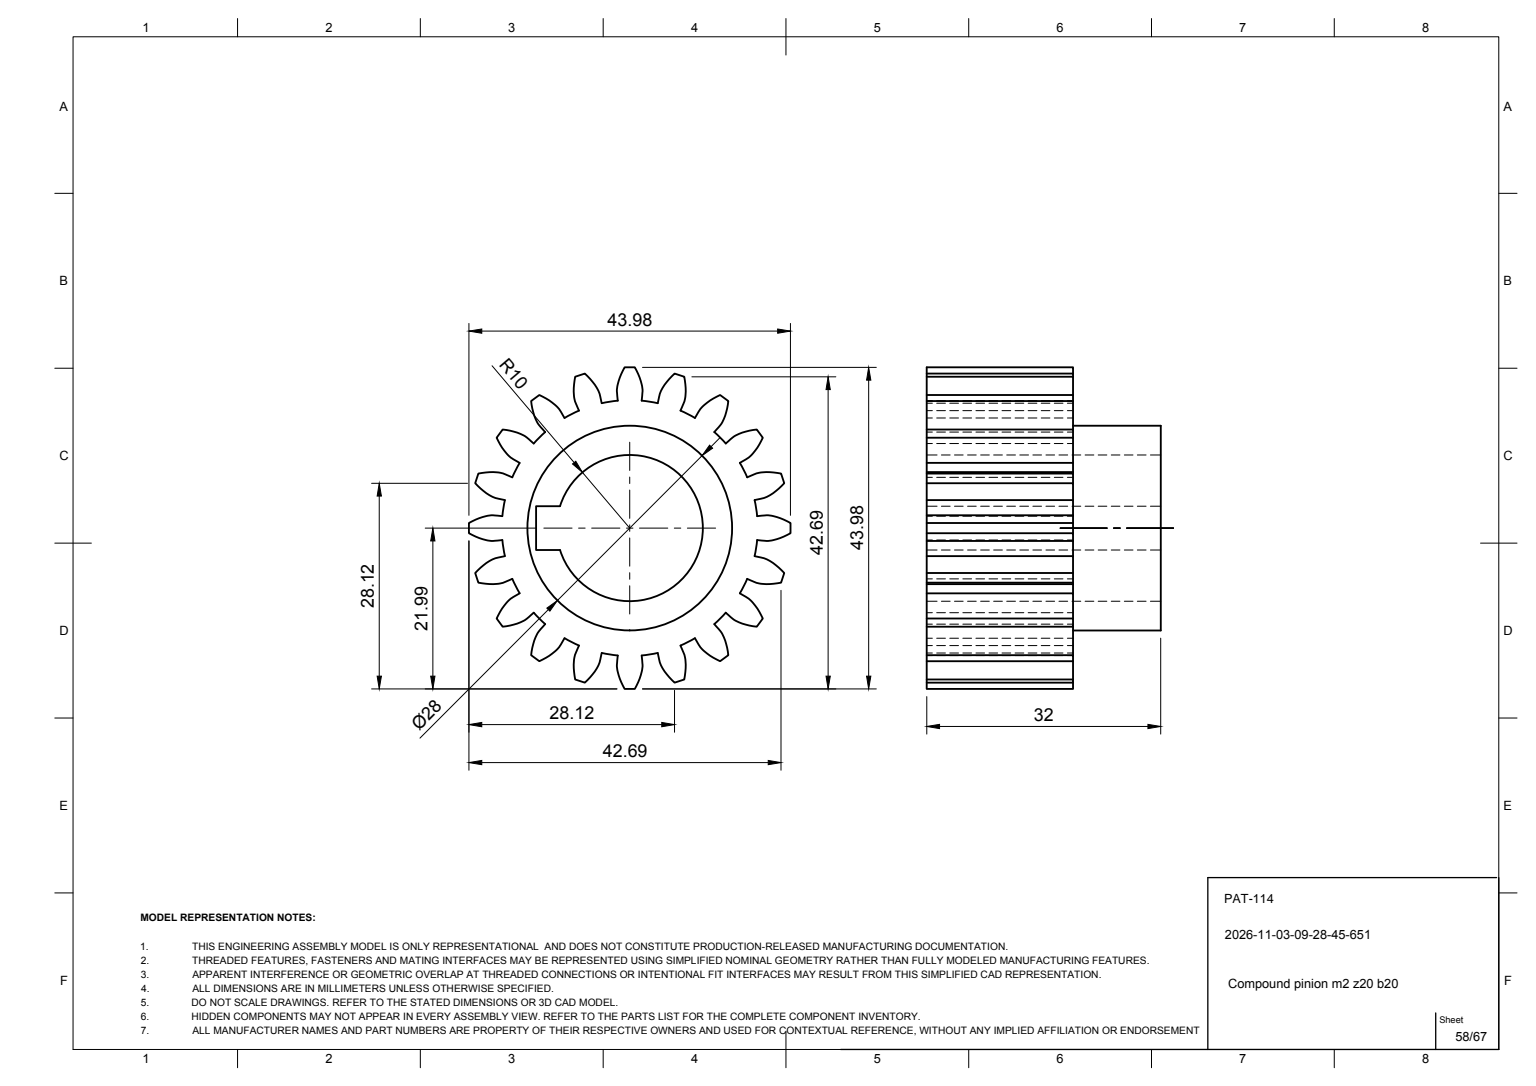
ISO-10303-21;
HEADER;
/* Generated by software containing ST-Developer
 * from STEP Tools, Inc. (www.steptools.com) 
 */

FILE_DESCRIPTION(
/* description */ ('Two-stage gear reducer in split housing'),
/* implementation_level */ '2;1');

FILE_NAME(
/* name */ 'Compound pinion m2 z20 b20.step',
/* time_stamp */ '2026-10-28T03:22:31-07:00',
/* author */ (''),
/* organization */ (''),
/* preprocessor_version */ 'ST-DEVELOPER v20.2',
/* originating_system */ 'Autodesk Translation Framework v15.17.0.0',
/* authorisation */ '');

FILE_SCHEMA (('AUTOMOTIVE_DESIGN { 1 0 10303 214 3 1 1 }'));
ENDSEC;

DATA;
#10=MECHANICAL_DESIGN_GEOMETRIC_PRESENTATION_REPRESENTATION('',(#1294),#73366);
#51=(
BOUNDED_SURFACE()
B_SPLINE_SURFACE(5,1,((#40614,#40615),(#40616,#40617),(#40618,#40619),(#40620,
#40621),(#40622,#40623),(#40624,#40625),(#40626,#40627),(#40628,#40629),
(#40630,#40631),(#40632,#40633),(#40634,#40635),(#40636,#40637),(#40638,
#40639),(#40640,#40641),(#40642,#40643),(#40644,#40645),(#40646,#40647),
(#40648,#40649),(#40650,#40651),(#40652,#40653),(#40654,#40655),(#40656,
#40657),(#40658,#40659),(#40660,#40661),(#40662,#40663),(#40664,#40665),
(#40666,#40667),(#40668,#40669),(#40670,#40671),(#40672,#40673),(#40674,
#40675),(#40676,#40677),(#40678,#40679),(#40680,#40681),(#40682,#40683),
(#40684,#40685),(#40686,#40687),(#40688,#40689),(#40690,#40691),(#40692,
#40693),(#40694,#40695),(#40696,#40697),(#40698,#40699),(#40700,#40701),
(#40702,#40703),(#40704,#40705),(#40706,#40707),(#40708,#40709),(#40710,
#40711),(#40712,#40713),(#40714,#40715),(#40716,#40717),(#40718,#40719),
(#40720,#40721),(#40722,#40723),(#40724,#40725),(#40726,#40727),(#40728,
#40729),(#40730,#40731),(#40732,#40733),(#40734,#40735),(#40736,#40737),
(#40738,#40739),(#40740,#40741),(#40742,#40743),(#40744,#40745),(#40746,
#40747),(#40748,#40749),(#40750,#40751),(#40752,#40753)),.UNSPECIFIED.,
 .F.,.F.,.F.)
B_SPLINE_SURFACE_WITH_KNOTS((6,1,1,1,1,1,1,1,1,1,1,1,1,1,1,1,1,1,1,1,1,
1,1,1,1,1,1,1,1,1,1,1,1,1,1,1,1,1,1,1,1,1,1,1,1,1,1,1,1,1,1,1,1,1,1,1,1,
1,1,1,1,1,1,1,1,6),(2,2),(-1.,-0.984615384615383,-0.969230769230768,-0.953846153846152,
-0.938461538461537,-0.923076923076922,-0.907692307692306,-0.892307692307691,
-0.876923076923076,-0.86153846153846,-0.846153846153845,-0.83076923076923,
-0.815384615384614,-0.799999999999999,-0.784615384615384,-0.769230769230768,
-0.753846153846153,-0.738461538461538,-0.723076923076922,-0.707692307692307,
-0.692307692307692,-0.676923076923076,-0.661538461538461,-0.646153846153846,
-0.63076923076923,-0.615384615384615,-0.6,-0.584615384615384,-0.569230769230769,
-0.553846153846154,-0.538461538461538,-0.523076923076923,-0.507692307692308,
-0.492307692307692,-0.476923076923077,-0.461538461538462,-0.446153846153846,
-0.430769230769231,-0.415384615384615,-0.4,-0.384615384615385,-0.369230769230769,
-0.353846153846154,-0.338461538461538,-0.323076923076923,-0.307692307692308,
-0.292307692307692,-0.276923076923077,-0.261538461538462,-0.246153846153846,
-0.230769230769231,-0.215384615384615,-0.2,-0.184615384615385,-0.169230769230769,
-0.153846153846154,-0.138461538461538,-0.123076923076923,-0.107692307692308,
-0.0923076923076923,-0.0769230769230769,-0.0615384615384615,-0.0461538461538462,
-0.0307692307692308,-0.0153846153846154,0.),(-1.,1.),.UNSPECIFIED.)
GEOMETRIC_REPRESENTATION_ITEM()
RATIONAL_B_SPLINE_SURFACE(((1.,1.),(1.,1.),(1.,1.),(1.,1.),(1.,1.),(1.,
1.),(1.,1.),(1.,1.),(1.,1.),(1.,1.),(1.,1.),(1.,1.),(1.,1.),(1.,1.),(1.,
1.),(1.,1.),(1.,1.),(1.,1.),(1.,1.),(1.,1.),(1.,1.),(1.,1.),(1.,1.),(1.,
1.),(1.,1.),(1.,1.),(1.,1.),(1.,1.),(1.,1.),(1.,1.),(1.,1.),(1.,1.),(1.,
1.),(1.,1.),(1.,1.),(1.,1.),(1.,1.),(1.,1.),(1.,1.),(1.,1.),(1.,1.),(1.,
1.),(1.,1.),(1.,1.),(1.,1.),(1.,1.),(1.,1.),(1.,1.),(1.,1.),(1.,1.),(1.,
1.),(1.,1.),(1.,1.),(1.,1.),(1.,1.),(1.,1.),(1.,1.),(1.,1.),(1.,1.),(1.,
1.),(1.,1.),(1.,1.),(1.,1.),(1.,1.),(1.,1.),(1.,1.),(1.,1.),(1.,1.),(1.,
1.),(1.,1.)))
REPRESENTATION_ITEM('')
SURFACE()
);
#52=(
BOUNDED_SURFACE()
B_SPLINE_SURFACE(5,1,((#40832,#40833),(#40834,#40835),(#40836,#40837),(#40838,
#40839),(#40840,#40841),(#40842,#40843),(#40844,#40845),(#40846,#40847),
(#40848,#40849),(#40850,#40851),(#40852,#40853),(#40854,#40855),(#40856,
#40857),(#40858,#40859),(#40860,#40861),(#40862,#40863),(#40864,#40865),
(#40866,#40867),(#40868,#40869),(#40870,#40871),(#40872,#40873),(#40874,
#40875),(#40876,#40877),(#40878,#40879),(#40880,#40881),(#40882,#40883),
(#40884,#40885),(#40886,#40887),(#40888,#40889),(#40890,#40891),(#40892,
#40893),(#40894,#40895),(#40896,#40897),(#40898,#40899),(#40900,#40901),
(#40902,#40903),(#40904,#40905),(#40906,#40907),(#40908,#40909),(#40910,
#40911),(#40912,#40913),(#40914,#40915),(#40916,#40917),(#40918,#40919),
(#40920,#40921),(#40922,#40923),(#40924,#40925),(#40926,#40927),(#40928,
#40929),(#40930,#40931),(#40932,#40933),(#40934,#40935),(#40936,#40937),
(#40938,#40939),(#40940,#40941),(#40942,#40943),(#40944,#40945),(#40946,
#40947),(#40948,#40949),(#40950,#40951),(#40952,#40953),(#40954,#40955),
(#40956,#40957),(#40958,#40959),(#40960,#40961),(#40962,#40963),(#40964,
#40965),(#40966,#40967),(#40968,#40969),(#40970,#40971)),.UNSPECIFIED.,
 .F.,.F.,.F.)
B_SPLINE_SURFACE_WITH_KNOTS((6,1,1,1,1,1,1,1,1,1,1,1,1,1,1,1,1,1,1,1,1,
1,1,1,1,1,1,1,1,1,1,1,1,1,1,1,1,1,1,1,1,1,1,1,1,1,1,1,1,1,1,1,1,1,1,1,1,
1,1,1,1,1,1,1,1,6),(2,2),(-1.,-0.984615384615383,-0.969230769230768,-0.953846153846152,
-0.938461538461537,-0.923076923076922,-0.907692307692306,-0.892307692307691,
-0.876923076923076,-0.86153846153846,-0.846153846153845,-0.83076923076923,
-0.815384615384614,-0.799999999999999,-0.784615384615384,-0.769230769230768,
-0.753846153846153,-0.738461538461538,-0.723076923076922,-0.707692307692307,
-0.692307692307692,-0.676923076923076,-0.661538461538461,-0.646153846153846,
-0.63076923076923,-0.615384615384615,-0.6,-0.584615384615384,-0.569230769230769,
-0.553846153846154,-0.538461538461538,-0.523076923076923,-0.507692307692308,
-0.492307692307692,-0.476923076923077,-0.461538461538462,-0.446153846153846,
-0.430769230769231,-0.415384615384615,-0.4,-0.384615384615385,-0.369230769230769,
-0.353846153846154,-0.338461538461538,-0.323076923076923,-0.307692307692308,
-0.292307692307692,-0.276923076923077,-0.261538461538462,-0.246153846153846,
-0.230769230769231,-0.215384615384615,-0.2,-0.184615384615385,-0.169230769230769,
-0.153846153846154,-0.138461538461538,-0.123076923076923,-0.107692307692308,
-0.0923076923076923,-0.0769230769230769,-0.0615384615384615,-0.0461538461538462,
-0.0307692307692308,-0.0153846153846154,0.),(-1.,1.),.UNSPECIFIED.)
GEOMETRIC_REPRESENTATION_ITEM()
RATIONAL_B_SPLINE_SURFACE(((1.,1.),(1.,1.),(1.,1.),(1.,1.),(1.,1.),(1.,
1.),(1.,1.),(1.,1.),(1.,1.),(1.,1.),(1.,1.),(1.,1.),(1.,1.),(1.,1.),(1.,
1.),(1.,1.),(1.,1.),(1.,1.),(1.,1.),(1.,1.),(1.,1.),(1.,1.),(1.,1.),(1.,
1.),(1.,1.),(1.,1.),(1.,1.),(1.,1.),(1.,1.),(1.,1.),(1.,1.),(1.,1.),(1.,
1.),(1.,1.),(1.,1.),(1.,1.),(1.,1.),(1.,1.),(1.,1.),(1.,1.),(1.,1.),(1.,
1.),(1.,1.),(1.,1.),(1.,1.),(1.,1.),(1.,1.),(1.,1.),(1.,1.),(1.,1.),(1.,
1.),(1.,1.),(1.,1.),(1.,1.),(1.,1.),(1.,1.),(1.,1.),(1.,1.),(1.,1.),(1.,
1.),(1.,1.),(1.,1.),(1.,1.),(1.,1.),(1.,1.),(1.,1.),(1.,1.),(1.,1.),(1.,
1.),(1.,1.)))
REPRESENTATION_ITEM('')
SURFACE()
);
#53=(
BOUNDED_SURFACE()
B_SPLINE_SURFACE(5,1,((#41048,#41049),(#41050,#41051),(#41052,#41053),(#41054,
#41055),(#41056,#41057),(#41058,#41059),(#41060,#41061),(#41062,#41063),
(#41064,#41065),(#41066,#41067),(#41068,#41069),(#41070,#41071),(#41072,
#41073),(#41074,#41075),(#41076,#41077),(#41078,#41079),(#41080,#41081),
(#41082,#41083),(#41084,#41085),(#41086,#41087),(#41088,#41089),(#41090,
#41091),(#41092,#41093),(#41094,#41095),(#41096,#41097),(#41098,#41099),
(#41100,#41101),(#41102,#41103),(#41104,#41105),(#41106,#41107),(#41108,
#41109),(#41110,#41111),(#41112,#41113),(#41114,#41115),(#41116,#41117),
(#41118,#41119),(#41120,#41121),(#41122,#41123),(#41124,#41125),(#41126,
#41127),(#41128,#41129),(#41130,#41131),(#41132,#41133),(#41134,#41135),
(#41136,#41137),(#41138,#41139),(#41140,#41141),(#41142,#41143),(#41144,
#41145),(#41146,#41147),(#41148,#41149),(#41150,#41151),(#41152,#41153),
(#41154,#41155),(#41156,#41157),(#41158,#41159),(#41160,#41161),(#41162,
#41163),(#41164,#41165),(#41166,#41167),(#41168,#41169),(#41170,#41171),
(#41172,#41173),(#41174,#41175),(#41176,#41177),(#41178,#41179),(#41180,
#41181),(#41182,#41183),(#41184,#41185),(#41186,#41187)),.UNSPECIFIED.,
 .F.,.F.,.F.)
B_SPLINE_SURFACE_WITH_KNOTS((6,1,1,1,1,1,1,1,1,1,1,1,1,1,1,1,1,1,1,1,1,
1,1,1,1,1,1,1,1,1,1,1,1,1,1,1,1,1,1,1,1,1,1,1,1,1,1,1,1,1,1,1,1,1,1,1,1,
1,1,1,1,1,1,1,1,6),(2,2),(-1.,-0.984615384615383,-0.969230769230768,-0.953846153846152,
-0.938461538461537,-0.923076923076922,-0.907692307692306,-0.892307692307691,
-0.876923076923076,-0.86153846153846,-0.846153846153845,-0.83076923076923,
-0.815384615384614,-0.799999999999999,-0.784615384615384,-0.769230769230768,
-0.753846153846153,-0.738461538461538,-0.723076923076922,-0.707692307692307,
-0.692307692307692,-0.676923076923076,-0.661538461538461,-0.646153846153846,
-0.63076923076923,-0.615384615384615,-0.6,-0.584615384615384,-0.569230769230769,
-0.553846153846154,-0.538461538461538,-0.523076923076923,-0.507692307692308,
-0.492307692307692,-0.476923076923077,-0.461538461538462,-0.446153846153846,
-0.430769230769231,-0.415384615384615,-0.4,-0.384615384615385,-0.369230769230769,
-0.353846153846154,-0.338461538461538,-0.323076923076923,-0.307692307692308,
-0.292307692307692,-0.276923076923077,-0.261538461538462,-0.246153846153846,
-0.230769230769231,-0.215384615384615,-0.2,-0.184615384615385,-0.169230769230769,
-0.153846153846154,-0.138461538461538,-0.123076923076923,-0.107692307692308,
-0.0923076923076923,-0.0769230769230769,-0.0615384615384615,-0.0461538461538462,
-0.0307692307692308,-0.0153846153846154,0.),(-1.,1.),.UNSPECIFIED.)
GEOMETRIC_REPRESENTATION_ITEM()
RATIONAL_B_SPLINE_SURFACE(((1.,1.),(1.,1.),(1.,1.),(1.,1.),(1.,1.),(1.,
1.),(1.,1.),(1.,1.),(1.,1.),(1.,1.),(1.,1.),(1.,1.),(1.,1.),(1.,1.),(1.,
1.),(1.,1.),(1.,1.),(1.,1.),(1.,1.),(1.,1.),(1.,1.),(1.,1.),(1.,1.),(1.,
1.),(1.,1.),(1.,1.),(1.,1.),(1.,1.),(1.,1.),(1.,1.),(1.,1.),(1.,1.),(1.,
1.),(1.,1.),(1.,1.),(1.,1.),(1.,1.),(1.,1.),(1.,1.),(1.,1.),(1.,1.),(1.,
1.),(1.,1.),(1.,1.),(1.,1.),(1.,1.),(1.,1.),(1.,1.),(1.,1.),(1.,1.),(1.,
1.),(1.,1.),(1.,1.),(1.,1.),(1.,1.),(1.,1.),(1.,1.),(1.,1.),(1.,1.),(1.,
1.),(1.,1.),(1.,1.),(1.,1.),(1.,1.),(1.,1.),(1.,1.),(1.,1.),(1.,1.),(1.,
1.),(1.,1.)))
REPRESENTATION_ITEM('')
SURFACE()
);
#54=(
BOUNDED_SURFACE()
B_SPLINE_SURFACE(5,1,((#41264,#41265),(#41266,#41267),(#41268,#41269),(#41270,
#41271),(#41272,#41273),(#41274,#41275),(#41276,#41277),(#41278,#41279),
(#41280,#41281),(#41282,#41283),(#41284,#41285),(#41286,#41287),(#41288,
#41289),(#41290,#41291),(#41292,#41293),(#41294,#41295),(#41296,#41297),
(#41298,#41299),(#41300,#41301),(#41302,#41303),(#41304,#41305),(#41306,
#41307),(#41308,#41309),(#41310,#41311),(#41312,#41313),(#41314,#41315),
(#41316,#41317),(#41318,#41319),(#41320,#41321),(#41322,#41323),(#41324,
#41325),(#41326,#41327),(#41328,#41329),(#41330,#41331),(#41332,#41333),
(#41334,#41335),(#41336,#41337),(#41338,#41339),(#41340,#41341),(#41342,
#41343),(#41344,#41345),(#41346,#41347),(#41348,#41349),(#41350,#41351),
(#41352,#41353),(#41354,#41355),(#41356,#41357),(#41358,#41359),(#41360,
#41361),(#41362,#41363),(#41364,#41365),(#41366,#41367),(#41368,#41369),
(#41370,#41371),(#41372,#41373),(#41374,#41375),(#41376,#41377),(#41378,
#41379),(#41380,#41381),(#41382,#41383),(#41384,#41385),(#41386,#41387),
(#41388,#41389),(#41390,#41391),(#41392,#41393),(#41394,#41395),(#41396,
#41397),(#41398,#41399),(#41400,#41401),(#41402,#41403)),.UNSPECIFIED.,
 .F.,.F.,.F.)
B_SPLINE_SURFACE_WITH_KNOTS((6,1,1,1,1,1,1,1,1,1,1,1,1,1,1,1,1,1,1,1,1,
1,1,1,1,1,1,1,1,1,1,1,1,1,1,1,1,1,1,1,1,1,1,1,1,1,1,1,1,1,1,1,1,1,1,1,1,
1,1,1,1,1,1,1,1,6),(2,2),(-1.,-0.984615384615383,-0.969230769230768,-0.953846153846152,
-0.938461538461537,-0.923076923076922,-0.907692307692306,-0.892307692307691,
-0.876923076923076,-0.86153846153846,-0.846153846153845,-0.83076923076923,
-0.815384615384614,-0.799999999999999,-0.784615384615384,-0.769230769230768,
-0.753846153846153,-0.738461538461538,-0.723076923076922,-0.707692307692307,
-0.692307692307692,-0.676923076923076,-0.661538461538461,-0.646153846153846,
-0.63076923076923,-0.615384615384615,-0.6,-0.584615384615384,-0.569230769230769,
-0.553846153846154,-0.538461538461538,-0.523076923076923,-0.507692307692308,
-0.492307692307692,-0.476923076923077,-0.461538461538462,-0.446153846153846,
-0.430769230769231,-0.415384615384615,-0.4,-0.384615384615385,-0.369230769230769,
-0.353846153846154,-0.338461538461538,-0.323076923076923,-0.307692307692308,
-0.292307692307692,-0.276923076923077,-0.261538461538462,-0.246153846153846,
-0.230769230769231,-0.215384615384615,-0.2,-0.184615384615385,-0.169230769230769,
-0.153846153846154,-0.138461538461538,-0.123076923076923,-0.107692307692308,
-0.0923076923076923,-0.0769230769230769,-0.0615384615384615,-0.0461538461538462,
-0.0307692307692308,-0.0153846153846154,0.),(-1.,1.),.UNSPECIFIED.)
GEOMETRIC_REPRESENTATION_ITEM()
RATIONAL_B_SPLINE_SURFACE(((1.,1.),(1.,1.),(1.,1.),(1.,1.),(1.,1.),(1.,
1.),(1.,1.),(1.,1.),(1.,1.),(1.,1.),(1.,1.),(1.,1.),(1.,1.),(1.,1.),(1.,
1.),(1.,1.),(1.,1.),(1.,1.),(1.,1.),(1.,1.),(1.,1.),(1.,1.),(1.,1.),(1.,
1.),(1.,1.),(1.,1.),(1.,1.),(1.,1.),(1.,1.),(1.,1.),(1.,1.),(1.,1.),(1.,
1.),(1.,1.),(1.,1.),(1.,1.),(1.,1.),(1.,1.),(1.,1.),(1.,1.),(1.,1.),(1.,
1.),(1.,1.),(1.,1.),(1.,1.),(1.,1.),(1.,1.),(1.,1.),(1.,1.),(1.,1.),(1.,
1.),(1.,1.),(1.,1.),(1.,1.),(1.,1.),(1.,1.),(1.,1.),(1.,1.),(1.,1.),(1.,
1.),(1.,1.),(1.,1.),(1.,1.),(1.,1.),(1.,1.),(1.,1.),(1.,1.),(1.,1.),(1.,
1.),(1.,1.)))
REPRESENTATION_ITEM('')
SURFACE()
);
#55=(
BOUNDED_SURFACE()
B_SPLINE_SURFACE(5,1,((#41480,#41481),(#41482,#41483),(#41484,#41485),(#41486,
#41487),(#41488,#41489),(#41490,#41491),(#41492,#41493),(#41494,#41495),
(#41496,#41497),(#41498,#41499),(#41500,#41501),(#41502,#41503),(#41504,
#41505),(#41506,#41507),(#41508,#41509),(#41510,#41511),(#41512,#41513),
(#41514,#41515),(#41516,#41517),(#41518,#41519),(#41520,#41521),(#41522,
#41523),(#41524,#41525),(#41526,#41527),(#41528,#41529),(#41530,#41531),
(#41532,#41533),(#41534,#41535),(#41536,#41537),(#41538,#41539),(#41540,
#41541),(#41542,#41543),(#41544,#41545),(#41546,#41547),(#41548,#41549),
(#41550,#41551),(#41552,#41553),(#41554,#41555),(#41556,#41557),(#41558,
#41559),(#41560,#41561),(#41562,#41563),(#41564,#41565),(#41566,#41567),
(#41568,#41569),(#41570,#41571),(#41572,#41573),(#41574,#41575),(#41576,
#41577),(#41578,#41579),(#41580,#41581),(#41582,#41583),(#41584,#41585),
(#41586,#41587),(#41588,#41589),(#41590,#41591),(#41592,#41593),(#41594,
#41595),(#41596,#41597),(#41598,#41599),(#41600,#41601),(#41602,#41603),
(#41604,#41605),(#41606,#41607),(#41608,#41609),(#41610,#41611),(#41612,
#41613),(#41614,#41615),(#41616,#41617),(#41618,#41619)),.UNSPECIFIED.,
 .F.,.F.,.F.)
B_SPLINE_SURFACE_WITH_KNOTS((6,1,1,1,1,1,1,1,1,1,1,1,1,1,1,1,1,1,1,1,1,
1,1,1,1,1,1,1,1,1,1,1,1,1,1,1,1,1,1,1,1,1,1,1,1,1,1,1,1,1,1,1,1,1,1,1,1,
1,1,1,1,1,1,1,1,6),(2,2),(-1.,-0.984615384615383,-0.969230769230768,-0.953846153846152,
-0.938461538461537,-0.923076923076922,-0.907692307692306,-0.892307692307691,
-0.876923076923076,-0.86153846153846,-0.846153846153845,-0.83076923076923,
-0.815384615384614,-0.799999999999999,-0.784615384615384,-0.769230769230768,
-0.753846153846153,-0.738461538461538,-0.723076923076922,-0.707692307692307,
-0.692307692307692,-0.676923076923076,-0.661538461538461,-0.646153846153846,
-0.63076923076923,-0.615384615384615,-0.6,-0.584615384615384,-0.569230769230769,
-0.553846153846154,-0.538461538461538,-0.523076923076923,-0.507692307692308,
-0.492307692307692,-0.476923076923077,-0.461538461538462,-0.446153846153846,
-0.430769230769231,-0.415384615384615,-0.4,-0.384615384615385,-0.369230769230769,
-0.353846153846154,-0.338461538461538,-0.323076923076923,-0.307692307692308,
-0.292307692307692,-0.276923076923077,-0.261538461538462,-0.246153846153846,
-0.230769230769231,-0.215384615384615,-0.2,-0.184615384615385,-0.169230769230769,
-0.153846153846154,-0.138461538461538,-0.123076923076923,-0.107692307692308,
-0.0923076923076923,-0.0769230769230769,-0.0615384615384615,-0.0461538461538462,
-0.0307692307692308,-0.0153846153846154,0.),(-1.,1.),.UNSPECIFIED.)
GEOMETRIC_REPRESENTATION_ITEM()
RATIONAL_B_SPLINE_SURFACE(((1.,1.),(1.,1.),(1.,1.),(1.,1.),(1.,1.),(1.,
1.),(1.,1.),(1.,1.),(1.,1.),(1.,1.),(1.,1.),(1.,1.),(1.,1.),(1.,1.),(1.,
1.),(1.,1.),(1.,1.),(1.,1.),(1.,1.),(1.,1.),(1.,1.),(1.,1.),(1.,1.),(1.,
1.),(1.,1.),(1.,1.),(1.,1.),(1.,1.),(1.,1.),(1.,1.),(1.,1.),(1.,1.),(1.,
1.),(1.,1.),(1.,1.),(1.,1.),(1.,1.),(1.,1.),(1.,1.),(1.,1.),(1.,1.),(1.,
1.),(1.,1.),(1.,1.),(1.,1.),(1.,1.),(1.,1.),(1.,1.),(1.,1.),(1.,1.),(1.,
1.),(1.,1.),(1.,1.),(1.,1.),(1.,1.),(1.,1.),(1.,1.),(1.,1.),(1.,1.),(1.,
1.),(1.,1.),(1.,1.),(1.,1.),(1.,1.),(1.,1.),(1.,1.),(1.,1.),(1.,1.),(1.,
1.),(1.,1.)))
REPRESENTATION_ITEM('')
SURFACE()
);
#56=(
BOUNDED_SURFACE()
B_SPLINE_SURFACE(5,1,((#41696,#41697),(#41698,#41699),(#41700,#41701),(#41702,
#41703),(#41704,#41705),(#41706,#41707),(#41708,#41709),(#41710,#41711),
(#41712,#41713),(#41714,#41715),(#41716,#41717),(#41718,#41719),(#41720,
#41721),(#41722,#41723),(#41724,#41725),(#41726,#41727),(#41728,#41729),
(#41730,#41731),(#41732,#41733),(#41734,#41735),(#41736,#41737),(#41738,
#41739),(#41740,#41741),(#41742,#41743),(#41744,#41745),(#41746,#41747),
(#41748,#41749),(#41750,#41751),(#41752,#41753),(#41754,#41755),(#41756,
#41757),(#41758,#41759),(#41760,#41761),(#41762,#41763),(#41764,#41765),
(#41766,#41767),(#41768,#41769),(#41770,#41771),(#41772,#41773),(#41774,
#41775),(#41776,#41777),(#41778,#41779),(#41780,#41781),(#41782,#41783),
(#41784,#41785),(#41786,#41787),(#41788,#41789),(#41790,#41791),(#41792,
#41793),(#41794,#41795),(#41796,#41797),(#41798,#41799),(#41800,#41801),
(#41802,#41803),(#41804,#41805),(#41806,#41807),(#41808,#41809),(#41810,
#41811),(#41812,#41813),(#41814,#41815),(#41816,#41817),(#41818,#41819),
(#41820,#41821),(#41822,#41823),(#41824,#41825),(#41826,#41827),(#41828,
#41829),(#41830,#41831),(#41832,#41833),(#41834,#41835)),.UNSPECIFIED.,
 .F.,.F.,.F.)
B_SPLINE_SURFACE_WITH_KNOTS((6,1,1,1,1,1,1,1,1,1,1,1,1,1,1,1,1,1,1,1,1,
1,1,1,1,1,1,1,1,1,1,1,1,1,1,1,1,1,1,1,1,1,1,1,1,1,1,1,1,1,1,1,1,1,1,1,1,
1,1,1,1,1,1,1,1,6),(2,2),(-1.,-0.984615384615383,-0.969230769230768,-0.953846153846152,
-0.938461538461537,-0.923076923076922,-0.907692307692306,-0.892307692307691,
-0.876923076923076,-0.86153846153846,-0.846153846153845,-0.83076923076923,
-0.815384615384614,-0.799999999999999,-0.784615384615384,-0.769230769230768,
-0.753846153846153,-0.738461538461538,-0.723076923076922,-0.707692307692307,
-0.692307692307692,-0.676923076923076,-0.661538461538461,-0.646153846153846,
-0.63076923076923,-0.615384615384615,-0.6,-0.584615384615384,-0.569230769230769,
-0.553846153846154,-0.538461538461538,-0.523076923076923,-0.507692307692308,
-0.492307692307692,-0.476923076923077,-0.461538461538462,-0.446153846153846,
-0.430769230769231,-0.415384615384615,-0.4,-0.384615384615385,-0.369230769230769,
-0.353846153846154,-0.338461538461538,-0.323076923076923,-0.307692307692308,
-0.292307692307692,-0.276923076923077,-0.261538461538462,-0.246153846153846,
-0.230769230769231,-0.215384615384615,-0.2,-0.184615384615385,-0.169230769230769,
-0.153846153846154,-0.138461538461538,-0.123076923076923,-0.107692307692308,
-0.0923076923076923,-0.0769230769230769,-0.0615384615384615,-0.0461538461538462,
-0.0307692307692308,-0.0153846153846154,0.),(-1.,1.),.UNSPECIFIED.)
GEOMETRIC_REPRESENTATION_ITEM()
RATIONAL_B_SPLINE_SURFACE(((1.,1.),(1.,1.),(1.,1.),(1.,1.),(1.,1.),(1.,
1.),(1.,1.),(1.,1.),(1.,1.),(1.,1.),(1.,1.),(1.,1.),(1.,1.),(1.,1.),(1.,
1.),(1.,1.),(1.,1.),(1.,1.),(1.,1.),(1.,1.),(1.,1.),(1.,1.),(1.,1.),(1.,
1.),(1.,1.),(1.,1.),(1.,1.),(1.,1.),(1.,1.),(1.,1.),(1.,1.),(1.,1.),(1.,
1.),(1.,1.),(1.,1.),(1.,1.),(1.,1.),(1.,1.),(1.,1.),(1.,1.),(1.,1.),(1.,
1.),(1.,1.),(1.,1.),(1.,1.),(1.,1.),(1.,1.),(1.,1.),(1.,1.),(1.,1.),(1.,
1.),(1.,1.),(1.,1.),(1.,1.),(1.,1.),(1.,1.),(1.,1.),(1.,1.),(1.,1.),(1.,
1.),(1.,1.),(1.,1.),(1.,1.),(1.,1.),(1.,1.),(1.,1.),(1.,1.),(1.,1.),(1.,
1.),(1.,1.)))
REPRESENTATION_ITEM('')
SURFACE()
);
#57=(
BOUNDED_SURFACE()
B_SPLINE_SURFACE(5,1,((#41912,#41913),(#41914,#41915),(#41916,#41917),(#41918,
#41919),(#41920,#41921),(#41922,#41923),(#41924,#41925),(#41926,#41927),
(#41928,#41929),(#41930,#41931),(#41932,#41933),(#41934,#41935),(#41936,
#41937),(#41938,#41939),(#41940,#41941),(#41942,#41943),(#41944,#41945),
(#41946,#41947),(#41948,#41949),(#41950,#41951),(#41952,#41953),(#41954,
#41955),(#41956,#41957),(#41958,#41959),(#41960,#41961),(#41962,#41963),
(#41964,#41965),(#41966,#41967),(#41968,#41969),(#41970,#41971),(#41972,
#41973),(#41974,#41975),(#41976,#41977),(#41978,#41979),(#41980,#41981),
(#41982,#41983),(#41984,#41985),(#41986,#41987),(#41988,#41989),(#41990,
#41991),(#41992,#41993),(#41994,#41995),(#41996,#41997),(#41998,#41999),
(#42000,#42001),(#42002,#42003),(#42004,#42005),(#42006,#42007),(#42008,
#42009),(#42010,#42011),(#42012,#42013),(#42014,#42015),(#42016,#42017),
(#42018,#42019),(#42020,#42021),(#42022,#42023),(#42024,#42025),(#42026,
#42027),(#42028,#42029),(#42030,#42031),(#42032,#42033),(#42034,#42035),
(#42036,#42037),(#42038,#42039),(#42040,#42041),(#42042,#42043),(#42044,
#42045),(#42046,#42047),(#42048,#42049),(#42050,#42051)),.UNSPECIFIED.,
 .F.,.F.,.F.)
B_SPLINE_SURFACE_WITH_KNOTS((6,1,1,1,1,1,1,1,1,1,1,1,1,1,1,1,1,1,1,1,1,
1,1,1,1,1,1,1,1,1,1,1,1,1,1,1,1,1,1,1,1,1,1,1,1,1,1,1,1,1,1,1,1,1,1,1,1,
1,1,1,1,1,1,1,1,6),(2,2),(-1.,-0.984615384615383,-0.969230769230768,-0.953846153846152,
-0.938461538461537,-0.923076923076922,-0.907692307692306,-0.892307692307691,
-0.876923076923076,-0.86153846153846,-0.846153846153845,-0.83076923076923,
-0.815384615384614,-0.799999999999999,-0.784615384615384,-0.769230769230768,
-0.753846153846153,-0.738461538461538,-0.723076923076922,-0.707692307692307,
-0.692307692307692,-0.676923076923076,-0.661538461538461,-0.646153846153846,
-0.63076923076923,-0.615384615384615,-0.6,-0.584615384615384,-0.569230769230769,
-0.553846153846154,-0.538461538461538,-0.523076923076923,-0.507692307692308,
-0.492307692307692,-0.476923076923077,-0.461538461538462,-0.446153846153846,
-0.430769230769231,-0.415384615384615,-0.4,-0.384615384615385,-0.369230769230769,
-0.353846153846154,-0.338461538461538,-0.323076923076923,-0.307692307692308,
-0.292307692307692,-0.276923076923077,-0.261538461538462,-0.246153846153846,
-0.230769230769231,-0.215384615384615,-0.2,-0.184615384615385,-0.169230769230769,
-0.153846153846154,-0.138461538461538,-0.123076923076923,-0.107692307692308,
-0.0923076923076923,-0.0769230769230769,-0.0615384615384615,-0.0461538461538462,
-0.0307692307692308,-0.0153846153846154,0.),(-1.,1.),.UNSPECIFIED.)
GEOMETRIC_REPRESENTATION_ITEM()
RATIONAL_B_SPLINE_SURFACE(((1.,1.),(1.,1.),(1.,1.),(1.,1.),(1.,1.),(1.,
1.),(1.,1.),(1.,1.),(1.,1.),(1.,1.),(1.,1.),(1.,1.),(1.,1.),(1.,1.),(1.,
1.),(1.,1.),(1.,1.),(1.,1.),(1.,1.),(1.,1.),(1.,1.),(1.,1.),(1.,1.),(1.,
1.),(1.,1.),(1.,1.),(1.,1.),(1.,1.),(1.,1.),(1.,1.),(1.,1.),(1.,1.),(1.,
1.),(1.,1.),(1.,1.),(1.,1.),(1.,1.),(1.,1.),(1.,1.),(1.,1.),(1.,1.),(1.,
1.),(1.,1.),(1.,1.),(1.,1.),(1.,1.),(1.,1.),(1.,1.),(1.,1.),(1.,1.),(1.,
1.),(1.,1.),(1.,1.),(1.,1.),(1.,1.),(1.,1.),(1.,1.),(1.,1.),(1.,1.),(1.,
1.),(1.,1.),(1.,1.),(1.,1.),(1.,1.),(1.,1.),(1.,1.),(1.,1.),(1.,1.),(1.,
1.),(1.,1.)))
REPRESENTATION_ITEM('')
SURFACE()
);
#58=(
BOUNDED_SURFACE()
B_SPLINE_SURFACE(5,1,((#42128,#42129),(#42130,#42131),(#42132,#42133),(#42134,
#42135),(#42136,#42137),(#42138,#42139),(#42140,#42141),(#42142,#42143),
(#42144,#42145),(#42146,#42147),(#42148,#42149),(#42150,#42151),(#42152,
#42153),(#42154,#42155),(#42156,#42157),(#42158,#42159),(#42160,#42161),
(#42162,#42163),(#42164,#42165),(#42166,#42167),(#42168,#42169),(#42170,
#42171),(#42172,#42173),(#42174,#42175),(#42176,#42177),(#42178,#42179),
(#42180,#42181),(#42182,#42183),(#42184,#42185),(#42186,#42187),(#42188,
#42189),(#42190,#42191),(#42192,#42193),(#42194,#42195),(#42196,#42197),
(#42198,#42199),(#42200,#42201),(#42202,#42203),(#42204,#42205),(#42206,
#42207),(#42208,#42209),(#42210,#42211),(#42212,#42213),(#42214,#42215),
(#42216,#42217),(#42218,#42219),(#42220,#42221),(#42222,#42223),(#42224,
#42225),(#42226,#42227),(#42228,#42229),(#42230,#42231),(#42232,#42233),
(#42234,#42235),(#42236,#42237),(#42238,#42239),(#42240,#42241),(#42242,
#42243),(#42244,#42245),(#42246,#42247),(#42248,#42249),(#42250,#42251),
(#42252,#42253),(#42254,#42255),(#42256,#42257),(#42258,#42259),(#42260,
#42261),(#42262,#42263),(#42264,#42265),(#42266,#42267)),.UNSPECIFIED.,
 .F.,.F.,.F.)
B_SPLINE_SURFACE_WITH_KNOTS((6,1,1,1,1,1,1,1,1,1,1,1,1,1,1,1,1,1,1,1,1,
1,1,1,1,1,1,1,1,1,1,1,1,1,1,1,1,1,1,1,1,1,1,1,1,1,1,1,1,1,1,1,1,1,1,1,1,
1,1,1,1,1,1,1,1,6),(2,2),(-1.,-0.984615384615383,-0.969230769230768,-0.953846153846152,
-0.938461538461537,-0.923076923076922,-0.907692307692306,-0.892307692307691,
-0.876923076923076,-0.86153846153846,-0.846153846153845,-0.83076923076923,
-0.815384615384614,-0.799999999999999,-0.784615384615384,-0.769230769230768,
-0.753846153846153,-0.738461538461538,-0.723076923076922,-0.707692307692307,
-0.692307692307692,-0.676923076923076,-0.661538461538461,-0.646153846153846,
-0.63076923076923,-0.615384615384615,-0.6,-0.584615384615384,-0.569230769230769,
-0.553846153846154,-0.538461538461538,-0.523076923076923,-0.507692307692308,
-0.492307692307692,-0.476923076923077,-0.461538461538462,-0.446153846153846,
-0.430769230769231,-0.415384615384615,-0.4,-0.384615384615385,-0.369230769230769,
-0.353846153846154,-0.338461538461538,-0.323076923076923,-0.307692307692308,
-0.292307692307692,-0.276923076923077,-0.261538461538462,-0.246153846153846,
-0.230769230769231,-0.215384615384615,-0.2,-0.184615384615385,-0.169230769230769,
-0.153846153846154,-0.138461538461538,-0.123076923076923,-0.107692307692308,
-0.0923076923076923,-0.0769230769230769,-0.0615384615384615,-0.0461538461538462,
-0.0307692307692308,-0.0153846153846154,0.),(-1.,1.),.UNSPECIFIED.)
GEOMETRIC_REPRESENTATION_ITEM()
RATIONAL_B_SPLINE_SURFACE(((1.,1.),(1.,1.),(1.,1.),(1.,1.),(1.,1.),(1.,
1.),(1.,1.),(1.,1.),(1.,1.),(1.,1.),(1.,1.),(1.,1.),(1.,1.),(1.,1.),(1.,
1.),(1.,1.),(1.,1.),(1.,1.),(1.,1.),(1.,1.),(1.,1.),(1.,1.),(1.,1.),(1.,
1.),(1.,1.),(1.,1.),(1.,1.),(1.,1.),(1.,1.),(1.,1.),(1.,1.),(1.,1.),(1.,
1.),(1.,1.),(1.,1.),(1.,1.),(1.,1.),(1.,1.),(1.,1.),(1.,1.),(1.,1.),(1.,
1.),(1.,1.),(1.,1.),(1.,1.),(1.,1.),(1.,1.),(1.,1.),(1.,1.),(1.,1.),(1.,
1.),(1.,1.),(1.,1.),(1.,1.),(1.,1.),(1.,1.),(1.,1.),(1.,1.),(1.,1.),(1.,
1.),(1.,1.),(1.,1.),(1.,1.),(1.,1.),(1.,1.),(1.,1.),(1.,1.),(1.,1.),(1.,
1.),(1.,1.)))
REPRESENTATION_ITEM('')
SURFACE()
);
#59=(
BOUNDED_SURFACE()
B_SPLINE_SURFACE(5,1,((#42344,#42345),(#42346,#42347),(#42348,#42349),(#42350,
#42351),(#42352,#42353),(#42354,#42355),(#42356,#42357),(#42358,#42359),
(#42360,#42361),(#42362,#42363),(#42364,#42365),(#42366,#42367),(#42368,
#42369),(#42370,#42371),(#42372,#42373),(#42374,#42375),(#42376,#42377),
(#42378,#42379),(#42380,#42381),(#42382,#42383),(#42384,#42385),(#42386,
#42387),(#42388,#42389),(#42390,#42391),(#42392,#42393),(#42394,#42395),
(#42396,#42397),(#42398,#42399),(#42400,#42401),(#42402,#42403),(#42404,
#42405),(#42406,#42407),(#42408,#42409),(#42410,#42411),(#42412,#42413),
(#42414,#42415),(#42416,#42417),(#42418,#42419),(#42420,#42421),(#42422,
#42423),(#42424,#42425),(#42426,#42427),(#42428,#42429),(#42430,#42431),
(#42432,#42433),(#42434,#42435),(#42436,#42437),(#42438,#42439),(#42440,
#42441),(#42442,#42443),(#42444,#42445),(#42446,#42447),(#42448,#42449),
(#42450,#42451),(#42452,#42453),(#42454,#42455),(#42456,#42457),(#42458,
#42459),(#42460,#42461),(#42462,#42463),(#42464,#42465),(#42466,#42467),
(#42468,#42469),(#42470,#42471),(#42472,#42473),(#42474,#42475),(#42476,
#42477),(#42478,#42479),(#42480,#42481),(#42482,#42483)),.UNSPECIFIED.,
 .F.,.F.,.F.)
B_SPLINE_SURFACE_WITH_KNOTS((6,1,1,1,1,1,1,1,1,1,1,1,1,1,1,1,1,1,1,1,1,
1,1,1,1,1,1,1,1,1,1,1,1,1,1,1,1,1,1,1,1,1,1,1,1,1,1,1,1,1,1,1,1,1,1,1,1,
1,1,1,1,1,1,1,1,6),(2,2),(-1.,-0.984615384615383,-0.969230769230768,-0.953846153846152,
-0.938461538461537,-0.923076923076922,-0.907692307692306,-0.892307692307691,
-0.876923076923076,-0.86153846153846,-0.846153846153845,-0.83076923076923,
-0.815384615384614,-0.799999999999999,-0.784615384615384,-0.769230769230768,
-0.753846153846153,-0.738461538461538,-0.723076923076922,-0.707692307692307,
-0.692307692307692,-0.676923076923076,-0.661538461538461,-0.646153846153846,
-0.63076923076923,-0.615384615384615,-0.6,-0.584615384615384,-0.569230769230769,
-0.553846153846154,-0.538461538461538,-0.523076923076923,-0.507692307692308,
-0.492307692307692,-0.476923076923077,-0.461538461538462,-0.446153846153846,
-0.430769230769231,-0.415384615384615,-0.4,-0.384615384615385,-0.369230769230769,
-0.353846153846154,-0.338461538461538,-0.323076923076923,-0.307692307692308,
-0.292307692307692,-0.276923076923077,-0.261538461538462,-0.246153846153846,
-0.230769230769231,-0.215384615384615,-0.2,-0.184615384615385,-0.169230769230769,
-0.153846153846154,-0.138461538461538,-0.123076923076923,-0.107692307692308,
-0.0923076923076923,-0.0769230769230769,-0.0615384615384615,-0.0461538461538462,
-0.0307692307692308,-0.0153846153846154,0.),(-1.,1.),.UNSPECIFIED.)
GEOMETRIC_REPRESENTATION_ITEM()
RATIONAL_B_SPLINE_SURFACE(((1.,1.),(1.,1.),(1.,1.),(1.,1.),(1.,1.),(1.,
1.),(1.,1.),(1.,1.),(1.,1.),(1.,1.),(1.,1.),(1.,1.),(1.,1.),(1.,1.),(1.,
1.),(1.,1.),(1.,1.),(1.,1.),(1.,1.),(1.,1.),(1.,1.),(1.,1.),(1.,1.),(1.,
1.),(1.,1.),(1.,1.),(1.,1.),(1.,1.),(1.,1.),(1.,1.),(1.,1.),(1.,1.),(1.,
1.),(1.,1.),(1.,1.),(1.,1.),(1.,1.),(1.,1.),(1.,1.),(1.,1.),(1.,1.),(1.,
1.),(1.,1.),(1.,1.),(1.,1.),(1.,1.),(1.,1.),(1.,1.),(1.,1.),(1.,1.),(1.,
1.),(1.,1.),(1.,1.),(1.,1.),(1.,1.),(1.,1.),(1.,1.),(1.,1.),(1.,1.),(1.,
1.),(1.,1.),(1.,1.),(1.,1.),(1.,1.),(1.,1.),(1.,1.),(1.,1.),(1.,1.),(1.,
1.),(1.,1.)))
REPRESENTATION_ITEM('')
SURFACE()
);
#60=(
BOUNDED_SURFACE()
B_SPLINE_SURFACE(5,1,((#42560,#42561),(#42562,#42563),(#42564,#42565),(#42566,
#42567),(#42568,#42569),(#42570,#42571),(#42572,#42573),(#42574,#42575),
(#42576,#42577),(#42578,#42579),(#42580,#42581),(#42582,#42583),(#42584,
#42585),(#42586,#42587),(#42588,#42589),(#42590,#42591),(#42592,#42593),
(#42594,#42595),(#42596,#42597),(#42598,#42599),(#42600,#42601),(#42602,
#42603),(#42604,#42605),(#42606,#42607),(#42608,#42609),(#42610,#42611),
(#42612,#42613),(#42614,#42615),(#42616,#42617),(#42618,#42619),(#42620,
#42621),(#42622,#42623),(#42624,#42625),(#42626,#42627),(#42628,#42629),
(#42630,#42631),(#42632,#42633),(#42634,#42635),(#42636,#42637),(#42638,
#42639),(#42640,#42641),(#42642,#42643),(#42644,#42645),(#42646,#42647),
(#42648,#42649),(#42650,#42651),(#42652,#42653),(#42654,#42655),(#42656,
#42657),(#42658,#42659),(#42660,#42661),(#42662,#42663),(#42664,#42665),
(#42666,#42667),(#42668,#42669),(#42670,#42671),(#42672,#42673),(#42674,
#42675),(#42676,#42677),(#42678,#42679),(#42680,#42681),(#42682,#42683),
(#42684,#42685),(#42686,#42687),(#42688,#42689),(#42690,#42691),(#42692,
#42693),(#42694,#42695),(#42696,#42697),(#42698,#42699)),.UNSPECIFIED.,
 .F.,.F.,.F.)
B_SPLINE_SURFACE_WITH_KNOTS((6,1,1,1,1,1,1,1,1,1,1,1,1,1,1,1,1,1,1,1,1,
1,1,1,1,1,1,1,1,1,1,1,1,1,1,1,1,1,1,1,1,1,1,1,1,1,1,1,1,1,1,1,1,1,1,1,1,
1,1,1,1,1,1,1,1,6),(2,2),(-1.,-0.984615384615383,-0.969230769230768,-0.953846153846152,
-0.938461538461537,-0.923076923076922,-0.907692307692306,-0.892307692307691,
-0.876923076923076,-0.86153846153846,-0.846153846153845,-0.83076923076923,
-0.815384615384614,-0.799999999999999,-0.784615384615384,-0.769230769230768,
-0.753846153846153,-0.738461538461538,-0.723076923076922,-0.707692307692307,
-0.692307692307692,-0.676923076923076,-0.661538461538461,-0.646153846153846,
-0.63076923076923,-0.615384615384615,-0.6,-0.584615384615384,-0.569230769230769,
-0.553846153846154,-0.538461538461538,-0.523076923076923,-0.507692307692308,
-0.492307692307692,-0.476923076923077,-0.461538461538462,-0.446153846153846,
-0.430769230769231,-0.415384615384615,-0.4,-0.384615384615385,-0.369230769230769,
-0.353846153846154,-0.338461538461538,-0.323076923076923,-0.307692307692308,
-0.292307692307692,-0.276923076923077,-0.261538461538462,-0.246153846153846,
-0.230769230769231,-0.215384615384615,-0.2,-0.184615384615385,-0.169230769230769,
-0.153846153846154,-0.138461538461538,-0.123076923076923,-0.107692307692308,
-0.0923076923076923,-0.0769230769230769,-0.0615384615384615,-0.0461538461538462,
-0.0307692307692308,-0.0153846153846154,0.),(-1.,1.),.UNSPECIFIED.)
GEOMETRIC_REPRESENTATION_ITEM()
RATIONAL_B_SPLINE_SURFACE(((1.,1.),(1.,1.),(1.,1.),(1.,1.),(1.,1.),(1.,
1.),(1.,1.),(1.,1.),(1.,1.),(1.,1.),(1.,1.),(1.,1.),(1.,1.),(1.,1.),(1.,
1.),(1.,1.),(1.,1.),(1.,1.),(1.,1.),(1.,1.),(1.,1.),(1.,1.),(1.,1.),(1.,
1.),(1.,1.),(1.,1.),(1.,1.),(1.,1.),(1.,1.),(1.,1.),(1.,1.),(1.,1.),(1.,
1.),(1.,1.),(1.,1.),(1.,1.),(1.,1.),(1.,1.),(1.,1.),(1.,1.),(1.,1.),(1.,
1.),(1.,1.),(1.,1.),(1.,1.),(1.,1.),(1.,1.),(1.,1.),(1.,1.),(1.,1.),(1.,
1.),(1.,1.),(1.,1.),(1.,1.),(1.,1.),(1.,1.),(1.,1.),(1.,1.),(1.,1.),(1.,
1.),(1.,1.),(1.,1.),(1.,1.),(1.,1.),(1.,1.),(1.,1.),(1.,1.),(1.,1.),(1.,
1.),(1.,1.)))
REPRESENTATION_ITEM('')
SURFACE()
);
#61=(
BOUNDED_SURFACE()
B_SPLINE_SURFACE(5,1,((#42776,#42777),(#42778,#42779),(#42780,#42781),(#42782,
#42783),(#42784,#42785),(#42786,#42787),(#42788,#42789),(#42790,#42791),
(#42792,#42793),(#42794,#42795),(#42796,#42797),(#42798,#42799),(#42800,
#42801),(#42802,#42803),(#42804,#42805),(#42806,#42807),(#42808,#42809),
(#42810,#42811),(#42812,#42813),(#42814,#42815),(#42816,#42817),(#42818,
#42819),(#42820,#42821),(#42822,#42823),(#42824,#42825),(#42826,#42827),
(#42828,#42829),(#42830,#42831),(#42832,#42833),(#42834,#42835),(#42836,
#42837),(#42838,#42839),(#42840,#42841),(#42842,#42843),(#42844,#42845),
(#42846,#42847),(#42848,#42849),(#42850,#42851),(#42852,#42853),(#42854,
#42855),(#42856,#42857),(#42858,#42859),(#42860,#42861),(#42862,#42863),
(#42864,#42865),(#42866,#42867),(#42868,#42869),(#42870,#42871),(#42872,
#42873),(#42874,#42875),(#42876,#42877),(#42878,#42879),(#42880,#42881),
(#42882,#42883),(#42884,#42885),(#42886,#42887),(#42888,#42889),(#42890,
#42891),(#42892,#42893),(#42894,#42895),(#42896,#42897),(#42898,#42899),
(#42900,#42901),(#42902,#42903),(#42904,#42905),(#42906,#42907),(#42908,
#42909),(#42910,#42911),(#42912,#42913),(#42914,#42915)),.UNSPECIFIED.,
 .F.,.F.,.F.)
B_SPLINE_SURFACE_WITH_KNOTS((6,1,1,1,1,1,1,1,1,1,1,1,1,1,1,1,1,1,1,1,1,
1,1,1,1,1,1,1,1,1,1,1,1,1,1,1,1,1,1,1,1,1,1,1,1,1,1,1,1,1,1,1,1,1,1,1,1,
1,1,1,1,1,1,1,1,6),(2,2),(-1.,-0.984615384615383,-0.969230769230768,-0.953846153846152,
-0.938461538461537,-0.923076923076922,-0.907692307692306,-0.892307692307691,
-0.876923076923076,-0.86153846153846,-0.846153846153845,-0.83076923076923,
-0.815384615384614,-0.799999999999999,-0.784615384615384,-0.769230769230768,
-0.753846153846153,-0.738461538461538,-0.723076923076922,-0.707692307692307,
-0.692307692307692,-0.676923076923076,-0.661538461538461,-0.646153846153846,
-0.63076923076923,-0.615384615384615,-0.6,-0.584615384615384,-0.569230769230769,
-0.553846153846154,-0.538461538461538,-0.523076923076923,-0.507692307692308,
-0.492307692307692,-0.476923076923077,-0.461538461538462,-0.446153846153846,
-0.430769230769231,-0.415384615384615,-0.4,-0.384615384615385,-0.369230769230769,
-0.353846153846154,-0.338461538461538,-0.323076923076923,-0.307692307692308,
-0.292307692307692,-0.276923076923077,-0.261538461538462,-0.246153846153846,
-0.230769230769231,-0.215384615384615,-0.2,-0.184615384615385,-0.169230769230769,
-0.153846153846154,-0.138461538461538,-0.123076923076923,-0.107692307692308,
-0.0923076923076923,-0.0769230769230769,-0.0615384615384615,-0.0461538461538462,
-0.0307692307692308,-0.0153846153846154,0.),(-1.,1.),.UNSPECIFIED.)
GEOMETRIC_REPRESENTATION_ITEM()
RATIONAL_B_SPLINE_SURFACE(((1.,1.),(1.,1.),(1.,1.),(1.,1.),(1.,1.),(1.,
1.),(1.,1.),(1.,1.),(1.,1.),(1.,1.),(1.,1.),(1.,1.),(1.,1.),(1.,1.),(1.,
1.),(1.,1.),(1.,1.),(1.,1.),(1.,1.),(1.,1.),(1.,1.),(1.,1.),(1.,1.),(1.,
1.),(1.,1.),(1.,1.),(1.,1.),(1.,1.),(1.,1.),(1.,1.),(1.,1.),(1.,1.),(1.,
1.),(1.,1.),(1.,1.),(1.,1.),(1.,1.),(1.,1.),(1.,1.),(1.,1.),(1.,1.),(1.,
1.),(1.,1.),(1.,1.),(1.,1.),(1.,1.),(1.,1.),(1.,1.),(1.,1.),(1.,1.),(1.,
1.),(1.,1.),(1.,1.),(1.,1.),(1.,1.),(1.,1.),(1.,1.),(1.,1.),(1.,1.),(1.,
1.),(1.,1.),(1.,1.),(1.,1.),(1.,1.),(1.,1.),(1.,1.),(1.,1.),(1.,1.),(1.,
1.),(1.,1.)))
REPRESENTATION_ITEM('')
SURFACE()
);
#62=(
BOUNDED_SURFACE()
B_SPLINE_SURFACE(5,1,((#42992,#42993),(#42994,#42995),(#42996,#42997),(#42998,
#42999),(#43000,#43001),(#43002,#43003),(#43004,#43005),(#43006,#43007),
(#43008,#43009),(#43010,#43011),(#43012,#43013),(#43014,#43015),(#43016,
#43017),(#43018,#43019),(#43020,#43021),(#43022,#43023),(#43024,#43025),
(#43026,#43027),(#43028,#43029),(#43030,#43031),(#43032,#43033),(#43034,
#43035),(#43036,#43037),(#43038,#43039),(#43040,#43041),(#43042,#43043),
(#43044,#43045),(#43046,#43047),(#43048,#43049),(#43050,#43051),(#43052,
#43053),(#43054,#43055),(#43056,#43057),(#43058,#43059),(#43060,#43061),
(#43062,#43063),(#43064,#43065),(#43066,#43067),(#43068,#43069),(#43070,
#43071),(#43072,#43073),(#43074,#43075),(#43076,#43077),(#43078,#43079),
(#43080,#43081),(#43082,#43083),(#43084,#43085),(#43086,#43087),(#43088,
#43089),(#43090,#43091),(#43092,#43093),(#43094,#43095),(#43096,#43097),
(#43098,#43099),(#43100,#43101),(#43102,#43103),(#43104,#43105),(#43106,
#43107),(#43108,#43109),(#43110,#43111),(#43112,#43113),(#43114,#43115),
(#43116,#43117),(#43118,#43119),(#43120,#43121),(#43122,#43123),(#43124,
#43125),(#43126,#43127),(#43128,#43129),(#43130,#43131)),.UNSPECIFIED.,
 .F.,.F.,.F.)
B_SPLINE_SURFACE_WITH_KNOTS((6,1,1,1,1,1,1,1,1,1,1,1,1,1,1,1,1,1,1,1,1,
1,1,1,1,1,1,1,1,1,1,1,1,1,1,1,1,1,1,1,1,1,1,1,1,1,1,1,1,1,1,1,1,1,1,1,1,
1,1,1,1,1,1,1,1,6),(2,2),(-1.,-0.984615384615383,-0.969230769230768,-0.953846153846152,
-0.938461538461537,-0.923076923076922,-0.907692307692306,-0.892307692307691,
-0.876923076923076,-0.86153846153846,-0.846153846153845,-0.83076923076923,
-0.815384615384614,-0.799999999999999,-0.784615384615384,-0.769230769230768,
-0.753846153846153,-0.738461538461538,-0.723076923076922,-0.707692307692307,
-0.692307692307692,-0.676923076923076,-0.661538461538461,-0.646153846153846,
-0.63076923076923,-0.615384615384615,-0.6,-0.584615384615384,-0.569230769230769,
-0.553846153846154,-0.538461538461538,-0.523076923076923,-0.507692307692308,
-0.492307692307692,-0.476923076923077,-0.461538461538462,-0.446153846153846,
-0.430769230769231,-0.415384615384615,-0.4,-0.384615384615385,-0.369230769230769,
-0.353846153846154,-0.338461538461538,-0.323076923076923,-0.307692307692308,
-0.292307692307692,-0.276923076923077,-0.261538461538462,-0.246153846153846,
-0.230769230769231,-0.215384615384615,-0.2,-0.184615384615385,-0.169230769230769,
-0.153846153846154,-0.138461538461538,-0.123076923076923,-0.107692307692308,
-0.0923076923076923,-0.0769230769230769,-0.0615384615384615,-0.0461538461538462,
-0.0307692307692308,-0.0153846153846154,0.),(-1.,1.),.UNSPECIFIED.)
GEOMETRIC_REPRESENTATION_ITEM()
RATIONAL_B_SPLINE_SURFACE(((1.,1.),(1.,1.),(1.,1.),(1.,1.),(1.,1.),(1.,
1.),(1.,1.),(1.,1.),(1.,1.),(1.,1.),(1.,1.),(1.,1.),(1.,1.),(1.,1.),(1.,
1.),(1.,1.),(1.,1.),(1.,1.),(1.,1.),(1.,1.),(1.,1.),(1.,1.),(1.,1.),(1.,
1.),(1.,1.),(1.,1.),(1.,1.),(1.,1.),(1.,1.),(1.,1.),(1.,1.),(1.,1.),(1.,
1.),(1.,1.),(1.,1.),(1.,1.),(1.,1.),(1.,1.),(1.,1.),(1.,1.),(1.,1.),(1.,
1.),(1.,1.),(1.,1.),(1.,1.),(1.,1.),(1.,1.),(1.,1.),(1.,1.),(1.,1.),(1.,
1.),(1.,1.),(1.,1.),(1.,1.),(1.,1.),(1.,1.),(1.,1.),(1.,1.),(1.,1.),(1.,
1.),(1.,1.),(1.,1.),(1.,1.),(1.,1.),(1.,1.),(1.,1.),(1.,1.),(1.,1.),(1.,
1.),(1.,1.)))
REPRESENTATION_ITEM('')
SURFACE()
);
#63=(
BOUNDED_SURFACE()
B_SPLINE_SURFACE(5,1,((#43208,#43209),(#43210,#43211),(#43212,#43213),(#43214,
#43215),(#43216,#43217),(#43218,#43219),(#43220,#43221),(#43222,#43223),
(#43224,#43225),(#43226,#43227),(#43228,#43229),(#43230,#43231),(#43232,
#43233),(#43234,#43235),(#43236,#43237),(#43238,#43239),(#43240,#43241),
(#43242,#43243),(#43244,#43245),(#43246,#43247),(#43248,#43249),(#43250,
#43251),(#43252,#43253),(#43254,#43255),(#43256,#43257),(#43258,#43259),
(#43260,#43261),(#43262,#43263),(#43264,#43265),(#43266,#43267),(#43268,
#43269),(#43270,#43271),(#43272,#43273),(#43274,#43275),(#43276,#43277),
(#43278,#43279),(#43280,#43281),(#43282,#43283),(#43284,#43285),(#43286,
#43287),(#43288,#43289),(#43290,#43291),(#43292,#43293),(#43294,#43295),
(#43296,#43297),(#43298,#43299),(#43300,#43301),(#43302,#43303),(#43304,
#43305),(#43306,#43307),(#43308,#43309),(#43310,#43311),(#43312,#43313),
(#43314,#43315),(#43316,#43317),(#43318,#43319),(#43320,#43321),(#43322,
#43323),(#43324,#43325),(#43326,#43327),(#43328,#43329),(#43330,#43331),
(#43332,#43333),(#43334,#43335),(#43336,#43337),(#43338,#43339),(#43340,
#43341),(#43342,#43343),(#43344,#43345),(#43346,#43347)),.UNSPECIFIED.,
 .F.,.F.,.F.)
B_SPLINE_SURFACE_WITH_KNOTS((6,1,1,1,1,1,1,1,1,1,1,1,1,1,1,1,1,1,1,1,1,
1,1,1,1,1,1,1,1,1,1,1,1,1,1,1,1,1,1,1,1,1,1,1,1,1,1,1,1,1,1,1,1,1,1,1,1,
1,1,1,1,1,1,1,1,6),(2,2),(-1.,-0.984615384615383,-0.969230769230768,-0.953846153846152,
-0.938461538461537,-0.923076923076922,-0.907692307692306,-0.892307692307691,
-0.876923076923076,-0.86153846153846,-0.846153846153845,-0.83076923076923,
-0.815384615384614,-0.799999999999999,-0.784615384615384,-0.769230769230768,
-0.753846153846153,-0.738461538461538,-0.723076923076922,-0.707692307692307,
-0.692307692307692,-0.676923076923076,-0.661538461538461,-0.646153846153846,
-0.63076923076923,-0.615384615384615,-0.6,-0.584615384615384,-0.569230769230769,
-0.553846153846154,-0.538461538461538,-0.523076923076923,-0.507692307692308,
-0.492307692307692,-0.476923076923077,-0.461538461538462,-0.446153846153846,
-0.430769230769231,-0.415384615384615,-0.4,-0.384615384615385,-0.369230769230769,
-0.353846153846154,-0.338461538461538,-0.323076923076923,-0.307692307692308,
-0.292307692307692,-0.276923076923077,-0.261538461538462,-0.246153846153846,
-0.230769230769231,-0.215384615384615,-0.2,-0.184615384615385,-0.169230769230769,
-0.153846153846154,-0.138461538461538,-0.123076923076923,-0.107692307692308,
-0.0923076923076923,-0.0769230769230769,-0.0615384615384615,-0.0461538461538462,
-0.0307692307692308,-0.0153846153846154,0.),(-1.,1.),.UNSPECIFIED.)
GEOMETRIC_REPRESENTATION_ITEM()
RATIONAL_B_SPLINE_SURFACE(((1.,1.),(1.,1.),(1.,1.),(1.,1.),(1.,1.),(1.,
1.),(1.,1.),(1.,1.),(1.,1.),(1.,1.),(1.,1.),(1.,1.),(1.,1.),(1.,1.),(1.,
1.),(1.,1.),(1.,1.),(1.,1.),(1.,1.),(1.,1.),(1.,1.),(1.,1.),(1.,1.),(1.,
1.),(1.,1.),(1.,1.),(1.,1.),(1.,1.),(1.,1.),(1.,1.),(1.,1.),(1.,1.),(1.,
1.),(1.,1.),(1.,1.),(1.,1.),(1.,1.),(1.,1.),(1.,1.),(1.,1.),(1.,1.),(1.,
1.),(1.,1.),(1.,1.),(1.,1.),(1.,1.),(1.,1.),(1.,1.),(1.,1.),(1.,1.),(1.,
1.),(1.,1.),(1.,1.),(1.,1.),(1.,1.),(1.,1.),(1.,1.),(1.,1.),(1.,1.),(1.,
1.),(1.,1.),(1.,1.),(1.,1.),(1.,1.),(1.,1.),(1.,1.),(1.,1.),(1.,1.),(1.,
1.),(1.,1.)))
REPRESENTATION_ITEM('')
SURFACE()
);
#64=(
BOUNDED_SURFACE()
B_SPLINE_SURFACE(5,1,((#43424,#43425),(#43426,#43427),(#43428,#43429),(#43430,
#43431),(#43432,#43433),(#43434,#43435),(#43436,#43437),(#43438,#43439),
(#43440,#43441),(#43442,#43443),(#43444,#43445),(#43446,#43447),(#43448,
#43449),(#43450,#43451),(#43452,#43453),(#43454,#43455),(#43456,#43457),
(#43458,#43459),(#43460,#43461),(#43462,#43463),(#43464,#43465),(#43466,
#43467),(#43468,#43469),(#43470,#43471),(#43472,#43473),(#43474,#43475),
(#43476,#43477),(#43478,#43479),(#43480,#43481),(#43482,#43483),(#43484,
#43485),(#43486,#43487),(#43488,#43489),(#43490,#43491),(#43492,#43493),
(#43494,#43495),(#43496,#43497),(#43498,#43499),(#43500,#43501),(#43502,
#43503),(#43504,#43505),(#43506,#43507),(#43508,#43509),(#43510,#43511),
(#43512,#43513),(#43514,#43515),(#43516,#43517),(#43518,#43519),(#43520,
#43521),(#43522,#43523),(#43524,#43525),(#43526,#43527),(#43528,#43529),
(#43530,#43531),(#43532,#43533),(#43534,#43535),(#43536,#43537),(#43538,
#43539),(#43540,#43541),(#43542,#43543),(#43544,#43545),(#43546,#43547),
(#43548,#43549),(#43550,#43551),(#43552,#43553),(#43554,#43555),(#43556,
#43557),(#43558,#43559),(#43560,#43561),(#43562,#43563)),.UNSPECIFIED.,
 .F.,.F.,.F.)
B_SPLINE_SURFACE_WITH_KNOTS((6,1,1,1,1,1,1,1,1,1,1,1,1,1,1,1,1,1,1,1,1,
1,1,1,1,1,1,1,1,1,1,1,1,1,1,1,1,1,1,1,1,1,1,1,1,1,1,1,1,1,1,1,1,1,1,1,1,
1,1,1,1,1,1,1,1,6),(2,2),(-1.,-0.984615384615383,-0.969230769230768,-0.953846153846152,
-0.938461538461537,-0.923076923076922,-0.907692307692306,-0.892307692307691,
-0.876923076923076,-0.86153846153846,-0.846153846153845,-0.83076923076923,
-0.815384615384614,-0.799999999999999,-0.784615384615384,-0.769230769230768,
-0.753846153846153,-0.738461538461538,-0.723076923076922,-0.707692307692307,
-0.692307692307692,-0.676923076923076,-0.661538461538461,-0.646153846153846,
-0.63076923076923,-0.615384615384615,-0.6,-0.584615384615384,-0.569230769230769,
-0.553846153846154,-0.538461538461538,-0.523076923076923,-0.507692307692308,
-0.492307692307692,-0.476923076923077,-0.461538461538462,-0.446153846153846,
-0.430769230769231,-0.415384615384615,-0.4,-0.384615384615385,-0.369230769230769,
-0.353846153846154,-0.338461538461538,-0.323076923076923,-0.307692307692308,
-0.292307692307692,-0.276923076923077,-0.261538461538462,-0.246153846153846,
-0.230769230769231,-0.215384615384615,-0.2,-0.184615384615385,-0.169230769230769,
-0.153846153846154,-0.138461538461538,-0.123076923076923,-0.107692307692308,
-0.0923076923076923,-0.0769230769230769,-0.0615384615384615,-0.0461538461538462,
-0.0307692307692308,-0.0153846153846154,0.),(-1.,1.),.UNSPECIFIED.)
GEOMETRIC_REPRESENTATION_ITEM()
RATIONAL_B_SPLINE_SURFACE(((1.,1.),(1.,1.),(1.,1.),(1.,1.),(1.,1.),(1.,
1.),(1.,1.),(1.,1.),(1.,1.),(1.,1.),(1.,1.),(1.,1.),(1.,1.),(1.,1.),(1.,
1.),(1.,1.),(1.,1.),(1.,1.),(1.,1.),(1.,1.),(1.,1.),(1.,1.),(1.,1.),(1.,
1.),(1.,1.),(1.,1.),(1.,1.),(1.,1.),(1.,1.),(1.,1.),(1.,1.),(1.,1.),(1.,
1.),(1.,1.),(1.,1.),(1.,1.),(1.,1.),(1.,1.),(1.,1.),(1.,1.),(1.,1.),(1.,
1.),(1.,1.),(1.,1.),(1.,1.),(1.,1.),(1.,1.),(1.,1.),(1.,1.),(1.,1.),(1.,
1.),(1.,1.),(1.,1.),(1.,1.),(1.,1.),(1.,1.),(1.,1.),(1.,1.),(1.,1.),(1.,
1.),(1.,1.),(1.,1.),(1.,1.),(1.,1.),(1.,1.),(1.,1.),(1.,1.),(1.,1.),(1.,
1.),(1.,1.)))
REPRESENTATION_ITEM('')
SURFACE()
);
#65=(
BOUNDED_SURFACE()
B_SPLINE_SURFACE(5,1,((#43640,#43641),(#43642,#43643),(#43644,#43645),(#43646,
#43647),(#43648,#43649),(#43650,#43651),(#43652,#43653),(#43654,#43655),
(#43656,#43657),(#43658,#43659),(#43660,#43661),(#43662,#43663),(#43664,
#43665),(#43666,#43667),(#43668,#43669),(#43670,#43671),(#43672,#43673),
(#43674,#43675),(#43676,#43677),(#43678,#43679),(#43680,#43681),(#43682,
#43683),(#43684,#43685),(#43686,#43687),(#43688,#43689),(#43690,#43691),
(#43692,#43693),(#43694,#43695),(#43696,#43697),(#43698,#43699),(#43700,
#43701),(#43702,#43703),(#43704,#43705),(#43706,#43707),(#43708,#43709),
(#43710,#43711),(#43712,#43713),(#43714,#43715),(#43716,#43717),(#43718,
#43719),(#43720,#43721),(#43722,#43723),(#43724,#43725),(#43726,#43727),
(#43728,#43729),(#43730,#43731),(#43732,#43733),(#43734,#43735),(#43736,
#43737),(#43738,#43739),(#43740,#43741),(#43742,#43743),(#43744,#43745),
(#43746,#43747),(#43748,#43749),(#43750,#43751),(#43752,#43753),(#43754,
#43755),(#43756,#43757),(#43758,#43759),(#43760,#43761),(#43762,#43763),
(#43764,#43765),(#43766,#43767),(#43768,#43769),(#43770,#43771),(#43772,
#43773),(#43774,#43775),(#43776,#43777),(#43778,#43779)),.UNSPECIFIED.,
 .F.,.F.,.F.)
B_SPLINE_SURFACE_WITH_KNOTS((6,1,1,1,1,1,1,1,1,1,1,1,1,1,1,1,1,1,1,1,1,
1,1,1,1,1,1,1,1,1,1,1,1,1,1,1,1,1,1,1,1,1,1,1,1,1,1,1,1,1,1,1,1,1,1,1,1,
1,1,1,1,1,1,1,1,6),(2,2),(-1.,-0.984615384615383,-0.969230769230768,-0.953846153846152,
-0.938461538461537,-0.923076923076922,-0.907692307692306,-0.892307692307691,
-0.876923076923076,-0.86153846153846,-0.846153846153845,-0.83076923076923,
-0.815384615384614,-0.799999999999999,-0.784615384615384,-0.769230769230768,
-0.753846153846153,-0.738461538461538,-0.723076923076922,-0.707692307692307,
-0.692307692307692,-0.676923076923076,-0.661538461538461,-0.646153846153846,
-0.63076923076923,-0.615384615384615,-0.6,-0.584615384615384,-0.569230769230769,
-0.553846153846154,-0.538461538461538,-0.523076923076923,-0.507692307692308,
-0.492307692307692,-0.476923076923077,-0.461538461538462,-0.446153846153846,
-0.430769230769231,-0.415384615384615,-0.4,-0.384615384615385,-0.369230769230769,
-0.353846153846154,-0.338461538461538,-0.323076923076923,-0.307692307692308,
-0.292307692307692,-0.276923076923077,-0.261538461538462,-0.246153846153846,
-0.230769230769231,-0.215384615384615,-0.2,-0.184615384615385,-0.169230769230769,
-0.153846153846154,-0.138461538461538,-0.123076923076923,-0.107692307692308,
-0.0923076923076923,-0.0769230769230769,-0.0615384615384615,-0.0461538461538462,
-0.0307692307692308,-0.0153846153846154,0.),(-1.,1.),.UNSPECIFIED.)
GEOMETRIC_REPRESENTATION_ITEM()
RATIONAL_B_SPLINE_SURFACE(((1.,1.),(1.,1.),(1.,1.),(1.,1.),(1.,1.),(1.,
1.),(1.,1.),(1.,1.),(1.,1.),(1.,1.),(1.,1.),(1.,1.),(1.,1.),(1.,1.),(1.,
1.),(1.,1.),(1.,1.),(1.,1.),(1.,1.),(1.,1.),(1.,1.),(1.,1.),(1.,1.),(1.,
1.),(1.,1.),(1.,1.),(1.,1.),(1.,1.),(1.,1.),(1.,1.),(1.,1.),(1.,1.),(1.,
1.),(1.,1.),(1.,1.),(1.,1.),(1.,1.),(1.,1.),(1.,1.),(1.,1.),(1.,1.),(1.,
1.),(1.,1.),(1.,1.),(1.,1.),(1.,1.),(1.,1.),(1.,1.),(1.,1.),(1.,1.),(1.,
1.),(1.,1.),(1.,1.),(1.,1.),(1.,1.),(1.,1.),(1.,1.),(1.,1.),(1.,1.),(1.,
1.),(1.,1.),(1.,1.),(1.,1.),(1.,1.),(1.,1.),(1.,1.),(1.,1.),(1.,1.),(1.,
1.),(1.,1.)))
REPRESENTATION_ITEM('')
SURFACE()
);
#66=(
BOUNDED_SURFACE()
B_SPLINE_SURFACE(5,1,((#43856,#43857),(#43858,#43859),(#43860,#43861),(#43862,
#43863),(#43864,#43865),(#43866,#43867),(#43868,#43869),(#43870,#43871),
(#43872,#43873),(#43874,#43875),(#43876,#43877),(#43878,#43879),(#43880,
#43881),(#43882,#43883),(#43884,#43885),(#43886,#43887),(#43888,#43889),
(#43890,#43891),(#43892,#43893),(#43894,#43895),(#43896,#43897),(#43898,
#43899),(#43900,#43901),(#43902,#43903),(#43904,#43905),(#43906,#43907),
(#43908,#43909),(#43910,#43911),(#43912,#43913),(#43914,#43915),(#43916,
#43917),(#43918,#43919),(#43920,#43921),(#43922,#43923),(#43924,#43925),
(#43926,#43927),(#43928,#43929),(#43930,#43931),(#43932,#43933),(#43934,
#43935),(#43936,#43937),(#43938,#43939),(#43940,#43941),(#43942,#43943),
(#43944,#43945),(#43946,#43947),(#43948,#43949),(#43950,#43951),(#43952,
#43953),(#43954,#43955),(#43956,#43957),(#43958,#43959),(#43960,#43961),
(#43962,#43963),(#43964,#43965),(#43966,#43967),(#43968,#43969),(#43970,
#43971),(#43972,#43973),(#43974,#43975),(#43976,#43977),(#43978,#43979),
(#43980,#43981),(#43982,#43983),(#43984,#43985),(#43986,#43987),(#43988,
#43989),(#43990,#43991),(#43992,#43993),(#43994,#43995)),.UNSPECIFIED.,
 .F.,.F.,.F.)
B_SPLINE_SURFACE_WITH_KNOTS((6,1,1,1,1,1,1,1,1,1,1,1,1,1,1,1,1,1,1,1,1,
1,1,1,1,1,1,1,1,1,1,1,1,1,1,1,1,1,1,1,1,1,1,1,1,1,1,1,1,1,1,1,1,1,1,1,1,
1,1,1,1,1,1,1,1,6),(2,2),(-1.,-0.984615384615383,-0.969230769230768,-0.953846153846152,
-0.938461538461537,-0.923076923076922,-0.907692307692306,-0.892307692307691,
-0.876923076923076,-0.86153846153846,-0.846153846153845,-0.83076923076923,
-0.815384615384614,-0.799999999999999,-0.784615384615384,-0.769230769230768,
-0.753846153846153,-0.738461538461538,-0.723076923076922,-0.707692307692307,
-0.692307692307692,-0.676923076923076,-0.661538461538461,-0.646153846153846,
-0.63076923076923,-0.615384615384615,-0.6,-0.584615384615384,-0.569230769230769,
-0.553846153846154,-0.538461538461538,-0.523076923076923,-0.507692307692308,
-0.492307692307692,-0.476923076923077,-0.461538461538462,-0.446153846153846,
-0.430769230769231,-0.415384615384615,-0.4,-0.384615384615385,-0.369230769230769,
-0.353846153846154,-0.338461538461538,-0.323076923076923,-0.307692307692308,
-0.292307692307692,-0.276923076923077,-0.261538461538462,-0.246153846153846,
-0.230769230769231,-0.215384615384615,-0.2,-0.184615384615385,-0.169230769230769,
-0.153846153846154,-0.138461538461538,-0.123076923076923,-0.107692307692308,
-0.0923076923076923,-0.0769230769230769,-0.0615384615384615,-0.0461538461538462,
-0.0307692307692308,-0.0153846153846154,0.),(-1.,1.),.UNSPECIFIED.)
GEOMETRIC_REPRESENTATION_ITEM()
RATIONAL_B_SPLINE_SURFACE(((1.,1.),(1.,1.),(1.,1.),(1.,1.),(1.,1.),(1.,
1.),(1.,1.),(1.,1.),(1.,1.),(1.,1.),(1.,1.),(1.,1.),(1.,1.),(1.,1.),(1.,
1.),(1.,1.),(1.,1.),(1.,1.),(1.,1.),(1.,1.),(1.,1.),(1.,1.),(1.,1.),(1.,
1.),(1.,1.),(1.,1.),(1.,1.),(1.,1.),(1.,1.),(1.,1.),(1.,1.),(1.,1.),(1.,
1.),(1.,1.),(1.,1.),(1.,1.),(1.,1.),(1.,1.),(1.,1.),(1.,1.),(1.,1.),(1.,
1.),(1.,1.),(1.,1.),(1.,1.),(1.,1.),(1.,1.),(1.,1.),(1.,1.),(1.,1.),(1.,
1.),(1.,1.),(1.,1.),(1.,1.),(1.,1.),(1.,1.),(1.,1.),(1.,1.),(1.,1.),(1.,
1.),(1.,1.),(1.,1.),(1.,1.),(1.,1.),(1.,1.),(1.,1.),(1.,1.),(1.,1.),(1.,
1.),(1.,1.)))
REPRESENTATION_ITEM('')
SURFACE()
);
#67=(
BOUNDED_SURFACE()
B_SPLINE_SURFACE(5,1,((#44072,#44073),(#44074,#44075),(#44076,#44077),(#44078,
#44079),(#44080,#44081),(#44082,#44083),(#44084,#44085),(#44086,#44087),
(#44088,#44089),(#44090,#44091),(#44092,#44093),(#44094,#44095),(#44096,
#44097),(#44098,#44099),(#44100,#44101),(#44102,#44103),(#44104,#44105),
(#44106,#44107),(#44108,#44109),(#44110,#44111),(#44112,#44113),(#44114,
#44115),(#44116,#44117),(#44118,#44119),(#44120,#44121),(#44122,#44123),
(#44124,#44125),(#44126,#44127),(#44128,#44129),(#44130,#44131),(#44132,
#44133),(#44134,#44135),(#44136,#44137),(#44138,#44139),(#44140,#44141),
(#44142,#44143),(#44144,#44145),(#44146,#44147),(#44148,#44149),(#44150,
#44151),(#44152,#44153),(#44154,#44155),(#44156,#44157),(#44158,#44159),
(#44160,#44161),(#44162,#44163),(#44164,#44165),(#44166,#44167),(#44168,
#44169),(#44170,#44171),(#44172,#44173),(#44174,#44175),(#44176,#44177),
(#44178,#44179),(#44180,#44181),(#44182,#44183),(#44184,#44185),(#44186,
#44187),(#44188,#44189),(#44190,#44191),(#44192,#44193),(#44194,#44195),
(#44196,#44197),(#44198,#44199),(#44200,#44201),(#44202,#44203),(#44204,
#44205),(#44206,#44207),(#44208,#44209),(#44210,#44211)),.UNSPECIFIED.,
 .F.,.F.,.F.)
B_SPLINE_SURFACE_WITH_KNOTS((6,1,1,1,1,1,1,1,1,1,1,1,1,1,1,1,1,1,1,1,1,
1,1,1,1,1,1,1,1,1,1,1,1,1,1,1,1,1,1,1,1,1,1,1,1,1,1,1,1,1,1,1,1,1,1,1,1,
1,1,1,1,1,1,1,1,6),(2,2),(-1.,-0.984615384615383,-0.969230769230768,-0.953846153846152,
-0.938461538461537,-0.923076923076922,-0.907692307692306,-0.892307692307691,
-0.876923076923076,-0.86153846153846,-0.846153846153845,-0.83076923076923,
-0.815384615384614,-0.799999999999999,-0.784615384615384,-0.769230769230768,
-0.753846153846153,-0.738461538461538,-0.723076923076922,-0.707692307692307,
-0.692307692307692,-0.676923076923076,-0.661538461538461,-0.646153846153846,
-0.63076923076923,-0.615384615384615,-0.6,-0.584615384615384,-0.569230769230769,
-0.553846153846154,-0.538461538461538,-0.523076923076923,-0.507692307692308,
-0.492307692307692,-0.476923076923077,-0.461538461538462,-0.446153846153846,
-0.430769230769231,-0.415384615384615,-0.4,-0.384615384615385,-0.369230769230769,
-0.353846153846154,-0.338461538461538,-0.323076923076923,-0.307692307692308,
-0.292307692307692,-0.276923076923077,-0.261538461538462,-0.246153846153846,
-0.230769230769231,-0.215384615384615,-0.2,-0.184615384615385,-0.169230769230769,
-0.153846153846154,-0.138461538461538,-0.123076923076923,-0.107692307692308,
-0.0923076923076923,-0.0769230769230769,-0.0615384615384615,-0.0461538461538462,
-0.0307692307692308,-0.0153846153846154,0.),(-1.,1.),.UNSPECIFIED.)
GEOMETRIC_REPRESENTATION_ITEM()
RATIONAL_B_SPLINE_SURFACE(((1.,1.),(1.,1.),(1.,1.),(1.,1.),(1.,1.),(1.,
1.),(1.,1.),(1.,1.),(1.,1.),(1.,1.),(1.,1.),(1.,1.),(1.,1.),(1.,1.),(1.,
1.),(1.,1.),(1.,1.),(1.,1.),(1.,1.),(1.,1.),(1.,1.),(1.,1.),(1.,1.),(1.,
1.),(1.,1.),(1.,1.),(1.,1.),(1.,1.),(1.,1.),(1.,1.),(1.,1.),(1.,1.),(1.,
1.),(1.,1.),(1.,1.),(1.,1.),(1.,1.),(1.,1.),(1.,1.),(1.,1.),(1.,1.),(1.,
1.),(1.,1.),(1.,1.),(1.,1.),(1.,1.),(1.,1.),(1.,1.),(1.,1.),(1.,1.),(1.,
1.),(1.,1.),(1.,1.),(1.,1.),(1.,1.),(1.,1.),(1.,1.),(1.,1.),(1.,1.),(1.,
1.),(1.,1.),(1.,1.),(1.,1.),(1.,1.),(1.,1.),(1.,1.),(1.,1.),(1.,1.),(1.,
1.),(1.,1.)))
REPRESENTATION_ITEM('')
SURFACE()
);
#68=(
BOUNDED_SURFACE()
B_SPLINE_SURFACE(5,1,((#44288,#44289),(#44290,#44291),(#44292,#44293),(#44294,
#44295),(#44296,#44297),(#44298,#44299),(#44300,#44301),(#44302,#44303),
(#44304,#44305),(#44306,#44307),(#44308,#44309),(#44310,#44311),(#44312,
#44313),(#44314,#44315),(#44316,#44317),(#44318,#44319),(#44320,#44321),
(#44322,#44323),(#44324,#44325),(#44326,#44327),(#44328,#44329),(#44330,
#44331),(#44332,#44333),(#44334,#44335),(#44336,#44337),(#44338,#44339),
(#44340,#44341),(#44342,#44343),(#44344,#44345),(#44346,#44347),(#44348,
#44349),(#44350,#44351),(#44352,#44353),(#44354,#44355),(#44356,#44357),
(#44358,#44359),(#44360,#44361),(#44362,#44363),(#44364,#44365),(#44366,
#44367),(#44368,#44369),(#44370,#44371),(#44372,#44373),(#44374,#44375),
(#44376,#44377),(#44378,#44379),(#44380,#44381),(#44382,#44383),(#44384,
#44385),(#44386,#44387),(#44388,#44389),(#44390,#44391),(#44392,#44393),
(#44394,#44395),(#44396,#44397),(#44398,#44399),(#44400,#44401),(#44402,
#44403),(#44404,#44405),(#44406,#44407),(#44408,#44409),(#44410,#44411),
(#44412,#44413),(#44414,#44415),(#44416,#44417),(#44418,#44419),(#44420,
#44421),(#44422,#44423),(#44424,#44425),(#44426,#44427)),.UNSPECIFIED.,
 .F.,.F.,.F.)
B_SPLINE_SURFACE_WITH_KNOTS((6,1,1,1,1,1,1,1,1,1,1,1,1,1,1,1,1,1,1,1,1,
1,1,1,1,1,1,1,1,1,1,1,1,1,1,1,1,1,1,1,1,1,1,1,1,1,1,1,1,1,1,1,1,1,1,1,1,
1,1,1,1,1,1,1,1,6),(2,2),(-1.,-0.984615384615383,-0.969230769230768,-0.953846153846152,
-0.938461538461537,-0.923076923076922,-0.907692307692306,-0.892307692307691,
-0.876923076923076,-0.86153846153846,-0.846153846153845,-0.83076923076923,
-0.815384615384614,-0.799999999999999,-0.784615384615384,-0.769230769230768,
-0.753846153846153,-0.738461538461538,-0.723076923076922,-0.707692307692307,
-0.692307692307692,-0.676923076923076,-0.661538461538461,-0.646153846153846,
-0.63076923076923,-0.615384615384615,-0.6,-0.584615384615384,-0.569230769230769,
-0.553846153846154,-0.538461538461538,-0.523076923076923,-0.507692307692308,
-0.492307692307692,-0.476923076923077,-0.461538461538462,-0.446153846153846,
-0.430769230769231,-0.415384615384615,-0.4,-0.384615384615385,-0.369230769230769,
-0.353846153846154,-0.338461538461538,-0.323076923076923,-0.307692307692308,
-0.292307692307692,-0.276923076923077,-0.261538461538462,-0.246153846153846,
-0.230769230769231,-0.215384615384615,-0.2,-0.184615384615385,-0.169230769230769,
-0.153846153846154,-0.138461538461538,-0.123076923076923,-0.107692307692308,
-0.0923076923076923,-0.0769230769230769,-0.0615384615384615,-0.0461538461538462,
-0.0307692307692308,-0.0153846153846154,0.),(-1.,1.),.UNSPECIFIED.)
GEOMETRIC_REPRESENTATION_ITEM()
RATIONAL_B_SPLINE_SURFACE(((1.,1.),(1.,1.),(1.,1.),(1.,1.),(1.,1.),(1.,
1.),(1.,1.),(1.,1.),(1.,1.),(1.,1.),(1.,1.),(1.,1.),(1.,1.),(1.,1.),(1.,
1.),(1.,1.),(1.,1.),(1.,1.),(1.,1.),(1.,1.),(1.,1.),(1.,1.),(1.,1.),(1.,
1.),(1.,1.),(1.,1.),(1.,1.),(1.,1.),(1.,1.),(1.,1.),(1.,1.),(1.,1.),(1.,
1.),(1.,1.),(1.,1.),(1.,1.),(1.,1.),(1.,1.),(1.,1.),(1.,1.),(1.,1.),(1.,
1.),(1.,1.),(1.,1.),(1.,1.),(1.,1.),(1.,1.),(1.,1.),(1.,1.),(1.,1.),(1.,
1.),(1.,1.),(1.,1.),(1.,1.),(1.,1.),(1.,1.),(1.,1.),(1.,1.),(1.,1.),(1.,
1.),(1.,1.),(1.,1.),(1.,1.),(1.,1.),(1.,1.),(1.,1.),(1.,1.),(1.,1.),(1.,
1.),(1.,1.)))
REPRESENTATION_ITEM('')
SURFACE()
);
#69=(
BOUNDED_SURFACE()
B_SPLINE_SURFACE(5,1,((#44504,#44505),(#44506,#44507),(#44508,#44509),(#44510,
#44511),(#44512,#44513),(#44514,#44515),(#44516,#44517),(#44518,#44519),
(#44520,#44521),(#44522,#44523),(#44524,#44525),(#44526,#44527),(#44528,
#44529),(#44530,#44531),(#44532,#44533),(#44534,#44535),(#44536,#44537),
(#44538,#44539),(#44540,#44541),(#44542,#44543),(#44544,#44545),(#44546,
#44547),(#44548,#44549),(#44550,#44551),(#44552,#44553),(#44554,#44555),
(#44556,#44557),(#44558,#44559),(#44560,#44561),(#44562,#44563),(#44564,
#44565),(#44566,#44567),(#44568,#44569),(#44570,#44571),(#44572,#44573),
(#44574,#44575),(#44576,#44577),(#44578,#44579),(#44580,#44581),(#44582,
#44583),(#44584,#44585),(#44586,#44587),(#44588,#44589),(#44590,#44591),
(#44592,#44593),(#44594,#44595),(#44596,#44597),(#44598,#44599),(#44600,
#44601),(#44602,#44603),(#44604,#44605),(#44606,#44607),(#44608,#44609),
(#44610,#44611),(#44612,#44613),(#44614,#44615),(#44616,#44617),(#44618,
#44619),(#44620,#44621),(#44622,#44623),(#44624,#44625),(#44626,#44627),
(#44628,#44629),(#44630,#44631),(#44632,#44633),(#44634,#44635),(#44636,
#44637),(#44638,#44639),(#44640,#44641),(#44642,#44643)),.UNSPECIFIED.,
 .F.,.F.,.F.)
B_SPLINE_SURFACE_WITH_KNOTS((6,1,1,1,1,1,1,1,1,1,1,1,1,1,1,1,1,1,1,1,1,
1,1,1,1,1,1,1,1,1,1,1,1,1,1,1,1,1,1,1,1,1,1,1,1,1,1,1,1,1,1,1,1,1,1,1,1,
1,1,1,1,1,1,1,1,6),(2,2),(-1.,-0.984615384615383,-0.969230769230768,-0.953846153846152,
-0.938461538461537,-0.923076923076922,-0.907692307692306,-0.892307692307691,
-0.876923076923076,-0.86153846153846,-0.846153846153845,-0.83076923076923,
-0.815384615384614,-0.799999999999999,-0.784615384615384,-0.769230769230768,
-0.753846153846153,-0.738461538461538,-0.723076923076922,-0.707692307692307,
-0.692307692307692,-0.676923076923076,-0.661538461538461,-0.646153846153846,
-0.63076923076923,-0.615384615384615,-0.6,-0.584615384615384,-0.569230769230769,
-0.553846153846154,-0.538461538461538,-0.523076923076923,-0.507692307692308,
-0.492307692307692,-0.476923076923077,-0.461538461538462,-0.446153846153846,
-0.430769230769231,-0.415384615384615,-0.4,-0.384615384615385,-0.369230769230769,
-0.353846153846154,-0.338461538461538,-0.323076923076923,-0.307692307692308,
-0.292307692307692,-0.276923076923077,-0.261538461538462,-0.246153846153846,
-0.230769230769231,-0.215384615384615,-0.2,-0.184615384615385,-0.169230769230769,
-0.153846153846154,-0.138461538461538,-0.123076923076923,-0.107692307692308,
-0.0923076923076923,-0.0769230769230769,-0.0615384615384615,-0.0461538461538462,
-0.0307692307692308,-0.0153846153846154,0.),(-1.,1.),.UNSPECIFIED.)
GEOMETRIC_REPRESENTATION_ITEM()
RATIONAL_B_SPLINE_SURFACE(((1.,1.),(1.,1.),(1.,1.),(1.,1.),(1.,1.),(1.,
1.),(1.,1.),(1.,1.),(1.,1.),(1.,1.),(1.,1.),(1.,1.),(1.,1.),(1.,1.),(1.,
1.),(1.,1.),(1.,1.),(1.,1.),(1.,1.),(1.,1.),(1.,1.),(1.,1.),(1.,1.),(1.,
1.),(1.,1.),(1.,1.),(1.,1.),(1.,1.),(1.,1.),(1.,1.),(1.,1.),(1.,1.),(1.,
1.),(1.,1.),(1.,1.),(1.,1.),(1.,1.),(1.,1.),(1.,1.),(1.,1.),(1.,1.),(1.,
1.),(1.,1.),(1.,1.),(1.,1.),(1.,1.),(1.,1.),(1.,1.),(1.,1.),(1.,1.),(1.,
1.),(1.,1.),(1.,1.),(1.,1.),(1.,1.),(1.,1.),(1.,1.),(1.,1.),(1.,1.),(1.,
1.),(1.,1.),(1.,1.),(1.,1.),(1.,1.),(1.,1.),(1.,1.),(1.,1.),(1.,1.),(1.,
1.),(1.,1.)))
REPRESENTATION_ITEM('')
SURFACE()
);
#70=(
BOUNDED_SURFACE()
B_SPLINE_SURFACE(5,1,((#44720,#44721),(#44722,#44723),(#44724,#44725),(#44726,
#44727),(#44728,#44729),(#44730,#44731),(#44732,#44733),(#44734,#44735),
(#44736,#44737),(#44738,#44739),(#44740,#44741),(#44742,#44743),(#44744,
#44745),(#44746,#44747),(#44748,#44749),(#44750,#44751),(#44752,#44753),
(#44754,#44755),(#44756,#44757),(#44758,#44759),(#44760,#44761),(#44762,
#44763),(#44764,#44765),(#44766,#44767),(#44768,#44769),(#44770,#44771),
(#44772,#44773),(#44774,#44775),(#44776,#44777),(#44778,#44779),(#44780,
#44781),(#44782,#44783),(#44784,#44785),(#44786,#44787),(#44788,#44789),
(#44790,#44791),(#44792,#44793),(#44794,#44795),(#44796,#44797),(#44798,
#44799),(#44800,#44801),(#44802,#44803),(#44804,#44805),(#44806,#44807),
(#44808,#44809),(#44810,#44811),(#44812,#44813),(#44814,#44815),(#44816,
#44817),(#44818,#44819),(#44820,#44821),(#44822,#44823),(#44824,#44825),
(#44826,#44827),(#44828,#44829),(#44830,#44831),(#44832,#44833),(#44834,
#44835),(#44836,#44837),(#44838,#44839),(#44840,#44841),(#44842,#44843),
(#44844,#44845),(#44846,#44847),(#44848,#44849),(#44850,#44851),(#44852,
#44853),(#44854,#44855),(#44856,#44857),(#44858,#44859)),.UNSPECIFIED.,
 .F.,.F.,.F.)
B_SPLINE_SURFACE_WITH_KNOTS((6,1,1,1,1,1,1,1,1,1,1,1,1,1,1,1,1,1,1,1,1,
1,1,1,1,1,1,1,1,1,1,1,1,1,1,1,1,1,1,1,1,1,1,1,1,1,1,1,1,1,1,1,1,1,1,1,1,
1,1,1,1,1,1,1,1,6),(2,2),(-1.,-0.984615384615383,-0.969230769230768,-0.953846153846152,
-0.938461538461537,-0.923076923076922,-0.907692307692306,-0.892307692307691,
-0.876923076923076,-0.86153846153846,-0.846153846153845,-0.83076923076923,
-0.815384615384614,-0.799999999999999,-0.784615384615384,-0.769230769230768,
-0.753846153846153,-0.738461538461538,-0.723076923076922,-0.707692307692307,
-0.692307692307692,-0.676923076923076,-0.661538461538461,-0.646153846153846,
-0.63076923076923,-0.615384615384615,-0.6,-0.584615384615384,-0.569230769230769,
-0.553846153846154,-0.538461538461538,-0.523076923076923,-0.507692307692308,
-0.492307692307692,-0.476923076923077,-0.461538461538462,-0.446153846153846,
-0.430769230769231,-0.415384615384615,-0.4,-0.384615384615385,-0.369230769230769,
-0.353846153846154,-0.338461538461538,-0.323076923076923,-0.307692307692308,
-0.292307692307692,-0.276923076923077,-0.261538461538462,-0.246153846153846,
-0.230769230769231,-0.215384615384615,-0.2,-0.184615384615385,-0.169230769230769,
-0.153846153846154,-0.138461538461538,-0.123076923076923,-0.107692307692308,
-0.0923076923076923,-0.0769230769230769,-0.0615384615384615,-0.0461538461538462,
-0.0307692307692308,-0.0153846153846154,0.),(-1.,1.),.UNSPECIFIED.)
GEOMETRIC_REPRESENTATION_ITEM()
RATIONAL_B_SPLINE_SURFACE(((1.,1.),(1.,1.),(1.,1.),(1.,1.),(1.,1.),(1.,
1.),(1.,1.),(1.,1.),(1.,1.),(1.,1.),(1.,1.),(1.,1.),(1.,1.),(1.,1.),(1.,
1.),(1.,1.),(1.,1.),(1.,1.),(1.,1.),(1.,1.),(1.,1.),(1.,1.),(1.,1.),(1.,
1.),(1.,1.),(1.,1.),(1.,1.),(1.,1.),(1.,1.),(1.,1.),(1.,1.),(1.,1.),(1.,
1.),(1.,1.),(1.,1.),(1.,1.),(1.,1.),(1.,1.),(1.,1.),(1.,1.),(1.,1.),(1.,
1.),(1.,1.),(1.,1.),(1.,1.),(1.,1.),(1.,1.),(1.,1.),(1.,1.),(1.,1.),(1.,
1.),(1.,1.),(1.,1.),(1.,1.),(1.,1.),(1.,1.),(1.,1.),(1.,1.),(1.,1.),(1.,
1.),(1.,1.),(1.,1.),(1.,1.),(1.,1.),(1.,1.),(1.,1.),(1.,1.),(1.,1.),(1.,
1.),(1.,1.)))
REPRESENTATION_ITEM('')
SURFACE()
);
#71=(
BOUNDED_SURFACE()
B_SPLINE_SURFACE(5,1,((#44936,#44937),(#44938,#44939),(#44940,#44941),(#44942,
#44943),(#44944,#44945),(#44946,#44947),(#44948,#44949),(#44950,#44951),
(#44952,#44953),(#44954,#44955),(#44956,#44957),(#44958,#44959),(#44960,
#44961),(#44962,#44963),(#44964,#44965),(#44966,#44967),(#44968,#44969),
(#44970,#44971),(#44972,#44973),(#44974,#44975),(#44976,#44977),(#44978,
#44979),(#44980,#44981),(#44982,#44983),(#44984,#44985),(#44986,#44987),
(#44988,#44989),(#44990,#44991),(#44992,#44993),(#44994,#44995),(#44996,
#44997),(#44998,#44999),(#45000,#45001),(#45002,#45003),(#45004,#45005),
(#45006,#45007),(#45008,#45009),(#45010,#45011),(#45012,#45013),(#45014,
#45015),(#45016,#45017),(#45018,#45019),(#45020,#45021),(#45022,#45023),
(#45024,#45025),(#45026,#45027),(#45028,#45029),(#45030,#45031),(#45032,
#45033),(#45034,#45035),(#45036,#45037),(#45038,#45039),(#45040,#45041),
(#45042,#45043),(#45044,#45045),(#45046,#45047),(#45048,#45049),(#45050,
#45051),(#45052,#45053),(#45054,#45055),(#45056,#45057),(#45058,#45059),
(#45060,#45061),(#45062,#45063),(#45064,#45065),(#45066,#45067),(#45068,
#45069),(#45070,#45071),(#45072,#45073),(#45074,#45075)),.UNSPECIFIED.,
 .F.,.F.,.F.)
B_SPLINE_SURFACE_WITH_KNOTS((6,1,1,1,1,1,1,1,1,1,1,1,1,1,1,1,1,1,1,1,1,
1,1,1,1,1,1,1,1,1,1,1,1,1,1,1,1,1,1,1,1,1,1,1,1,1,1,1,1,1,1,1,1,1,1,1,1,
1,1,1,1,1,1,1,1,6),(2,2),(-1.,-0.984615384615383,-0.969230769230768,-0.953846153846152,
-0.938461538461537,-0.923076923076922,-0.907692307692306,-0.892307692307691,
-0.876923076923076,-0.86153846153846,-0.846153846153845,-0.83076923076923,
-0.815384615384614,-0.799999999999999,-0.784615384615384,-0.769230769230768,
-0.753846153846153,-0.738461538461538,-0.723076923076922,-0.707692307692307,
-0.692307692307692,-0.676923076923076,-0.661538461538461,-0.646153846153846,
-0.63076923076923,-0.615384615384615,-0.6,-0.584615384615384,-0.569230769230769,
-0.553846153846154,-0.538461538461538,-0.523076923076923,-0.507692307692308,
-0.492307692307692,-0.476923076923077,-0.461538461538462,-0.446153846153846,
-0.430769230769231,-0.415384615384615,-0.4,-0.384615384615385,-0.369230769230769,
-0.353846153846154,-0.338461538461538,-0.323076923076923,-0.307692307692308,
-0.292307692307692,-0.276923076923077,-0.261538461538462,-0.246153846153846,
-0.230769230769231,-0.215384615384615,-0.2,-0.184615384615385,-0.169230769230769,
-0.153846153846154,-0.138461538461538,-0.123076923076923,-0.107692307692308,
-0.0923076923076923,-0.0769230769230769,-0.0615384615384615,-0.0461538461538462,
-0.0307692307692308,-0.0153846153846154,0.),(-1.,1.),.UNSPECIFIED.)
GEOMETRIC_REPRESENTATION_ITEM()
RATIONAL_B_SPLINE_SURFACE(((1.,1.),(1.,1.),(1.,1.),(1.,1.),(1.,1.),(1.,
1.),(1.,1.),(1.,1.),(1.,1.),(1.,1.),(1.,1.),(1.,1.),(1.,1.),(1.,1.),(1.,
1.),(1.,1.),(1.,1.),(1.,1.),(1.,1.),(1.,1.),(1.,1.),(1.,1.),(1.,1.),(1.,
1.),(1.,1.),(1.,1.),(1.,1.),(1.,1.),(1.,1.),(1.,1.),(1.,1.),(1.,1.),(1.,
1.),(1.,1.),(1.,1.),(1.,1.),(1.,1.),(1.,1.),(1.,1.),(1.,1.),(1.,1.),(1.,
1.),(1.,1.),(1.,1.),(1.,1.),(1.,1.),(1.,1.),(1.,1.),(1.,1.),(1.,1.),(1.,
1.),(1.,1.),(1.,1.),(1.,1.),(1.,1.),(1.,1.),(1.,1.),(1.,1.),(1.,1.),(1.,
1.),(1.,1.),(1.,1.),(1.,1.),(1.,1.),(1.,1.),(1.,1.),(1.,1.),(1.,1.),(1.,
1.),(1.,1.)))
REPRESENTATION_ITEM('')
SURFACE()
);
#72=(
BOUNDED_SURFACE()
B_SPLINE_SURFACE(5,1,((#45152,#45153),(#45154,#45155),(#45156,#45157),(#45158,
#45159),(#45160,#45161),(#45162,#45163),(#45164,#45165),(#45166,#45167),
(#45168,#45169),(#45170,#45171),(#45172,#45173),(#45174,#45175),(#45176,
#45177),(#45178,#45179),(#45180,#45181),(#45182,#45183),(#45184,#45185),
(#45186,#45187),(#45188,#45189),(#45190,#45191),(#45192,#45193),(#45194,
#45195),(#45196,#45197),(#45198,#45199),(#45200,#45201),(#45202,#45203),
(#45204,#45205),(#45206,#45207),(#45208,#45209),(#45210,#45211),(#45212,
#45213),(#45214,#45215),(#45216,#45217),(#45218,#45219),(#45220,#45221),
(#45222,#45223),(#45224,#45225),(#45226,#45227),(#45228,#45229),(#45230,
#45231),(#45232,#45233),(#45234,#45235),(#45236,#45237),(#45238,#45239),
(#45240,#45241),(#45242,#45243),(#45244,#45245),(#45246,#45247),(#45248,
#45249),(#45250,#45251),(#45252,#45253),(#45254,#45255),(#45256,#45257),
(#45258,#45259),(#45260,#45261),(#45262,#45263),(#45264,#45265),(#45266,
#45267),(#45268,#45269),(#45270,#45271),(#45272,#45273),(#45274,#45275),
(#45276,#45277),(#45278,#45279),(#45280,#45281),(#45282,#45283),(#45284,
#45285),(#45286,#45287),(#45288,#45289),(#45290,#45291)),.UNSPECIFIED.,
 .F.,.F.,.F.)
B_SPLINE_SURFACE_WITH_KNOTS((6,1,1,1,1,1,1,1,1,1,1,1,1,1,1,1,1,1,1,1,1,
1,1,1,1,1,1,1,1,1,1,1,1,1,1,1,1,1,1,1,1,1,1,1,1,1,1,1,1,1,1,1,1,1,1,1,1,
1,1,1,1,1,1,1,1,6),(2,2),(-1.,-0.984615384615383,-0.969230769230768,-0.953846153846152,
-0.938461538461537,-0.923076923076922,-0.907692307692306,-0.892307692307691,
-0.876923076923076,-0.86153846153846,-0.846153846153845,-0.83076923076923,
-0.815384615384614,-0.799999999999999,-0.784615384615384,-0.769230769230768,
-0.753846153846153,-0.738461538461538,-0.723076923076922,-0.707692307692307,
-0.692307692307692,-0.676923076923076,-0.661538461538461,-0.646153846153846,
-0.63076923076923,-0.615384615384615,-0.6,-0.584615384615384,-0.569230769230769,
-0.553846153846154,-0.538461538461538,-0.523076923076923,-0.507692307692308,
-0.492307692307692,-0.476923076923077,-0.461538461538462,-0.446153846153846,
-0.430769230769231,-0.415384615384615,-0.4,-0.384615384615385,-0.369230769230769,
-0.353846153846154,-0.338461538461538,-0.323076923076923,-0.307692307692308,
-0.292307692307692,-0.276923076923077,-0.261538461538462,-0.246153846153846,
-0.230769230769231,-0.215384615384615,-0.2,-0.184615384615385,-0.169230769230769,
-0.153846153846154,-0.138461538461538,-0.123076923076923,-0.107692307692308,
-0.0923076923076923,-0.0769230769230769,-0.0615384615384615,-0.0461538461538462,
-0.0307692307692308,-0.0153846153846154,0.),(-1.,1.),.UNSPECIFIED.)
GEOMETRIC_REPRESENTATION_ITEM()
RATIONAL_B_SPLINE_SURFACE(((1.,1.),(1.,1.),(1.,1.),(1.,1.),(1.,1.),(1.,
1.),(1.,1.),(1.,1.),(1.,1.),(1.,1.),(1.,1.),(1.,1.),(1.,1.),(1.,1.),(1.,
1.),(1.,1.),(1.,1.),(1.,1.),(1.,1.),(1.,1.),(1.,1.),(1.,1.),(1.,1.),(1.,
1.),(1.,1.),(1.,1.),(1.,1.),(1.,1.),(1.,1.),(1.,1.),(1.,1.),(1.,1.),(1.,
1.),(1.,1.),(1.,1.),(1.,1.),(1.,1.),(1.,1.),(1.,1.),(1.,1.),(1.,1.),(1.,
1.),(1.,1.),(1.,1.),(1.,1.),(1.,1.),(1.,1.),(1.,1.),(1.,1.),(1.,1.),(1.,
1.),(1.,1.),(1.,1.),(1.,1.),(1.,1.),(1.,1.),(1.,1.),(1.,1.),(1.,1.),(1.,
1.),(1.,1.),(1.,1.),(1.,1.),(1.,1.),(1.,1.),(1.,1.),(1.,1.),(1.,1.),(1.,
1.),(1.,1.)))
REPRESENTATION_ITEM('')
SURFACE()
);
#73=(
BOUNDED_SURFACE()
B_SPLINE_SURFACE(5,1,((#45368,#45369),(#45370,#45371),(#45372,#45373),(#45374,
#45375),(#45376,#45377),(#45378,#45379),(#45380,#45381),(#45382,#45383),
(#45384,#45385),(#45386,#45387),(#45388,#45389),(#45390,#45391),(#45392,
#45393),(#45394,#45395),(#45396,#45397),(#45398,#45399),(#45400,#45401),
(#45402,#45403),(#45404,#45405),(#45406,#45407),(#45408,#45409),(#45410,
#45411),(#45412,#45413),(#45414,#45415),(#45416,#45417),(#45418,#45419),
(#45420,#45421),(#45422,#45423),(#45424,#45425),(#45426,#45427),(#45428,
#45429),(#45430,#45431),(#45432,#45433),(#45434,#45435),(#45436,#45437),
(#45438,#45439),(#45440,#45441),(#45442,#45443),(#45444,#45445),(#45446,
#45447),(#45448,#45449),(#45450,#45451),(#45452,#45453),(#45454,#45455),
(#45456,#45457),(#45458,#45459),(#45460,#45461),(#45462,#45463),(#45464,
#45465),(#45466,#45467),(#45468,#45469),(#45470,#45471),(#45472,#45473),
(#45474,#45475),(#45476,#45477),(#45478,#45479),(#45480,#45481),(#45482,
#45483),(#45484,#45485),(#45486,#45487),(#45488,#45489),(#45490,#45491),
(#45492,#45493),(#45494,#45495),(#45496,#45497),(#45498,#45499),(#45500,
#45501),(#45502,#45503),(#45504,#45505),(#45506,#45507)),.UNSPECIFIED.,
 .F.,.F.,.F.)
B_SPLINE_SURFACE_WITH_KNOTS((6,1,1,1,1,1,1,1,1,1,1,1,1,1,1,1,1,1,1,1,1,
1,1,1,1,1,1,1,1,1,1,1,1,1,1,1,1,1,1,1,1,1,1,1,1,1,1,1,1,1,1,1,1,1,1,1,1,
1,1,1,1,1,1,1,1,6),(2,2),(-1.,-0.984615384615383,-0.969230769230768,-0.953846153846152,
-0.938461538461537,-0.923076923076922,-0.907692307692306,-0.892307692307691,
-0.876923076923076,-0.86153846153846,-0.846153846153845,-0.83076923076923,
-0.815384615384614,-0.799999999999999,-0.784615384615384,-0.769230769230768,
-0.753846153846153,-0.738461538461538,-0.723076923076922,-0.707692307692307,
-0.692307692307692,-0.676923076923076,-0.661538461538461,-0.646153846153846,
-0.63076923076923,-0.615384615384615,-0.6,-0.584615384615384,-0.569230769230769,
-0.553846153846154,-0.538461538461538,-0.523076923076923,-0.507692307692308,
-0.492307692307692,-0.476923076923077,-0.461538461538462,-0.446153846153846,
-0.430769230769231,-0.415384615384615,-0.4,-0.384615384615385,-0.369230769230769,
-0.353846153846154,-0.338461538461538,-0.323076923076923,-0.307692307692308,
-0.292307692307692,-0.276923076923077,-0.261538461538462,-0.246153846153846,
-0.230769230769231,-0.215384615384615,-0.2,-0.184615384615385,-0.169230769230769,
-0.153846153846154,-0.138461538461538,-0.123076923076923,-0.107692307692308,
-0.0923076923076923,-0.0769230769230769,-0.0615384615384615,-0.0461538461538462,
-0.0307692307692308,-0.0153846153846154,0.),(-1.,1.),.UNSPECIFIED.)
GEOMETRIC_REPRESENTATION_ITEM()
RATIONAL_B_SPLINE_SURFACE(((1.,1.),(1.,1.),(1.,1.),(1.,1.),(1.,1.),(1.,
1.),(1.,1.),(1.,1.),(1.,1.),(1.,1.),(1.,1.),(1.,1.),(1.,1.),(1.,1.),(1.,
1.),(1.,1.),(1.,1.),(1.,1.),(1.,1.),(1.,1.),(1.,1.),(1.,1.),(1.,1.),(1.,
1.),(1.,1.),(1.,1.),(1.,1.),(1.,1.),(1.,1.),(1.,1.),(1.,1.),(1.,1.),(1.,
1.),(1.,1.),(1.,1.),(1.,1.),(1.,1.),(1.,1.),(1.,1.),(1.,1.),(1.,1.),(1.,
1.),(1.,1.),(1.,1.),(1.,1.),(1.,1.),(1.,1.),(1.,1.),(1.,1.),(1.,1.),(1.,
1.),(1.,1.),(1.,1.),(1.,1.),(1.,1.),(1.,1.),(1.,1.),(1.,1.),(1.,1.),(1.,
1.),(1.,1.),(1.,1.),(1.,1.),(1.,1.),(1.,1.),(1.,1.),(1.,1.),(1.,1.),(1.,
1.),(1.,1.)))
REPRESENTATION_ITEM('')
SURFACE()
);
#74=(
BOUNDED_SURFACE()
B_SPLINE_SURFACE(5,1,((#45584,#45585),(#45586,#45587),(#45588,#45589),(#45590,
#45591),(#45592,#45593),(#45594,#45595),(#45596,#45597),(#45598,#45599),
(#45600,#45601),(#45602,#45603),(#45604,#45605),(#45606,#45607),(#45608,
#45609),(#45610,#45611),(#45612,#45613),(#45614,#45615),(#45616,#45617),
(#45618,#45619),(#45620,#45621),(#45622,#45623),(#45624,#45625),(#45626,
#45627),(#45628,#45629),(#45630,#45631),(#45632,#45633),(#45634,#45635),
(#45636,#45637),(#45638,#45639),(#45640,#45641),(#45642,#45643),(#45644,
#45645),(#45646,#45647),(#45648,#45649),(#45650,#45651),(#45652,#45653),
(#45654,#45655),(#45656,#45657),(#45658,#45659),(#45660,#45661),(#45662,
#45663),(#45664,#45665),(#45666,#45667),(#45668,#45669),(#45670,#45671),
(#45672,#45673),(#45674,#45675),(#45676,#45677),(#45678,#45679),(#45680,
#45681),(#45682,#45683),(#45684,#45685),(#45686,#45687),(#45688,#45689),
(#45690,#45691),(#45692,#45693),(#45694,#45695),(#45696,#45697),(#45698,
#45699),(#45700,#45701),(#45702,#45703),(#45704,#45705),(#45706,#45707),
(#45708,#45709),(#45710,#45711),(#45712,#45713),(#45714,#45715),(#45716,
#45717),(#45718,#45719),(#45720,#45721),(#45722,#45723)),.UNSPECIFIED.,
 .F.,.F.,.F.)
B_SPLINE_SURFACE_WITH_KNOTS((6,1,1,1,1,1,1,1,1,1,1,1,1,1,1,1,1,1,1,1,1,
1,1,1,1,1,1,1,1,1,1,1,1,1,1,1,1,1,1,1,1,1,1,1,1,1,1,1,1,1,1,1,1,1,1,1,1,
1,1,1,1,1,1,1,1,6),(2,2),(-1.,-0.984615384615383,-0.969230769230768,-0.953846153846152,
-0.938461538461537,-0.923076923076922,-0.907692307692306,-0.892307692307691,
-0.876923076923076,-0.86153846153846,-0.846153846153845,-0.83076923076923,
-0.815384615384614,-0.799999999999999,-0.784615384615384,-0.769230769230768,
-0.753846153846153,-0.738461538461538,-0.723076923076922,-0.707692307692307,
-0.692307692307692,-0.676923076923076,-0.661538461538461,-0.646153846153846,
-0.63076923076923,-0.615384615384615,-0.6,-0.584615384615384,-0.569230769230769,
-0.553846153846154,-0.538461538461538,-0.523076923076923,-0.507692307692308,
-0.492307692307692,-0.476923076923077,-0.461538461538462,-0.446153846153846,
-0.430769230769231,-0.415384615384615,-0.4,-0.384615384615385,-0.369230769230769,
-0.353846153846154,-0.338461538461538,-0.323076923076923,-0.307692307692308,
-0.292307692307692,-0.276923076923077,-0.261538461538462,-0.246153846153846,
-0.230769230769231,-0.215384615384615,-0.2,-0.184615384615385,-0.169230769230769,
-0.153846153846154,-0.138461538461538,-0.123076923076923,-0.107692307692308,
-0.0923076923076923,-0.0769230769230769,-0.0615384615384615,-0.0461538461538462,
-0.0307692307692308,-0.0153846153846154,0.),(-1.,1.),.UNSPECIFIED.)
GEOMETRIC_REPRESENTATION_ITEM()
RATIONAL_B_SPLINE_SURFACE(((1.,1.),(1.,1.),(1.,1.),(1.,1.),(1.,1.),(1.,
1.),(1.,1.),(1.,1.),(1.,1.),(1.,1.),(1.,1.),(1.,1.),(1.,1.),(1.,1.),(1.,
1.),(1.,1.),(1.,1.),(1.,1.),(1.,1.),(1.,1.),(1.,1.),(1.,1.),(1.,1.),(1.,
1.),(1.,1.),(1.,1.),(1.,1.),(1.,1.),(1.,1.),(1.,1.),(1.,1.),(1.,1.),(1.,
1.),(1.,1.),(1.,1.),(1.,1.),(1.,1.),(1.,1.),(1.,1.),(1.,1.),(1.,1.),(1.,
1.),(1.,1.),(1.,1.),(1.,1.),(1.,1.),(1.,1.),(1.,1.),(1.,1.),(1.,1.),(1.,
1.),(1.,1.),(1.,1.),(1.,1.),(1.,1.),(1.,1.),(1.,1.),(1.,1.),(1.,1.),(1.,
1.),(1.,1.),(1.,1.),(1.,1.),(1.,1.),(1.,1.),(1.,1.),(1.,1.),(1.,1.),(1.,
1.),(1.,1.)))
REPRESENTATION_ITEM('')
SURFACE()
);
#75=(
BOUNDED_SURFACE()
B_SPLINE_SURFACE(5,1,((#45800,#45801),(#45802,#45803),(#45804,#45805),(#45806,
#45807),(#45808,#45809),(#45810,#45811),(#45812,#45813),(#45814,#45815),
(#45816,#45817),(#45818,#45819),(#45820,#45821),(#45822,#45823),(#45824,
#45825),(#45826,#45827),(#45828,#45829),(#45830,#45831),(#45832,#45833),
(#45834,#45835),(#45836,#45837),(#45838,#45839),(#45840,#45841),(#45842,
#45843),(#45844,#45845),(#45846,#45847),(#45848,#45849),(#45850,#45851),
(#45852,#45853),(#45854,#45855),(#45856,#45857),(#45858,#45859),(#45860,
#45861),(#45862,#45863),(#45864,#45865),(#45866,#45867),(#45868,#45869),
(#45870,#45871),(#45872,#45873),(#45874,#45875),(#45876,#45877),(#45878,
#45879),(#45880,#45881),(#45882,#45883),(#45884,#45885),(#45886,#45887),
(#45888,#45889),(#45890,#45891),(#45892,#45893),(#45894,#45895),(#45896,
#45897),(#45898,#45899),(#45900,#45901),(#45902,#45903),(#45904,#45905),
(#45906,#45907),(#45908,#45909),(#45910,#45911),(#45912,#45913),(#45914,
#45915),(#45916,#45917),(#45918,#45919),(#45920,#45921),(#45922,#45923),
(#45924,#45925),(#45926,#45927),(#45928,#45929),(#45930,#45931),(#45932,
#45933),(#45934,#45935),(#45936,#45937),(#45938,#45939)),.UNSPECIFIED.,
 .F.,.F.,.F.)
B_SPLINE_SURFACE_WITH_KNOTS((6,1,1,1,1,1,1,1,1,1,1,1,1,1,1,1,1,1,1,1,1,
1,1,1,1,1,1,1,1,1,1,1,1,1,1,1,1,1,1,1,1,1,1,1,1,1,1,1,1,1,1,1,1,1,1,1,1,
1,1,1,1,1,1,1,1,6),(2,2),(-1.,-0.984615384615383,-0.969230769230768,-0.953846153846152,
-0.938461538461537,-0.923076923076922,-0.907692307692306,-0.892307692307691,
-0.876923076923076,-0.86153846153846,-0.846153846153845,-0.83076923076923,
-0.815384615384614,-0.799999999999999,-0.784615384615384,-0.769230769230768,
-0.753846153846153,-0.738461538461538,-0.723076923076922,-0.707692307692307,
-0.692307692307692,-0.676923076923076,-0.661538461538461,-0.646153846153846,
-0.63076923076923,-0.615384615384615,-0.6,-0.584615384615384,-0.569230769230769,
-0.553846153846154,-0.538461538461538,-0.523076923076923,-0.507692307692308,
-0.492307692307692,-0.476923076923077,-0.461538461538462,-0.446153846153846,
-0.430769230769231,-0.415384615384615,-0.4,-0.384615384615385,-0.369230769230769,
-0.353846153846154,-0.338461538461538,-0.323076923076923,-0.307692307692308,
-0.292307692307692,-0.276923076923077,-0.261538461538462,-0.246153846153846,
-0.230769230769231,-0.215384615384615,-0.2,-0.184615384615385,-0.169230769230769,
-0.153846153846154,-0.138461538461538,-0.123076923076923,-0.107692307692308,
-0.0923076923076923,-0.0769230769230769,-0.0615384615384615,-0.0461538461538462,
-0.0307692307692308,-0.0153846153846154,0.),(-1.,1.),.UNSPECIFIED.)
GEOMETRIC_REPRESENTATION_ITEM()
RATIONAL_B_SPLINE_SURFACE(((1.,1.),(1.,1.),(1.,1.),(1.,1.),(1.,1.),(1.,
1.),(1.,1.),(1.,1.),(1.,1.),(1.,1.),(1.,1.),(1.,1.),(1.,1.),(1.,1.),(1.,
1.),(1.,1.),(1.,1.),(1.,1.),(1.,1.),(1.,1.),(1.,1.),(1.,1.),(1.,1.),(1.,
1.),(1.,1.),(1.,1.),(1.,1.),(1.,1.),(1.,1.),(1.,1.),(1.,1.),(1.,1.),(1.,
1.),(1.,1.),(1.,1.),(1.,1.),(1.,1.),(1.,1.),(1.,1.),(1.,1.),(1.,1.),(1.,
1.),(1.,1.),(1.,1.),(1.,1.),(1.,1.),(1.,1.),(1.,1.),(1.,1.),(1.,1.),(1.,
1.),(1.,1.),(1.,1.),(1.,1.),(1.,1.),(1.,1.),(1.,1.),(1.,1.),(1.,1.),(1.,
1.),(1.,1.),(1.,1.),(1.,1.),(1.,1.),(1.,1.),(1.,1.),(1.,1.),(1.,1.),(1.,
1.),(1.,1.)))
REPRESENTATION_ITEM('')
SURFACE()
);
#76=(
BOUNDED_SURFACE()
B_SPLINE_SURFACE(5,1,((#46016,#46017),(#46018,#46019),(#46020,#46021),(#46022,
#46023),(#46024,#46025),(#46026,#46027),(#46028,#46029),(#46030,#46031),
(#46032,#46033),(#46034,#46035),(#46036,#46037),(#46038,#46039),(#46040,
#46041),(#46042,#46043),(#46044,#46045),(#46046,#46047),(#46048,#46049),
(#46050,#46051),(#46052,#46053),(#46054,#46055),(#46056,#46057),(#46058,
#46059),(#46060,#46061),(#46062,#46063),(#46064,#46065),(#46066,#46067),
(#46068,#46069),(#46070,#46071),(#46072,#46073),(#46074,#46075),(#46076,
#46077),(#46078,#46079),(#46080,#46081),(#46082,#46083),(#46084,#46085),
(#46086,#46087),(#46088,#46089),(#46090,#46091),(#46092,#46093),(#46094,
#46095),(#46096,#46097),(#46098,#46099),(#46100,#46101),(#46102,#46103),
(#46104,#46105),(#46106,#46107),(#46108,#46109),(#46110,#46111),(#46112,
#46113),(#46114,#46115),(#46116,#46117),(#46118,#46119),(#46120,#46121),
(#46122,#46123),(#46124,#46125),(#46126,#46127),(#46128,#46129),(#46130,
#46131),(#46132,#46133),(#46134,#46135),(#46136,#46137),(#46138,#46139),
(#46140,#46141),(#46142,#46143),(#46144,#46145),(#46146,#46147),(#46148,
#46149),(#46150,#46151),(#46152,#46153),(#46154,#46155)),.UNSPECIFIED.,
 .F.,.F.,.F.)
B_SPLINE_SURFACE_WITH_KNOTS((6,1,1,1,1,1,1,1,1,1,1,1,1,1,1,1,1,1,1,1,1,
1,1,1,1,1,1,1,1,1,1,1,1,1,1,1,1,1,1,1,1,1,1,1,1,1,1,1,1,1,1,1,1,1,1,1,1,
1,1,1,1,1,1,1,1,6),(2,2),(-1.,-0.984615384615383,-0.969230769230768,-0.953846153846152,
-0.938461538461537,-0.923076923076922,-0.907692307692306,-0.892307692307691,
-0.876923076923076,-0.86153846153846,-0.846153846153845,-0.83076923076923,
-0.815384615384614,-0.799999999999999,-0.784615384615384,-0.769230769230768,
-0.753846153846153,-0.738461538461538,-0.723076923076922,-0.707692307692307,
-0.692307692307692,-0.676923076923076,-0.661538461538461,-0.646153846153846,
-0.63076923076923,-0.615384615384615,-0.6,-0.584615384615384,-0.569230769230769,
-0.553846153846154,-0.538461538461538,-0.523076923076923,-0.507692307692308,
-0.492307692307692,-0.476923076923077,-0.461538461538462,-0.446153846153846,
-0.430769230769231,-0.415384615384615,-0.4,-0.384615384615385,-0.369230769230769,
-0.353846153846154,-0.338461538461538,-0.323076923076923,-0.307692307692308,
-0.292307692307692,-0.276923076923077,-0.261538461538462,-0.246153846153846,
-0.230769230769231,-0.215384615384615,-0.2,-0.184615384615385,-0.169230769230769,
-0.153846153846154,-0.138461538461538,-0.123076923076923,-0.107692307692308,
-0.0923076923076923,-0.0769230769230769,-0.0615384615384615,-0.0461538461538462,
-0.0307692307692308,-0.0153846153846154,0.),(-1.,1.),.UNSPECIFIED.)
GEOMETRIC_REPRESENTATION_ITEM()
RATIONAL_B_SPLINE_SURFACE(((1.,1.),(1.,1.),(1.,1.),(1.,1.),(1.,1.),(1.,
1.),(1.,1.),(1.,1.),(1.,1.),(1.,1.),(1.,1.),(1.,1.),(1.,1.),(1.,1.),(1.,
1.),(1.,1.),(1.,1.),(1.,1.),(1.,1.),(1.,1.),(1.,1.),(1.,1.),(1.,1.),(1.,
1.),(1.,1.),(1.,1.),(1.,1.),(1.,1.),(1.,1.),(1.,1.),(1.,1.),(1.,1.),(1.,
1.),(1.,1.),(1.,1.),(1.,1.),(1.,1.),(1.,1.),(1.,1.),(1.,1.),(1.,1.),(1.,
1.),(1.,1.),(1.,1.),(1.,1.),(1.,1.),(1.,1.),(1.,1.),(1.,1.),(1.,1.),(1.,
1.),(1.,1.),(1.,1.),(1.,1.),(1.,1.),(1.,1.),(1.,1.),(1.,1.),(1.,1.),(1.,
1.),(1.,1.),(1.,1.),(1.,1.),(1.,1.),(1.,1.),(1.,1.),(1.,1.),(1.,1.),(1.,
1.),(1.,1.)))
REPRESENTATION_ITEM('')
SURFACE()
);
#77=(
BOUNDED_SURFACE()
B_SPLINE_SURFACE(5,1,((#46232,#46233),(#46234,#46235),(#46236,#46237),(#46238,
#46239),(#46240,#46241),(#46242,#46243),(#46244,#46245),(#46246,#46247),
(#46248,#46249),(#46250,#46251),(#46252,#46253),(#46254,#46255),(#46256,
#46257),(#46258,#46259),(#46260,#46261),(#46262,#46263),(#46264,#46265),
(#46266,#46267),(#46268,#46269),(#46270,#46271),(#46272,#46273),(#46274,
#46275),(#46276,#46277),(#46278,#46279),(#46280,#46281),(#46282,#46283),
(#46284,#46285),(#46286,#46287),(#46288,#46289),(#46290,#46291),(#46292,
#46293),(#46294,#46295),(#46296,#46297),(#46298,#46299),(#46300,#46301),
(#46302,#46303),(#46304,#46305),(#46306,#46307),(#46308,#46309),(#46310,
#46311),(#46312,#46313),(#46314,#46315),(#46316,#46317),(#46318,#46319),
(#46320,#46321),(#46322,#46323),(#46324,#46325),(#46326,#46327),(#46328,
#46329),(#46330,#46331),(#46332,#46333),(#46334,#46335),(#46336,#46337),
(#46338,#46339),(#46340,#46341),(#46342,#46343),(#46344,#46345),(#46346,
#46347),(#46348,#46349),(#46350,#46351),(#46352,#46353),(#46354,#46355),
(#46356,#46357),(#46358,#46359),(#46360,#46361),(#46362,#46363),(#46364,
#46365),(#46366,#46367),(#46368,#46369),(#46370,#46371)),.UNSPECIFIED.,
 .F.,.F.,.F.)
B_SPLINE_SURFACE_WITH_KNOTS((6,1,1,1,1,1,1,1,1,1,1,1,1,1,1,1,1,1,1,1,1,
1,1,1,1,1,1,1,1,1,1,1,1,1,1,1,1,1,1,1,1,1,1,1,1,1,1,1,1,1,1,1,1,1,1,1,1,
1,1,1,1,1,1,1,1,6),(2,2),(-1.,-0.984615384615383,-0.969230769230768,-0.953846153846152,
-0.938461538461537,-0.923076923076922,-0.907692307692306,-0.892307692307691,
-0.876923076923076,-0.86153846153846,-0.846153846153845,-0.83076923076923,
-0.815384615384614,-0.799999999999999,-0.784615384615384,-0.769230769230768,
-0.753846153846153,-0.738461538461538,-0.723076923076922,-0.707692307692307,
-0.692307692307692,-0.676923076923076,-0.661538461538461,-0.646153846153846,
-0.63076923076923,-0.615384615384615,-0.6,-0.584615384615384,-0.569230769230769,
-0.553846153846154,-0.538461538461538,-0.523076923076923,-0.507692307692308,
-0.492307692307692,-0.476923076923077,-0.461538461538462,-0.446153846153846,
-0.430769230769231,-0.415384615384615,-0.4,-0.384615384615385,-0.369230769230769,
-0.353846153846154,-0.338461538461538,-0.323076923076923,-0.307692307692308,
-0.292307692307692,-0.276923076923077,-0.261538461538462,-0.246153846153846,
-0.230769230769231,-0.215384615384615,-0.2,-0.184615384615385,-0.169230769230769,
-0.153846153846154,-0.138461538461538,-0.123076923076923,-0.107692307692308,
-0.0923076923076923,-0.0769230769230769,-0.0615384615384615,-0.0461538461538462,
-0.0307692307692308,-0.0153846153846154,0.),(-1.,1.),.UNSPECIFIED.)
GEOMETRIC_REPRESENTATION_ITEM()
RATIONAL_B_SPLINE_SURFACE(((1.,1.),(1.,1.),(1.,1.),(1.,1.),(1.,1.),(1.,
1.),(1.,1.),(1.,1.),(1.,1.),(1.,1.),(1.,1.),(1.,1.),(1.,1.),(1.,1.),(1.,
1.),(1.,1.),(1.,1.),(1.,1.),(1.,1.),(1.,1.),(1.,1.),(1.,1.),(1.,1.),(1.,
1.),(1.,1.),(1.,1.),(1.,1.),(1.,1.),(1.,1.),(1.,1.),(1.,1.),(1.,1.),(1.,
1.),(1.,1.),(1.,1.),(1.,1.),(1.,1.),(1.,1.),(1.,1.),(1.,1.),(1.,1.),(1.,
1.),(1.,1.),(1.,1.),(1.,1.),(1.,1.),(1.,1.),(1.,1.),(1.,1.),(1.,1.),(1.,
1.),(1.,1.),(1.,1.),(1.,1.),(1.,1.),(1.,1.),(1.,1.),(1.,1.),(1.,1.),(1.,
1.),(1.,1.),(1.,1.),(1.,1.),(1.,1.),(1.,1.),(1.,1.),(1.,1.),(1.,1.),(1.,
1.),(1.,1.)))
REPRESENTATION_ITEM('')
SURFACE()
);
#78=(
BOUNDED_SURFACE()
B_SPLINE_SURFACE(5,1,((#46448,#46449),(#46450,#46451),(#46452,#46453),(#46454,
#46455),(#46456,#46457),(#46458,#46459),(#46460,#46461),(#46462,#46463),
(#46464,#46465),(#46466,#46467),(#46468,#46469),(#46470,#46471),(#46472,
#46473),(#46474,#46475),(#46476,#46477),(#46478,#46479),(#46480,#46481),
(#46482,#46483),(#46484,#46485),(#46486,#46487),(#46488,#46489),(#46490,
#46491),(#46492,#46493),(#46494,#46495),(#46496,#46497),(#46498,#46499),
(#46500,#46501),(#46502,#46503),(#46504,#46505),(#46506,#46507),(#46508,
#46509),(#46510,#46511),(#46512,#46513),(#46514,#46515),(#46516,#46517),
(#46518,#46519),(#46520,#46521),(#46522,#46523),(#46524,#46525),(#46526,
#46527),(#46528,#46529),(#46530,#46531),(#46532,#46533),(#46534,#46535),
(#46536,#46537),(#46538,#46539),(#46540,#46541),(#46542,#46543),(#46544,
#46545),(#46546,#46547),(#46548,#46549),(#46550,#46551),(#46552,#46553),
(#46554,#46555),(#46556,#46557),(#46558,#46559),(#46560,#46561),(#46562,
#46563),(#46564,#46565),(#46566,#46567),(#46568,#46569),(#46570,#46571),
(#46572,#46573),(#46574,#46575),(#46576,#46577),(#46578,#46579),(#46580,
#46581),(#46582,#46583),(#46584,#46585),(#46586,#46587)),.UNSPECIFIED.,
 .F.,.F.,.F.)
B_SPLINE_SURFACE_WITH_KNOTS((6,1,1,1,1,1,1,1,1,1,1,1,1,1,1,1,1,1,1,1,1,
1,1,1,1,1,1,1,1,1,1,1,1,1,1,1,1,1,1,1,1,1,1,1,1,1,1,1,1,1,1,1,1,1,1,1,1,
1,1,1,1,1,1,1,1,6),(2,2),(-1.,-0.984615384615383,-0.969230769230768,-0.953846153846152,
-0.938461538461537,-0.923076923076922,-0.907692307692306,-0.892307692307691,
-0.876923076923076,-0.86153846153846,-0.846153846153845,-0.83076923076923,
-0.815384615384614,-0.799999999999999,-0.784615384615384,-0.769230769230768,
-0.753846153846153,-0.738461538461538,-0.723076923076922,-0.707692307692307,
-0.692307692307692,-0.676923076923076,-0.661538461538461,-0.646153846153846,
-0.63076923076923,-0.615384615384615,-0.6,-0.584615384615384,-0.569230769230769,
-0.553846153846154,-0.538461538461538,-0.523076923076923,-0.507692307692308,
-0.492307692307692,-0.476923076923077,-0.461538461538462,-0.446153846153846,
-0.430769230769231,-0.415384615384615,-0.4,-0.384615384615385,-0.369230769230769,
-0.353846153846154,-0.338461538461538,-0.323076923076923,-0.307692307692308,
-0.292307692307692,-0.276923076923077,-0.261538461538462,-0.246153846153846,
-0.230769230769231,-0.215384615384615,-0.2,-0.184615384615385,-0.169230769230769,
-0.153846153846154,-0.138461538461538,-0.123076923076923,-0.107692307692308,
-0.0923076923076923,-0.0769230769230769,-0.0615384615384615,-0.0461538461538462,
-0.0307692307692308,-0.0153846153846154,0.),(-1.,1.),.UNSPECIFIED.)
GEOMETRIC_REPRESENTATION_ITEM()
RATIONAL_B_SPLINE_SURFACE(((1.,1.),(1.,1.),(1.,1.),(1.,1.),(1.,1.),(1.,
1.),(1.,1.),(1.,1.),(1.,1.),(1.,1.),(1.,1.),(1.,1.),(1.,1.),(1.,1.),(1.,
1.),(1.,1.),(1.,1.),(1.,1.),(1.,1.),(1.,1.),(1.,1.),(1.,1.),(1.,1.),(1.,
1.),(1.,1.),(1.,1.),(1.,1.),(1.,1.),(1.,1.),(1.,1.),(1.,1.),(1.,1.),(1.,
1.),(1.,1.),(1.,1.),(1.,1.),(1.,1.),(1.,1.),(1.,1.),(1.,1.),(1.,1.),(1.,
1.),(1.,1.),(1.,1.),(1.,1.),(1.,1.),(1.,1.),(1.,1.),(1.,1.),(1.,1.),(1.,
1.),(1.,1.),(1.,1.),(1.,1.),(1.,1.),(1.,1.),(1.,1.),(1.,1.),(1.,1.),(1.,
1.),(1.,1.),(1.,1.),(1.,1.),(1.,1.),(1.,1.),(1.,1.),(1.,1.),(1.,1.),(1.,
1.),(1.,1.)))
REPRESENTATION_ITEM('')
SURFACE()
);
#79=(
BOUNDED_SURFACE()
B_SPLINE_SURFACE(5,1,((#46664,#46665),(#46666,#46667),(#46668,#46669),(#46670,
#46671),(#46672,#46673),(#46674,#46675),(#46676,#46677),(#46678,#46679),
(#46680,#46681),(#46682,#46683),(#46684,#46685),(#46686,#46687),(#46688,
#46689),(#46690,#46691),(#46692,#46693),(#46694,#46695),(#46696,#46697),
(#46698,#46699),(#46700,#46701),(#46702,#46703),(#46704,#46705),(#46706,
#46707),(#46708,#46709),(#46710,#46711),(#46712,#46713),(#46714,#46715),
(#46716,#46717),(#46718,#46719),(#46720,#46721),(#46722,#46723),(#46724,
#46725),(#46726,#46727),(#46728,#46729),(#46730,#46731),(#46732,#46733),
(#46734,#46735),(#46736,#46737),(#46738,#46739),(#46740,#46741),(#46742,
#46743),(#46744,#46745),(#46746,#46747),(#46748,#46749),(#46750,#46751),
(#46752,#46753),(#46754,#46755),(#46756,#46757),(#46758,#46759),(#46760,
#46761),(#46762,#46763),(#46764,#46765),(#46766,#46767),(#46768,#46769),
(#46770,#46771),(#46772,#46773),(#46774,#46775),(#46776,#46777),(#46778,
#46779),(#46780,#46781),(#46782,#46783),(#46784,#46785),(#46786,#46787),
(#46788,#46789),(#46790,#46791),(#46792,#46793),(#46794,#46795),(#46796,
#46797),(#46798,#46799),(#46800,#46801),(#46802,#46803)),.UNSPECIFIED.,
 .F.,.F.,.F.)
B_SPLINE_SURFACE_WITH_KNOTS((6,1,1,1,1,1,1,1,1,1,1,1,1,1,1,1,1,1,1,1,1,
1,1,1,1,1,1,1,1,1,1,1,1,1,1,1,1,1,1,1,1,1,1,1,1,1,1,1,1,1,1,1,1,1,1,1,1,
1,1,1,1,1,1,1,1,6),(2,2),(-1.,-0.984615384615383,-0.969230769230768,-0.953846153846152,
-0.938461538461537,-0.923076923076922,-0.907692307692306,-0.892307692307691,
-0.876923076923076,-0.86153846153846,-0.846153846153845,-0.83076923076923,
-0.815384615384614,-0.799999999999999,-0.784615384615384,-0.769230769230768,
-0.753846153846153,-0.738461538461538,-0.723076923076922,-0.707692307692307,
-0.692307692307692,-0.676923076923076,-0.661538461538461,-0.646153846153846,
-0.63076923076923,-0.615384615384615,-0.6,-0.584615384615384,-0.569230769230769,
-0.553846153846154,-0.538461538461538,-0.523076923076923,-0.507692307692308,
-0.492307692307692,-0.476923076923077,-0.461538461538462,-0.446153846153846,
-0.430769230769231,-0.415384615384615,-0.4,-0.384615384615385,-0.369230769230769,
-0.353846153846154,-0.338461538461538,-0.323076923076923,-0.307692307692308,
-0.292307692307692,-0.276923076923077,-0.261538461538462,-0.246153846153846,
-0.230769230769231,-0.215384615384615,-0.2,-0.184615384615385,-0.169230769230769,
-0.153846153846154,-0.138461538461538,-0.123076923076923,-0.107692307692308,
-0.0923076923076923,-0.0769230769230769,-0.0615384615384615,-0.0461538461538462,
-0.0307692307692308,-0.0153846153846154,0.),(-1.,1.),.UNSPECIFIED.)
GEOMETRIC_REPRESENTATION_ITEM()
RATIONAL_B_SPLINE_SURFACE(((1.,1.),(1.,1.),(1.,1.),(1.,1.),(1.,1.),(1.,
1.),(1.,1.),(1.,1.),(1.,1.),(1.,1.),(1.,1.),(1.,1.),(1.,1.),(1.,1.),(1.,
1.),(1.,1.),(1.,1.),(1.,1.),(1.,1.),(1.,1.),(1.,1.),(1.,1.),(1.,1.),(1.,
1.),(1.,1.),(1.,1.),(1.,1.),(1.,1.),(1.,1.),(1.,1.),(1.,1.),(1.,1.),(1.,
1.),(1.,1.),(1.,1.),(1.,1.),(1.,1.),(1.,1.),(1.,1.),(1.,1.),(1.,1.),(1.,
1.),(1.,1.),(1.,1.),(1.,1.),(1.,1.),(1.,1.),(1.,1.),(1.,1.),(1.,1.),(1.,
1.),(1.,1.),(1.,1.),(1.,1.),(1.,1.),(1.,1.),(1.,1.),(1.,1.),(1.,1.),(1.,
1.),(1.,1.),(1.,1.),(1.,1.),(1.,1.),(1.,1.),(1.,1.),(1.,1.),(1.,1.),(1.,
1.),(1.,1.)))
REPRESENTATION_ITEM('')
SURFACE()
);
#80=(
BOUNDED_SURFACE()
B_SPLINE_SURFACE(5,1,((#46880,#46881),(#46882,#46883),(#46884,#46885),(#46886,
#46887),(#46888,#46889),(#46890,#46891),(#46892,#46893),(#46894,#46895),
(#46896,#46897),(#46898,#46899),(#46900,#46901),(#46902,#46903),(#46904,
#46905),(#46906,#46907),(#46908,#46909),(#46910,#46911),(#46912,#46913),
(#46914,#46915),(#46916,#46917),(#46918,#46919),(#46920,#46921),(#46922,
#46923),(#46924,#46925),(#46926,#46927),(#46928,#46929),(#46930,#46931),
(#46932,#46933),(#46934,#46935),(#46936,#46937),(#46938,#46939),(#46940,
#46941),(#46942,#46943),(#46944,#46945),(#46946,#46947),(#46948,#46949),
(#46950,#46951),(#46952,#46953),(#46954,#46955),(#46956,#46957),(#46958,
#46959),(#46960,#46961),(#46962,#46963),(#46964,#46965),(#46966,#46967),
(#46968,#46969),(#46970,#46971),(#46972,#46973),(#46974,#46975),(#46976,
#46977),(#46978,#46979),(#46980,#46981),(#46982,#46983),(#46984,#46985),
(#46986,#46987),(#46988,#46989),(#46990,#46991),(#46992,#46993),(#46994,
#46995),(#46996,#46997),(#46998,#46999),(#47000,#47001),(#47002,#47003),
(#47004,#47005),(#47006,#47007),(#47008,#47009),(#47010,#47011),(#47012,
#47013),(#47014,#47015),(#47016,#47017),(#47018,#47019)),.UNSPECIFIED.,
 .F.,.F.,.F.)
B_SPLINE_SURFACE_WITH_KNOTS((6,1,1,1,1,1,1,1,1,1,1,1,1,1,1,1,1,1,1,1,1,
1,1,1,1,1,1,1,1,1,1,1,1,1,1,1,1,1,1,1,1,1,1,1,1,1,1,1,1,1,1,1,1,1,1,1,1,
1,1,1,1,1,1,1,1,6),(2,2),(-1.,-0.984615384615383,-0.969230769230768,-0.953846153846152,
-0.938461538461537,-0.923076923076922,-0.907692307692306,-0.892307692307691,
-0.876923076923076,-0.86153846153846,-0.846153846153845,-0.83076923076923,
-0.815384615384614,-0.799999999999999,-0.784615384615384,-0.769230769230768,
-0.753846153846153,-0.738461538461538,-0.723076923076922,-0.707692307692307,
-0.692307692307692,-0.676923076923076,-0.661538461538461,-0.646153846153846,
-0.63076923076923,-0.615384615384615,-0.6,-0.584615384615384,-0.569230769230769,
-0.553846153846154,-0.538461538461538,-0.523076923076923,-0.507692307692308,
-0.492307692307692,-0.476923076923077,-0.461538461538462,-0.446153846153846,
-0.430769230769231,-0.415384615384615,-0.4,-0.384615384615385,-0.369230769230769,
-0.353846153846154,-0.338461538461538,-0.323076923076923,-0.307692307692308,
-0.292307692307692,-0.276923076923077,-0.261538461538462,-0.246153846153846,
-0.230769230769231,-0.215384615384615,-0.2,-0.184615384615385,-0.169230769230769,
-0.153846153846154,-0.138461538461538,-0.123076923076923,-0.107692307692308,
-0.0923076923076923,-0.0769230769230769,-0.0615384615384615,-0.0461538461538462,
-0.0307692307692308,-0.0153846153846154,0.),(-1.,1.),.UNSPECIFIED.)
GEOMETRIC_REPRESENTATION_ITEM()
RATIONAL_B_SPLINE_SURFACE(((1.,1.),(1.,1.),(1.,1.),(1.,1.),(1.,1.),(1.,
1.),(1.,1.),(1.,1.),(1.,1.),(1.,1.),(1.,1.),(1.,1.),(1.,1.),(1.,1.),(1.,
1.),(1.,1.),(1.,1.),(1.,1.),(1.,1.),(1.,1.),(1.,1.),(1.,1.),(1.,1.),(1.,
1.),(1.,1.),(1.,1.),(1.,1.),(1.,1.),(1.,1.),(1.,1.),(1.,1.),(1.,1.),(1.,
1.),(1.,1.),(1.,1.),(1.,1.),(1.,1.),(1.,1.),(1.,1.),(1.,1.),(1.,1.),(1.,
1.),(1.,1.),(1.,1.),(1.,1.),(1.,1.),(1.,1.),(1.,1.),(1.,1.),(1.,1.),(1.,
1.),(1.,1.),(1.,1.),(1.,1.),(1.,1.),(1.,1.),(1.,1.),(1.,1.),(1.,1.),(1.,
1.),(1.,1.),(1.,1.),(1.,1.),(1.,1.),(1.,1.),(1.,1.),(1.,1.),(1.,1.),(1.,
1.),(1.,1.)))
REPRESENTATION_ITEM('')
SURFACE()
);
#81=(
BOUNDED_SURFACE()
B_SPLINE_SURFACE(5,1,((#47096,#47097),(#47098,#47099),(#47100,#47101),(#47102,
#47103),(#47104,#47105),(#47106,#47107),(#47108,#47109),(#47110,#47111),
(#47112,#47113),(#47114,#47115),(#47116,#47117),(#47118,#47119),(#47120,
#47121),(#47122,#47123),(#47124,#47125),(#47126,#47127),(#47128,#47129),
(#47130,#47131),(#47132,#47133),(#47134,#47135),(#47136,#47137),(#47138,
#47139),(#47140,#47141),(#47142,#47143),(#47144,#47145),(#47146,#47147),
(#47148,#47149),(#47150,#47151),(#47152,#47153),(#47154,#47155),(#47156,
#47157),(#47158,#47159),(#47160,#47161),(#47162,#47163),(#47164,#47165),
(#47166,#47167),(#47168,#47169),(#47170,#47171),(#47172,#47173),(#47174,
#47175),(#47176,#47177),(#47178,#47179),(#47180,#47181),(#47182,#47183),
(#47184,#47185),(#47186,#47187),(#47188,#47189),(#47190,#47191),(#47192,
#47193),(#47194,#47195),(#47196,#47197),(#47198,#47199),(#47200,#47201),
(#47202,#47203),(#47204,#47205),(#47206,#47207),(#47208,#47209),(#47210,
#47211),(#47212,#47213),(#47214,#47215),(#47216,#47217),(#47218,#47219),
(#47220,#47221),(#47222,#47223),(#47224,#47225),(#47226,#47227),(#47228,
#47229),(#47230,#47231),(#47232,#47233),(#47234,#47235)),.UNSPECIFIED.,
 .F.,.F.,.F.)
B_SPLINE_SURFACE_WITH_KNOTS((6,1,1,1,1,1,1,1,1,1,1,1,1,1,1,1,1,1,1,1,1,
1,1,1,1,1,1,1,1,1,1,1,1,1,1,1,1,1,1,1,1,1,1,1,1,1,1,1,1,1,1,1,1,1,1,1,1,
1,1,1,1,1,1,1,1,6),(2,2),(-1.,-0.984615384615383,-0.969230769230768,-0.953846153846152,
-0.938461538461537,-0.923076923076922,-0.907692307692306,-0.892307692307691,
-0.876923076923076,-0.86153846153846,-0.846153846153845,-0.83076923076923,
-0.815384615384614,-0.799999999999999,-0.784615384615384,-0.769230769230768,
-0.753846153846153,-0.738461538461538,-0.723076923076922,-0.707692307692307,
-0.692307692307692,-0.676923076923076,-0.661538461538461,-0.646153846153846,
-0.63076923076923,-0.615384615384615,-0.6,-0.584615384615384,-0.569230769230769,
-0.553846153846154,-0.538461538461538,-0.523076923076923,-0.507692307692308,
-0.492307692307692,-0.476923076923077,-0.461538461538462,-0.446153846153846,
-0.430769230769231,-0.415384615384615,-0.4,-0.384615384615385,-0.369230769230769,
-0.353846153846154,-0.338461538461538,-0.323076923076923,-0.307692307692308,
-0.292307692307692,-0.276923076923077,-0.261538461538462,-0.246153846153846,
-0.230769230769231,-0.215384615384615,-0.2,-0.184615384615385,-0.169230769230769,
-0.153846153846154,-0.138461538461538,-0.123076923076923,-0.107692307692308,
-0.0923076923076923,-0.0769230769230769,-0.0615384615384615,-0.0461538461538462,
-0.0307692307692308,-0.0153846153846154,0.),(-1.,1.),.UNSPECIFIED.)
GEOMETRIC_REPRESENTATION_ITEM()
RATIONAL_B_SPLINE_SURFACE(((1.,1.),(1.,1.),(1.,1.),(1.,1.),(1.,1.),(1.,
1.),(1.,1.),(1.,1.),(1.,1.),(1.,1.),(1.,1.),(1.,1.),(1.,1.),(1.,1.),(1.,
1.),(1.,1.),(1.,1.),(1.,1.),(1.,1.),(1.,1.),(1.,1.),(1.,1.),(1.,1.),(1.,
1.),(1.,1.),(1.,1.),(1.,1.),(1.,1.),(1.,1.),(1.,1.),(1.,1.),(1.,1.),(1.,
1.),(1.,1.),(1.,1.),(1.,1.),(1.,1.),(1.,1.),(1.,1.),(1.,1.),(1.,1.),(1.,
1.),(1.,1.),(1.,1.),(1.,1.),(1.,1.),(1.,1.),(1.,1.),(1.,1.),(1.,1.),(1.,
1.),(1.,1.),(1.,1.),(1.,1.),(1.,1.),(1.,1.),(1.,1.),(1.,1.),(1.,1.),(1.,
1.),(1.,1.),(1.,1.),(1.,1.),(1.,1.),(1.,1.),(1.,1.),(1.,1.),(1.,1.),(1.,
1.),(1.,1.)))
REPRESENTATION_ITEM('')
SURFACE()
);
#82=(
BOUNDED_SURFACE()
B_SPLINE_SURFACE(5,1,((#47312,#47313),(#47314,#47315),(#47316,#47317),(#47318,
#47319),(#47320,#47321),(#47322,#47323),(#47324,#47325),(#47326,#47327),
(#47328,#47329),(#47330,#47331),(#47332,#47333),(#47334,#47335),(#47336,
#47337),(#47338,#47339),(#47340,#47341),(#47342,#47343),(#47344,#47345),
(#47346,#47347),(#47348,#47349),(#47350,#47351),(#47352,#47353),(#47354,
#47355),(#47356,#47357),(#47358,#47359),(#47360,#47361),(#47362,#47363),
(#47364,#47365),(#47366,#47367),(#47368,#47369),(#47370,#47371),(#47372,
#47373),(#47374,#47375),(#47376,#47377),(#47378,#47379),(#47380,#47381),
(#47382,#47383),(#47384,#47385),(#47386,#47387),(#47388,#47389),(#47390,
#47391),(#47392,#47393),(#47394,#47395),(#47396,#47397),(#47398,#47399),
(#47400,#47401),(#47402,#47403),(#47404,#47405),(#47406,#47407),(#47408,
#47409),(#47410,#47411),(#47412,#47413),(#47414,#47415),(#47416,#47417),
(#47418,#47419),(#47420,#47421),(#47422,#47423),(#47424,#47425),(#47426,
#47427),(#47428,#47429),(#47430,#47431),(#47432,#47433),(#47434,#47435),
(#47436,#47437),(#47438,#47439),(#47440,#47441),(#47442,#47443),(#47444,
#47445),(#47446,#47447),(#47448,#47449),(#47450,#47451)),.UNSPECIFIED.,
 .F.,.F.,.F.)
B_SPLINE_SURFACE_WITH_KNOTS((6,1,1,1,1,1,1,1,1,1,1,1,1,1,1,1,1,1,1,1,1,
1,1,1,1,1,1,1,1,1,1,1,1,1,1,1,1,1,1,1,1,1,1,1,1,1,1,1,1,1,1,1,1,1,1,1,1,
1,1,1,1,1,1,1,1,6),(2,2),(-1.,-0.984615384615383,-0.969230769230768,-0.953846153846152,
-0.938461538461537,-0.923076923076922,-0.907692307692306,-0.892307692307691,
-0.876923076923076,-0.86153846153846,-0.846153846153845,-0.83076923076923,
-0.815384615384614,-0.799999999999999,-0.784615384615384,-0.769230769230768,
-0.753846153846153,-0.738461538461538,-0.723076923076922,-0.707692307692307,
-0.692307692307692,-0.676923076923076,-0.661538461538461,-0.646153846153846,
-0.63076923076923,-0.615384615384615,-0.6,-0.584615384615384,-0.569230769230769,
-0.553846153846154,-0.538461538461538,-0.523076923076923,-0.507692307692308,
-0.492307692307692,-0.476923076923077,-0.461538461538462,-0.446153846153846,
-0.430769230769231,-0.415384615384615,-0.4,-0.384615384615385,-0.369230769230769,
-0.353846153846154,-0.338461538461538,-0.323076923076923,-0.307692307692308,
-0.292307692307692,-0.276923076923077,-0.261538461538462,-0.246153846153846,
-0.230769230769231,-0.215384615384615,-0.2,-0.184615384615385,-0.169230769230769,
-0.153846153846154,-0.138461538461538,-0.123076923076923,-0.107692307692308,
-0.0923076923076923,-0.0769230769230769,-0.0615384615384615,-0.0461538461538462,
-0.0307692307692308,-0.0153846153846154,0.),(-1.,1.),.UNSPECIFIED.)
GEOMETRIC_REPRESENTATION_ITEM()
RATIONAL_B_SPLINE_SURFACE(((1.,1.),(1.,1.),(1.,1.),(1.,1.),(1.,1.),(1.,
1.),(1.,1.),(1.,1.),(1.,1.),(1.,1.),(1.,1.),(1.,1.),(1.,1.),(1.,1.),(1.,
1.),(1.,1.),(1.,1.),(1.,1.),(1.,1.),(1.,1.),(1.,1.),(1.,1.),(1.,1.),(1.,
1.),(1.,1.),(1.,1.),(1.,1.),(1.,1.),(1.,1.),(1.,1.),(1.,1.),(1.,1.),(1.,
1.),(1.,1.),(1.,1.),(1.,1.),(1.,1.),(1.,1.),(1.,1.),(1.,1.),(1.,1.),(1.,
1.),(1.,1.),(1.,1.),(1.,1.),(1.,1.),(1.,1.),(1.,1.),(1.,1.),(1.,1.),(1.,
1.),(1.,1.),(1.,1.),(1.,1.),(1.,1.),(1.,1.),(1.,1.),(1.,1.),(1.,1.),(1.,
1.),(1.,1.),(1.,1.),(1.,1.),(1.,1.),(1.,1.),(1.,1.),(1.,1.),(1.,1.),(1.,
1.),(1.,1.)))
REPRESENTATION_ITEM('')
SURFACE()
);
#83=(
BOUNDED_SURFACE()
B_SPLINE_SURFACE(5,1,((#47528,#47529),(#47530,#47531),(#47532,#47533),(#47534,
#47535),(#47536,#47537),(#47538,#47539),(#47540,#47541),(#47542,#47543),
(#47544,#47545),(#47546,#47547),(#47548,#47549),(#47550,#47551),(#47552,
#47553),(#47554,#47555),(#47556,#47557),(#47558,#47559),(#47560,#47561),
(#47562,#47563),(#47564,#47565),(#47566,#47567),(#47568,#47569),(#47570,
#47571),(#47572,#47573),(#47574,#47575),(#47576,#47577),(#47578,#47579),
(#47580,#47581),(#47582,#47583),(#47584,#47585),(#47586,#47587),(#47588,
#47589),(#47590,#47591),(#47592,#47593),(#47594,#47595),(#47596,#47597),
(#47598,#47599),(#47600,#47601),(#47602,#47603),(#47604,#47605),(#47606,
#47607),(#47608,#47609),(#47610,#47611),(#47612,#47613),(#47614,#47615),
(#47616,#47617),(#47618,#47619),(#47620,#47621),(#47622,#47623),(#47624,
#47625),(#47626,#47627),(#47628,#47629),(#47630,#47631),(#47632,#47633),
(#47634,#47635),(#47636,#47637),(#47638,#47639),(#47640,#47641),(#47642,
#47643),(#47644,#47645),(#47646,#47647),(#47648,#47649),(#47650,#47651),
(#47652,#47653),(#47654,#47655),(#47656,#47657),(#47658,#47659),(#47660,
#47661),(#47662,#47663),(#47664,#47665),(#47666,#47667)),.UNSPECIFIED.,
 .F.,.F.,.F.)
B_SPLINE_SURFACE_WITH_KNOTS((6,1,1,1,1,1,1,1,1,1,1,1,1,1,1,1,1,1,1,1,1,
1,1,1,1,1,1,1,1,1,1,1,1,1,1,1,1,1,1,1,1,1,1,1,1,1,1,1,1,1,1,1,1,1,1,1,1,
1,1,1,1,1,1,1,1,6),(2,2),(-1.,-0.984615384615383,-0.969230769230768,-0.953846153846152,
-0.938461538461537,-0.923076923076922,-0.907692307692306,-0.892307692307691,
-0.876923076923076,-0.86153846153846,-0.846153846153845,-0.83076923076923,
-0.815384615384614,-0.799999999999999,-0.784615384615384,-0.769230769230768,
-0.753846153846153,-0.738461538461538,-0.723076923076922,-0.707692307692307,
-0.692307692307692,-0.676923076923076,-0.661538461538461,-0.646153846153846,
-0.63076923076923,-0.615384615384615,-0.6,-0.584615384615384,-0.569230769230769,
-0.553846153846154,-0.538461538461538,-0.523076923076923,-0.507692307692308,
-0.492307692307692,-0.476923076923077,-0.461538461538462,-0.446153846153846,
-0.430769230769231,-0.415384615384615,-0.4,-0.384615384615385,-0.369230769230769,
-0.353846153846154,-0.338461538461538,-0.323076923076923,-0.307692307692308,
-0.292307692307692,-0.276923076923077,-0.261538461538462,-0.246153846153846,
-0.230769230769231,-0.215384615384615,-0.2,-0.184615384615385,-0.169230769230769,
-0.153846153846154,-0.138461538461538,-0.123076923076923,-0.107692307692308,
-0.0923076923076923,-0.0769230769230769,-0.0615384615384615,-0.0461538461538462,
-0.0307692307692308,-0.0153846153846154,0.),(-1.,1.),.UNSPECIFIED.)
GEOMETRIC_REPRESENTATION_ITEM()
RATIONAL_B_SPLINE_SURFACE(((1.,1.),(1.,1.),(1.,1.),(1.,1.),(1.,1.),(1.,
1.),(1.,1.),(1.,1.),(1.,1.),(1.,1.),(1.,1.),(1.,1.),(1.,1.),(1.,1.),(1.,
1.),(1.,1.),(1.,1.),(1.,1.),(1.,1.),(1.,1.),(1.,1.),(1.,1.),(1.,1.),(1.,
1.),(1.,1.),(1.,1.),(1.,1.),(1.,1.),(1.,1.),(1.,1.),(1.,1.),(1.,1.),(1.,
1.),(1.,1.),(1.,1.),(1.,1.),(1.,1.),(1.,1.),(1.,1.),(1.,1.),(1.,1.),(1.,
1.),(1.,1.),(1.,1.),(1.,1.),(1.,1.),(1.,1.),(1.,1.),(1.,1.),(1.,1.),(1.,
1.),(1.,1.),(1.,1.),(1.,1.),(1.,1.),(1.,1.),(1.,1.),(1.,1.),(1.,1.),(1.,
1.),(1.,1.),(1.,1.),(1.,1.),(1.,1.),(1.,1.),(1.,1.),(1.,1.),(1.,1.),(1.,
1.),(1.,1.)))
REPRESENTATION_ITEM('')
SURFACE()
);
#84=(
BOUNDED_SURFACE()
B_SPLINE_SURFACE(5,1,((#47744,#47745),(#47746,#47747),(#47748,#47749),(#47750,
#47751),(#47752,#47753),(#47754,#47755),(#47756,#47757),(#47758,#47759),
(#47760,#47761),(#47762,#47763),(#47764,#47765),(#47766,#47767),(#47768,
#47769),(#47770,#47771),(#47772,#47773),(#47774,#47775),(#47776,#47777),
(#47778,#47779),(#47780,#47781),(#47782,#47783),(#47784,#47785),(#47786,
#47787),(#47788,#47789),(#47790,#47791),(#47792,#47793),(#47794,#47795),
(#47796,#47797),(#47798,#47799),(#47800,#47801),(#47802,#47803),(#47804,
#47805),(#47806,#47807),(#47808,#47809),(#47810,#47811),(#47812,#47813),
(#47814,#47815),(#47816,#47817),(#47818,#47819),(#47820,#47821),(#47822,
#47823),(#47824,#47825),(#47826,#47827),(#47828,#47829),(#47830,#47831),
(#47832,#47833),(#47834,#47835),(#47836,#47837),(#47838,#47839),(#47840,
#47841),(#47842,#47843),(#47844,#47845),(#47846,#47847),(#47848,#47849),
(#47850,#47851),(#47852,#47853),(#47854,#47855),(#47856,#47857),(#47858,
#47859),(#47860,#47861),(#47862,#47863),(#47864,#47865),(#47866,#47867),
(#47868,#47869),(#47870,#47871),(#47872,#47873),(#47874,#47875),(#47876,
#47877),(#47878,#47879),(#47880,#47881),(#47882,#47883)),.UNSPECIFIED.,
 .F.,.F.,.F.)
B_SPLINE_SURFACE_WITH_KNOTS((6,1,1,1,1,1,1,1,1,1,1,1,1,1,1,1,1,1,1,1,1,
1,1,1,1,1,1,1,1,1,1,1,1,1,1,1,1,1,1,1,1,1,1,1,1,1,1,1,1,1,1,1,1,1,1,1,1,
1,1,1,1,1,1,1,1,6),(2,2),(-1.,-0.984615384615383,-0.969230769230768,-0.953846153846152,
-0.938461538461537,-0.923076923076922,-0.907692307692306,-0.892307692307691,
-0.876923076923076,-0.86153846153846,-0.846153846153845,-0.83076923076923,
-0.815384615384614,-0.799999999999999,-0.784615384615384,-0.769230769230768,
-0.753846153846153,-0.738461538461538,-0.723076923076922,-0.707692307692307,
-0.692307692307692,-0.676923076923076,-0.661538461538461,-0.646153846153846,
-0.63076923076923,-0.615384615384615,-0.6,-0.584615384615384,-0.569230769230769,
-0.553846153846154,-0.538461538461538,-0.523076923076923,-0.507692307692308,
-0.492307692307692,-0.476923076923077,-0.461538461538462,-0.446153846153846,
-0.430769230769231,-0.415384615384615,-0.4,-0.384615384615385,-0.369230769230769,
-0.353846153846154,-0.338461538461538,-0.323076923076923,-0.307692307692308,
-0.292307692307692,-0.276923076923077,-0.261538461538462,-0.246153846153846,
-0.230769230769231,-0.215384615384615,-0.2,-0.184615384615385,-0.169230769230769,
-0.153846153846154,-0.138461538461538,-0.123076923076923,-0.107692307692308,
-0.0923076923076923,-0.0769230769230769,-0.0615384615384615,-0.0461538461538462,
-0.0307692307692308,-0.0153846153846154,0.),(-1.,1.),.UNSPECIFIED.)
GEOMETRIC_REPRESENTATION_ITEM()
RATIONAL_B_SPLINE_SURFACE(((1.,1.),(1.,1.),(1.,1.),(1.,1.),(1.,1.),(1.,
1.),(1.,1.),(1.,1.),(1.,1.),(1.,1.),(1.,1.),(1.,1.),(1.,1.),(1.,1.),(1.,
1.),(1.,1.),(1.,1.),(1.,1.),(1.,1.),(1.,1.),(1.,1.),(1.,1.),(1.,1.),(1.,
1.),(1.,1.),(1.,1.),(1.,1.),(1.,1.),(1.,1.),(1.,1.),(1.,1.),(1.,1.),(1.,
1.),(1.,1.),(1.,1.),(1.,1.),(1.,1.),(1.,1.),(1.,1.),(1.,1.),(1.,1.),(1.,
1.),(1.,1.),(1.,1.),(1.,1.),(1.,1.),(1.,1.),(1.,1.),(1.,1.),(1.,1.),(1.,
1.),(1.,1.),(1.,1.),(1.,1.),(1.,1.),(1.,1.),(1.,1.),(1.,1.),(1.,1.),(1.,
1.),(1.,1.),(1.,1.),(1.,1.),(1.,1.),(1.,1.),(1.,1.),(1.,1.),(1.,1.),(1.,
1.),(1.,1.)))
REPRESENTATION_ITEM('')
SURFACE()
);
#85=(
BOUNDED_SURFACE()
B_SPLINE_SURFACE(5,1,((#47960,#47961),(#47962,#47963),(#47964,#47965),(#47966,
#47967),(#47968,#47969),(#47970,#47971),(#47972,#47973),(#47974,#47975),
(#47976,#47977),(#47978,#47979),(#47980,#47981),(#47982,#47983),(#47984,
#47985),(#47986,#47987),(#47988,#47989),(#47990,#47991),(#47992,#47993),
(#47994,#47995),(#47996,#47997),(#47998,#47999),(#48000,#48001),(#48002,
#48003),(#48004,#48005),(#48006,#48007),(#48008,#48009),(#48010,#48011),
(#48012,#48013),(#48014,#48015),(#48016,#48017),(#48018,#48019),(#48020,
#48021),(#48022,#48023),(#48024,#48025),(#48026,#48027),(#48028,#48029),
(#48030,#48031),(#48032,#48033),(#48034,#48035),(#48036,#48037),(#48038,
#48039),(#48040,#48041),(#48042,#48043),(#48044,#48045),(#48046,#48047),
(#48048,#48049),(#48050,#48051),(#48052,#48053),(#48054,#48055),(#48056,
#48057),(#48058,#48059),(#48060,#48061),(#48062,#48063),(#48064,#48065),
(#48066,#48067),(#48068,#48069),(#48070,#48071),(#48072,#48073),(#48074,
#48075),(#48076,#48077),(#48078,#48079),(#48080,#48081),(#48082,#48083),
(#48084,#48085),(#48086,#48087),(#48088,#48089),(#48090,#48091),(#48092,
#48093),(#48094,#48095),(#48096,#48097),(#48098,#48099)),.UNSPECIFIED.,
 .F.,.F.,.F.)
B_SPLINE_SURFACE_WITH_KNOTS((6,1,1,1,1,1,1,1,1,1,1,1,1,1,1,1,1,1,1,1,1,
1,1,1,1,1,1,1,1,1,1,1,1,1,1,1,1,1,1,1,1,1,1,1,1,1,1,1,1,1,1,1,1,1,1,1,1,
1,1,1,1,1,1,1,1,6),(2,2),(-1.,-0.984615384615383,-0.969230769230768,-0.953846153846152,
-0.938461538461537,-0.923076923076922,-0.907692307692306,-0.892307692307691,
-0.876923076923076,-0.86153846153846,-0.846153846153845,-0.83076923076923,
-0.815384615384614,-0.799999999999999,-0.784615384615384,-0.769230769230768,
-0.753846153846153,-0.738461538461538,-0.723076923076922,-0.707692307692307,
-0.692307692307692,-0.676923076923076,-0.661538461538461,-0.646153846153846,
-0.63076923076923,-0.615384615384615,-0.6,-0.584615384615384,-0.569230769230769,
-0.553846153846154,-0.538461538461538,-0.523076923076923,-0.507692307692308,
-0.492307692307692,-0.476923076923077,-0.461538461538462,-0.446153846153846,
-0.430769230769231,-0.415384615384615,-0.4,-0.384615384615385,-0.369230769230769,
-0.353846153846154,-0.338461538461538,-0.323076923076923,-0.307692307692308,
-0.292307692307692,-0.276923076923077,-0.261538461538462,-0.246153846153846,
-0.230769230769231,-0.215384615384615,-0.2,-0.184615384615385,-0.169230769230769,
-0.153846153846154,-0.138461538461538,-0.123076923076923,-0.107692307692308,
-0.0923076923076923,-0.0769230769230769,-0.0615384615384615,-0.0461538461538462,
-0.0307692307692308,-0.0153846153846154,0.),(-1.,1.),.UNSPECIFIED.)
GEOMETRIC_REPRESENTATION_ITEM()
RATIONAL_B_SPLINE_SURFACE(((1.,1.),(1.,1.),(1.,1.),(1.,1.),(1.,1.),(1.,
1.),(1.,1.),(1.,1.),(1.,1.),(1.,1.),(1.,1.),(1.,1.),(1.,1.),(1.,1.),(1.,
1.),(1.,1.),(1.,1.),(1.,1.),(1.,1.),(1.,1.),(1.,1.),(1.,1.),(1.,1.),(1.,
1.),(1.,1.),(1.,1.),(1.,1.),(1.,1.),(1.,1.),(1.,1.),(1.,1.),(1.,1.),(1.,
1.),(1.,1.),(1.,1.),(1.,1.),(1.,1.),(1.,1.),(1.,1.),(1.,1.),(1.,1.),(1.,
1.),(1.,1.),(1.,1.),(1.,1.),(1.,1.),(1.,1.),(1.,1.),(1.,1.),(1.,1.),(1.,
1.),(1.,1.),(1.,1.),(1.,1.),(1.,1.),(1.,1.),(1.,1.),(1.,1.),(1.,1.),(1.,
1.),(1.,1.),(1.,1.),(1.,1.),(1.,1.),(1.,1.),(1.,1.),(1.,1.),(1.,1.),(1.,
1.),(1.,1.)))
REPRESENTATION_ITEM('')
SURFACE()
);
#86=(
BOUNDED_SURFACE()
B_SPLINE_SURFACE(5,1,((#48176,#48177),(#48178,#48179),(#48180,#48181),(#48182,
#48183),(#48184,#48185),(#48186,#48187),(#48188,#48189),(#48190,#48191),
(#48192,#48193),(#48194,#48195),(#48196,#48197),(#48198,#48199),(#48200,
#48201),(#48202,#48203),(#48204,#48205),(#48206,#48207),(#48208,#48209),
(#48210,#48211),(#48212,#48213),(#48214,#48215),(#48216,#48217),(#48218,
#48219),(#48220,#48221),(#48222,#48223),(#48224,#48225),(#48226,#48227),
(#48228,#48229),(#48230,#48231),(#48232,#48233),(#48234,#48235),(#48236,
#48237),(#48238,#48239),(#48240,#48241),(#48242,#48243),(#48244,#48245),
(#48246,#48247),(#48248,#48249),(#48250,#48251),(#48252,#48253),(#48254,
#48255),(#48256,#48257),(#48258,#48259),(#48260,#48261),(#48262,#48263),
(#48264,#48265),(#48266,#48267),(#48268,#48269),(#48270,#48271),(#48272,
#48273),(#48274,#48275),(#48276,#48277),(#48278,#48279),(#48280,#48281),
(#48282,#48283),(#48284,#48285),(#48286,#48287),(#48288,#48289),(#48290,
#48291),(#48292,#48293),(#48294,#48295),(#48296,#48297),(#48298,#48299),
(#48300,#48301),(#48302,#48303),(#48304,#48305),(#48306,#48307),(#48308,
#48309),(#48310,#48311),(#48312,#48313),(#48314,#48315)),.UNSPECIFIED.,
 .F.,.F.,.F.)
B_SPLINE_SURFACE_WITH_KNOTS((6,1,1,1,1,1,1,1,1,1,1,1,1,1,1,1,1,1,1,1,1,
1,1,1,1,1,1,1,1,1,1,1,1,1,1,1,1,1,1,1,1,1,1,1,1,1,1,1,1,1,1,1,1,1,1,1,1,
1,1,1,1,1,1,1,1,6),(2,2),(-1.,-0.984615384615383,-0.969230769230768,-0.953846153846152,
-0.938461538461537,-0.923076923076922,-0.907692307692306,-0.892307692307691,
-0.876923076923076,-0.86153846153846,-0.846153846153845,-0.83076923076923,
-0.815384615384614,-0.799999999999999,-0.784615384615384,-0.769230769230768,
-0.753846153846153,-0.738461538461538,-0.723076923076922,-0.707692307692307,
-0.692307692307692,-0.676923076923076,-0.661538461538461,-0.646153846153846,
-0.63076923076923,-0.615384615384615,-0.6,-0.584615384615384,-0.569230769230769,
-0.553846153846154,-0.538461538461538,-0.523076923076923,-0.507692307692308,
-0.492307692307692,-0.476923076923077,-0.461538461538462,-0.446153846153846,
-0.430769230769231,-0.415384615384615,-0.4,-0.384615384615385,-0.369230769230769,
-0.353846153846154,-0.338461538461538,-0.323076923076923,-0.307692307692308,
-0.292307692307692,-0.276923076923077,-0.261538461538462,-0.246153846153846,
-0.230769230769231,-0.215384615384615,-0.2,-0.184615384615385,-0.169230769230769,
-0.153846153846154,-0.138461538461538,-0.123076923076923,-0.107692307692308,
-0.0923076923076923,-0.0769230769230769,-0.0615384615384615,-0.0461538461538462,
-0.0307692307692308,-0.0153846153846154,0.),(-1.,1.),.UNSPECIFIED.)
GEOMETRIC_REPRESENTATION_ITEM()
RATIONAL_B_SPLINE_SURFACE(((1.,1.),(1.,1.),(1.,1.),(1.,1.),(1.,1.),(1.,
1.),(1.,1.),(1.,1.),(1.,1.),(1.,1.),(1.,1.),(1.,1.),(1.,1.),(1.,1.),(1.,
1.),(1.,1.),(1.,1.),(1.,1.),(1.,1.),(1.,1.),(1.,1.),(1.,1.),(1.,1.),(1.,
1.),(1.,1.),(1.,1.),(1.,1.),(1.,1.),(1.,1.),(1.,1.),(1.,1.),(1.,1.),(1.,
1.),(1.,1.),(1.,1.),(1.,1.),(1.,1.),(1.,1.),(1.,1.),(1.,1.),(1.,1.),(1.,
1.),(1.,1.),(1.,1.),(1.,1.),(1.,1.),(1.,1.),(1.,1.),(1.,1.),(1.,1.),(1.,
1.),(1.,1.),(1.,1.),(1.,1.),(1.,1.),(1.,1.),(1.,1.),(1.,1.),(1.,1.),(1.,
1.),(1.,1.),(1.,1.),(1.,1.),(1.,1.),(1.,1.),(1.,1.),(1.,1.),(1.,1.),(1.,
1.),(1.,1.)))
REPRESENTATION_ITEM('')
SURFACE()
);
#87=(
BOUNDED_SURFACE()
B_SPLINE_SURFACE(5,1,((#48392,#48393),(#48394,#48395),(#48396,#48397),(#48398,
#48399),(#48400,#48401),(#48402,#48403),(#48404,#48405),(#48406,#48407),
(#48408,#48409),(#48410,#48411),(#48412,#48413),(#48414,#48415),(#48416,
#48417),(#48418,#48419),(#48420,#48421),(#48422,#48423),(#48424,#48425),
(#48426,#48427),(#48428,#48429),(#48430,#48431),(#48432,#48433),(#48434,
#48435),(#48436,#48437),(#48438,#48439),(#48440,#48441),(#48442,#48443),
(#48444,#48445),(#48446,#48447),(#48448,#48449),(#48450,#48451),(#48452,
#48453),(#48454,#48455),(#48456,#48457),(#48458,#48459),(#48460,#48461),
(#48462,#48463),(#48464,#48465),(#48466,#48467),(#48468,#48469),(#48470,
#48471),(#48472,#48473),(#48474,#48475),(#48476,#48477),(#48478,#48479),
(#48480,#48481),(#48482,#48483),(#48484,#48485),(#48486,#48487),(#48488,
#48489),(#48490,#48491),(#48492,#48493),(#48494,#48495),(#48496,#48497),
(#48498,#48499),(#48500,#48501),(#48502,#48503),(#48504,#48505),(#48506,
#48507),(#48508,#48509),(#48510,#48511),(#48512,#48513),(#48514,#48515),
(#48516,#48517),(#48518,#48519),(#48520,#48521),(#48522,#48523),(#48524,
#48525),(#48526,#48527),(#48528,#48529),(#48530,#48531)),.UNSPECIFIED.,
 .F.,.F.,.F.)
B_SPLINE_SURFACE_WITH_KNOTS((6,1,1,1,1,1,1,1,1,1,1,1,1,1,1,1,1,1,1,1,1,
1,1,1,1,1,1,1,1,1,1,1,1,1,1,1,1,1,1,1,1,1,1,1,1,1,1,1,1,1,1,1,1,1,1,1,1,
1,1,1,1,1,1,1,1,6),(2,2),(-1.,-0.984615384615383,-0.969230769230768,-0.953846153846152,
-0.938461538461537,-0.923076923076922,-0.907692307692306,-0.892307692307691,
-0.876923076923076,-0.86153846153846,-0.846153846153845,-0.83076923076923,
-0.815384615384614,-0.799999999999999,-0.784615384615384,-0.769230769230768,
-0.753846153846153,-0.738461538461538,-0.723076923076922,-0.707692307692307,
-0.692307692307692,-0.676923076923076,-0.661538461538461,-0.646153846153846,
-0.63076923076923,-0.615384615384615,-0.6,-0.584615384615384,-0.569230769230769,
-0.553846153846154,-0.538461538461538,-0.523076923076923,-0.507692307692308,
-0.492307692307692,-0.476923076923077,-0.461538461538462,-0.446153846153846,
-0.430769230769231,-0.415384615384615,-0.4,-0.384615384615385,-0.369230769230769,
-0.353846153846154,-0.338461538461538,-0.323076923076923,-0.307692307692308,
-0.292307692307692,-0.276923076923077,-0.261538461538462,-0.246153846153846,
-0.230769230769231,-0.215384615384615,-0.2,-0.184615384615385,-0.169230769230769,
-0.153846153846154,-0.138461538461538,-0.123076923076923,-0.107692307692308,
-0.0923076923076923,-0.0769230769230769,-0.0615384615384615,-0.0461538461538462,
-0.0307692307692308,-0.0153846153846154,0.),(-1.,1.),.UNSPECIFIED.)
GEOMETRIC_REPRESENTATION_ITEM()
RATIONAL_B_SPLINE_SURFACE(((1.,1.),(1.,1.),(1.,1.),(1.,1.),(1.,1.),(1.,
1.),(1.,1.),(1.,1.),(1.,1.),(1.,1.),(1.,1.),(1.,1.),(1.,1.),(1.,1.),(1.,
1.),(1.,1.),(1.,1.),(1.,1.),(1.,1.),(1.,1.),(1.,1.),(1.,1.),(1.,1.),(1.,
1.),(1.,1.),(1.,1.),(1.,1.),(1.,1.),(1.,1.),(1.,1.),(1.,1.),(1.,1.),(1.,
1.),(1.,1.),(1.,1.),(1.,1.),(1.,1.),(1.,1.),(1.,1.),(1.,1.),(1.,1.),(1.,
1.),(1.,1.),(1.,1.),(1.,1.),(1.,1.),(1.,1.),(1.,1.),(1.,1.),(1.,1.),(1.,
1.),(1.,1.),(1.,1.),(1.,1.),(1.,1.),(1.,1.),(1.,1.),(1.,1.),(1.,1.),(1.,
1.),(1.,1.),(1.,1.),(1.,1.),(1.,1.),(1.,1.),(1.,1.),(1.,1.),(1.,1.),(1.,
1.),(1.,1.)))
REPRESENTATION_ITEM('')
SURFACE()
);
#88=(
BOUNDED_SURFACE()
B_SPLINE_SURFACE(5,1,((#48608,#48609),(#48610,#48611),(#48612,#48613),(#48614,
#48615),(#48616,#48617),(#48618,#48619),(#48620,#48621),(#48622,#48623),
(#48624,#48625),(#48626,#48627),(#48628,#48629),(#48630,#48631),(#48632,
#48633),(#48634,#48635),(#48636,#48637),(#48638,#48639),(#48640,#48641),
(#48642,#48643),(#48644,#48645),(#48646,#48647),(#48648,#48649),(#48650,
#48651),(#48652,#48653),(#48654,#48655),(#48656,#48657),(#48658,#48659),
(#48660,#48661),(#48662,#48663),(#48664,#48665),(#48666,#48667),(#48668,
#48669),(#48670,#48671),(#48672,#48673),(#48674,#48675),(#48676,#48677),
(#48678,#48679),(#48680,#48681),(#48682,#48683),(#48684,#48685),(#48686,
#48687),(#48688,#48689),(#48690,#48691),(#48692,#48693),(#48694,#48695),
(#48696,#48697),(#48698,#48699),(#48700,#48701),(#48702,#48703),(#48704,
#48705),(#48706,#48707),(#48708,#48709),(#48710,#48711),(#48712,#48713),
(#48714,#48715),(#48716,#48717),(#48718,#48719),(#48720,#48721),(#48722,
#48723),(#48724,#48725),(#48726,#48727),(#48728,#48729),(#48730,#48731),
(#48732,#48733),(#48734,#48735),(#48736,#48737),(#48738,#48739),(#48740,
#48741),(#48742,#48743),(#48744,#48745),(#48746,#48747)),.UNSPECIFIED.,
 .F.,.F.,.F.)
B_SPLINE_SURFACE_WITH_KNOTS((6,1,1,1,1,1,1,1,1,1,1,1,1,1,1,1,1,1,1,1,1,
1,1,1,1,1,1,1,1,1,1,1,1,1,1,1,1,1,1,1,1,1,1,1,1,1,1,1,1,1,1,1,1,1,1,1,1,
1,1,1,1,1,1,1,1,6),(2,2),(-1.,-0.984615384615383,-0.969230769230768,-0.953846153846152,
-0.938461538461537,-0.923076923076922,-0.907692307692306,-0.892307692307691,
-0.876923076923076,-0.86153846153846,-0.846153846153845,-0.83076923076923,
-0.815384615384614,-0.799999999999999,-0.784615384615384,-0.769230769230768,
-0.753846153846153,-0.738461538461538,-0.723076923076922,-0.707692307692307,
-0.692307692307692,-0.676923076923076,-0.661538461538461,-0.646153846153846,
-0.63076923076923,-0.615384615384615,-0.6,-0.584615384615384,-0.569230769230769,
-0.553846153846154,-0.538461538461538,-0.523076923076923,-0.507692307692308,
-0.492307692307692,-0.476923076923077,-0.461538461538462,-0.446153846153846,
-0.430769230769231,-0.415384615384615,-0.4,-0.384615384615385,-0.369230769230769,
-0.353846153846154,-0.338461538461538,-0.323076923076923,-0.307692307692308,
-0.292307692307692,-0.276923076923077,-0.261538461538462,-0.246153846153846,
-0.230769230769231,-0.215384615384615,-0.2,-0.184615384615385,-0.169230769230769,
-0.153846153846154,-0.138461538461538,-0.123076923076923,-0.107692307692308,
-0.0923076923076923,-0.0769230769230769,-0.0615384615384615,-0.0461538461538462,
-0.0307692307692308,-0.0153846153846154,0.),(-1.,1.),.UNSPECIFIED.)
GEOMETRIC_REPRESENTATION_ITEM()
RATIONAL_B_SPLINE_SURFACE(((1.,1.),(1.,1.),(1.,1.),(1.,1.),(1.,1.),(1.,
1.),(1.,1.),(1.,1.),(1.,1.),(1.,1.),(1.,1.),(1.,1.),(1.,1.),(1.,1.),(1.,
1.),(1.,1.),(1.,1.),(1.,1.),(1.,1.),(1.,1.),(1.,1.),(1.,1.),(1.,1.),(1.,
1.),(1.,1.),(1.,1.),(1.,1.),(1.,1.),(1.,1.),(1.,1.),(1.,1.),(1.,1.),(1.,
1.),(1.,1.),(1.,1.),(1.,1.),(1.,1.),(1.,1.),(1.,1.),(1.,1.),(1.,1.),(1.,
1.),(1.,1.),(1.,1.),(1.,1.),(1.,1.),(1.,1.),(1.,1.),(1.,1.),(1.,1.),(1.,
1.),(1.,1.),(1.,1.),(1.,1.),(1.,1.),(1.,1.),(1.,1.),(1.,1.),(1.,1.),(1.,
1.),(1.,1.),(1.,1.),(1.,1.),(1.,1.),(1.,1.),(1.,1.),(1.,1.),(1.,1.),(1.,
1.),(1.,1.)))
REPRESENTATION_ITEM('')
SURFACE()
);
#89=(
BOUNDED_SURFACE()
B_SPLINE_SURFACE(5,1,((#48824,#48825),(#48826,#48827),(#48828,#48829),(#48830,
#48831),(#48832,#48833),(#48834,#48835),(#48836,#48837),(#48838,#48839),
(#48840,#48841),(#48842,#48843),(#48844,#48845),(#48846,#48847),(#48848,
#48849),(#48850,#48851),(#48852,#48853),(#48854,#48855),(#48856,#48857),
(#48858,#48859),(#48860,#48861),(#48862,#48863),(#48864,#48865),(#48866,
#48867),(#48868,#48869),(#48870,#48871),(#48872,#48873),(#48874,#48875),
(#48876,#48877),(#48878,#48879),(#48880,#48881),(#48882,#48883),(#48884,
#48885),(#48886,#48887),(#48888,#48889),(#48890,#48891),(#48892,#48893),
(#48894,#48895),(#48896,#48897),(#48898,#48899),(#48900,#48901),(#48902,
#48903),(#48904,#48905),(#48906,#48907),(#48908,#48909),(#48910,#48911),
(#48912,#48913),(#48914,#48915),(#48916,#48917),(#48918,#48919),(#48920,
#48921),(#48922,#48923),(#48924,#48925),(#48926,#48927),(#48928,#48929),
(#48930,#48931),(#48932,#48933),(#48934,#48935),(#48936,#48937),(#48938,
#48939),(#48940,#48941),(#48942,#48943),(#48944,#48945),(#48946,#48947),
(#48948,#48949),(#48950,#48951),(#48952,#48953),(#48954,#48955),(#48956,
#48957),(#48958,#48959),(#48960,#48961),(#48962,#48963)),.UNSPECIFIED.,
 .F.,.F.,.F.)
B_SPLINE_SURFACE_WITH_KNOTS((6,1,1,1,1,1,1,1,1,1,1,1,1,1,1,1,1,1,1,1,1,
1,1,1,1,1,1,1,1,1,1,1,1,1,1,1,1,1,1,1,1,1,1,1,1,1,1,1,1,1,1,1,1,1,1,1,1,
1,1,1,1,1,1,1,1,6),(2,2),(-1.,-0.984615384615383,-0.969230769230768,-0.953846153846152,
-0.938461538461537,-0.923076923076922,-0.907692307692306,-0.892307692307691,
-0.876923076923076,-0.86153846153846,-0.846153846153845,-0.83076923076923,
-0.815384615384614,-0.799999999999999,-0.784615384615384,-0.769230769230768,
-0.753846153846153,-0.738461538461538,-0.723076923076922,-0.707692307692307,
-0.692307692307692,-0.676923076923076,-0.661538461538461,-0.646153846153846,
-0.63076923076923,-0.615384615384615,-0.6,-0.584615384615384,-0.569230769230769,
-0.553846153846154,-0.538461538461538,-0.523076923076923,-0.507692307692308,
-0.492307692307692,-0.476923076923077,-0.461538461538462,-0.446153846153846,
-0.430769230769231,-0.415384615384615,-0.4,-0.384615384615385,-0.369230769230769,
-0.353846153846154,-0.338461538461538,-0.323076923076923,-0.307692307692308,
-0.292307692307692,-0.276923076923077,-0.261538461538462,-0.246153846153846,
-0.230769230769231,-0.215384615384615,-0.2,-0.184615384615385,-0.169230769230769,
-0.153846153846154,-0.138461538461538,-0.123076923076923,-0.107692307692308,
-0.0923076923076923,-0.0769230769230769,-0.0615384615384615,-0.0461538461538462,
-0.0307692307692308,-0.0153846153846154,0.),(-1.,1.),.UNSPECIFIED.)
GEOMETRIC_REPRESENTATION_ITEM()
RATIONAL_B_SPLINE_SURFACE(((1.,1.),(1.,1.),(1.,1.),(1.,1.),(1.,1.),(1.,
1.),(1.,1.),(1.,1.),(1.,1.),(1.,1.),(1.,1.),(1.,1.),(1.,1.),(1.,1.),(1.,
1.),(1.,1.),(1.,1.),(1.,1.),(1.,1.),(1.,1.),(1.,1.),(1.,1.),(1.,1.),(1.,
1.),(1.,1.),(1.,1.),(1.,1.),(1.,1.),(1.,1.),(1.,1.),(1.,1.),(1.,1.),(1.,
1.),(1.,1.),(1.,1.),(1.,1.),(1.,1.),(1.,1.),(1.,1.),(1.,1.),(1.,1.),(1.,
1.),(1.,1.),(1.,1.),(1.,1.),(1.,1.),(1.,1.),(1.,1.),(1.,1.),(1.,1.),(1.,
1.),(1.,1.),(1.,1.),(1.,1.),(1.,1.),(1.,1.),(1.,1.),(1.,1.),(1.,1.),(1.,
1.),(1.,1.),(1.,1.),(1.,1.),(1.,1.),(1.,1.),(1.,1.),(1.,1.),(1.,1.),(1.,
1.),(1.,1.)))
REPRESENTATION_ITEM('')
SURFACE()
);
#90=(
BOUNDED_SURFACE()
B_SPLINE_SURFACE(5,1,((#49040,#49041),(#49042,#49043),(#49044,#49045),(#49046,
#49047),(#49048,#49049),(#49050,#49051),(#49052,#49053),(#49054,#49055),
(#49056,#49057),(#49058,#49059),(#49060,#49061),(#49062,#49063),(#49064,
#49065),(#49066,#49067),(#49068,#49069),(#49070,#49071),(#49072,#49073),
(#49074,#49075),(#49076,#49077),(#49078,#49079),(#49080,#49081),(#49082,
#49083),(#49084,#49085),(#49086,#49087),(#49088,#49089),(#49090,#49091),
(#49092,#49093),(#49094,#49095),(#49096,#49097),(#49098,#49099),(#49100,
#49101),(#49102,#49103),(#49104,#49105),(#49106,#49107),(#49108,#49109),
(#49110,#49111),(#49112,#49113),(#49114,#49115),(#49116,#49117),(#49118,
#49119),(#49120,#49121),(#49122,#49123),(#49124,#49125),(#49126,#49127),
(#49128,#49129),(#49130,#49131),(#49132,#49133),(#49134,#49135),(#49136,
#49137),(#49138,#49139),(#49140,#49141),(#49142,#49143),(#49144,#49145),
(#49146,#49147),(#49148,#49149),(#49150,#49151),(#49152,#49153),(#49154,
#49155),(#49156,#49157),(#49158,#49159),(#49160,#49161),(#49162,#49163),
(#49164,#49165),(#49166,#49167),(#49168,#49169),(#49170,#49171),(#49172,
#49173),(#49174,#49175),(#49176,#49177),(#49178,#49179)),.UNSPECIFIED.,
 .F.,.F.,.F.)
B_SPLINE_SURFACE_WITH_KNOTS((6,1,1,1,1,1,1,1,1,1,1,1,1,1,1,1,1,1,1,1,1,
1,1,1,1,1,1,1,1,1,1,1,1,1,1,1,1,1,1,1,1,1,1,1,1,1,1,1,1,1,1,1,1,1,1,1,1,
1,1,1,1,1,1,1,1,6),(2,2),(-1.,-0.984615384615383,-0.969230769230768,-0.953846153846152,
-0.938461538461537,-0.923076923076922,-0.907692307692306,-0.892307692307691,
-0.876923076923076,-0.86153846153846,-0.846153846153845,-0.83076923076923,
-0.815384615384614,-0.799999999999999,-0.784615384615384,-0.769230769230768,
-0.753846153846153,-0.738461538461538,-0.723076923076922,-0.707692307692307,
-0.692307692307692,-0.676923076923076,-0.661538461538461,-0.646153846153846,
-0.63076923076923,-0.615384615384615,-0.6,-0.584615384615384,-0.569230769230769,
-0.553846153846154,-0.538461538461538,-0.523076923076923,-0.507692307692308,
-0.492307692307692,-0.476923076923077,-0.461538461538462,-0.446153846153846,
-0.430769230769231,-0.415384615384615,-0.4,-0.384615384615385,-0.369230769230769,
-0.353846153846154,-0.338461538461538,-0.323076923076923,-0.307692307692308,
-0.292307692307692,-0.276923076923077,-0.261538461538462,-0.246153846153846,
-0.230769230769231,-0.215384615384615,-0.2,-0.184615384615385,-0.169230769230769,
-0.153846153846154,-0.138461538461538,-0.123076923076923,-0.107692307692308,
-0.0923076923076923,-0.0769230769230769,-0.0615384615384615,-0.0461538461538462,
-0.0307692307692308,-0.0153846153846154,0.),(-1.,1.),.UNSPECIFIED.)
GEOMETRIC_REPRESENTATION_ITEM()
RATIONAL_B_SPLINE_SURFACE(((1.,1.),(1.,1.),(1.,1.),(1.,1.),(1.,1.),(1.,
1.),(1.,1.),(1.,1.),(1.,1.),(1.,1.),(1.,1.),(1.,1.),(1.,1.),(1.,1.),(1.,
1.),(1.,1.),(1.,1.),(1.,1.),(1.,1.),(1.,1.),(1.,1.),(1.,1.),(1.,1.),(1.,
1.),(1.,1.),(1.,1.),(1.,1.),(1.,1.),(1.,1.),(1.,1.),(1.,1.),(1.,1.),(1.,
1.),(1.,1.),(1.,1.),(1.,1.),(1.,1.),(1.,1.),(1.,1.),(1.,1.),(1.,1.),(1.,
1.),(1.,1.),(1.,1.),(1.,1.),(1.,1.),(1.,1.),(1.,1.),(1.,1.),(1.,1.),(1.,
1.),(1.,1.),(1.,1.),(1.,1.),(1.,1.),(1.,1.),(1.,1.),(1.,1.),(1.,1.),(1.,
1.),(1.,1.),(1.,1.),(1.,1.),(1.,1.),(1.,1.),(1.,1.),(1.,1.),(1.,1.),(1.,
1.),(1.,1.)))
REPRESENTATION_ITEM('')
SURFACE()
);
#251=(
BOUNDED_CURVE()
B_SPLINE_CURVE(5,(#37694,#37695,#37696,#37697,#37698,#37699,#37700,#37701,
#37702,#37703,#37704,#37705,#37706,#37707,#37708,#37709,#37710,#37711,#37712,
#37713,#37714,#37715,#37716,#37717,#37718,#37719,#37720,#37721,#37722,#37723,
#37724,#37725,#37726,#37727,#37728,#37729,#37730,#37731,#37732,#37733,#37734,
#37735,#37736,#37737,#37738,#37739,#37740,#37741,#37742,#37743,#37744,#37745,
#37746,#37747,#37748,#37749,#37750,#37751,#37752,#37753,#37754,#37755,#37756,
#37757,#37758,#37759,#37760,#37761,#37762,#37763),.UNSPECIFIED.,.F.,.F.)
B_SPLINE_CURVE_WITH_KNOTS((6,1,1,1,1,1,1,1,1,1,1,1,1,1,1,1,1,1,1,1,1,1,
1,1,1,1,1,1,1,1,1,1,1,1,1,1,1,1,1,1,1,1,1,1,1,1,1,1,1,1,1,1,1,1,1,1,1,1,
1,1,1,1,1,1,1,6),(0.,0.0153846153846154,0.0307692307692308,0.0461538461538462,
0.0615384615384615,0.0769230769230769,0.0923076923076923,0.107692307692308,
0.123076923076923,0.138461538461538,0.153846153846154,0.169230769230769,
0.184615384615385,0.2,0.215384615384615,0.230769230769231,0.246153846153846,
0.261538461538462,0.276923076923077,0.292307692307692,0.307692307692308,
0.323076923076923,0.338461538461538,0.353846153846154,0.369230769230769,
0.384615384615385,0.4,0.415384615384615,0.430769230769231,0.446153846153846,
0.461538461538462,0.476923076923077,0.492307692307692,0.507692307692308,
0.523076923076923,0.538461538461538,0.553846153846154,0.569230769230769,
0.584615384615384,0.6,0.615384615384615,0.63076923076923,0.646153846153846,
0.661538461538461,0.676923076923076,0.692307692307692,0.707692307692307,
0.723076923076922,0.738461538461538,0.753846153846153,0.769230769230768,
0.784615384615384,0.799999999999999,0.815384615384614,0.83076923076923,
0.846153846153845,0.86153846153846,0.876923076923076,0.892307692307691,
0.907692307692306,0.923076923076922,0.938461538461537,0.953846153846152,
0.969230769230768,0.984615384615383,1.),.UNSPECIFIED.)
CURVE()
GEOMETRIC_REPRESENTATION_ITEM()
RATIONAL_B_SPLINE_CURVE((1.,1.,1.,1.,1.,1.,1.,1.,1.,1.,1.,1.,1.,1.,1.,1.,
1.,1.,1.,1.,1.,1.,1.,1.,1.,1.,1.,1.,1.,1.,1.,1.,1.,1.,1.,1.,1.,1.,1.,1.,
1.,1.,1.,1.,1.,1.,1.,1.,1.,1.,1.,1.,1.,1.,1.,1.,1.,1.,1.,1.,1.,1.,1.,1.,
1.,1.,1.,1.,1.,1.))
REPRESENTATION_ITEM('')
);
#252=(
BOUNDED_CURVE()
B_SPLINE_CURVE(5,(#37767,#37768,#37769,#37770,#37771,#37772,#37773,#37774,
#37775,#37776,#37777,#37778,#37779,#37780,#37781,#37782,#37783,#37784,#37785,
#37786,#37787,#37788,#37789,#37790,#37791,#37792,#37793,#37794,#37795,#37796,
#37797,#37798,#37799,#37800,#37801,#37802,#37803,#37804,#37805,#37806,#37807,
#37808,#37809,#37810,#37811,#37812,#37813,#37814,#37815,#37816,#37817,#37818,
#37819,#37820,#37821,#37822,#37823,#37824,#37825,#37826,#37827,#37828,#37829,
#37830,#37831,#37832,#37833,#37834,#37835,#37836),.UNSPECIFIED.,.F.,.F.)
B_SPLINE_CURVE_WITH_KNOTS((6,1,1,1,1,1,1,1,1,1,1,1,1,1,1,1,1,1,1,1,1,1,
1,1,1,1,1,1,1,1,1,1,1,1,1,1,1,1,1,1,1,1,1,1,1,1,1,1,1,1,1,1,1,1,1,1,1,1,
1,1,1,1,1,1,1,6),(0.,0.0153846153846154,0.0307692307692308,0.0461538461538462,
0.0615384615384615,0.0769230769230769,0.0923076923076923,0.107692307692308,
0.123076923076923,0.138461538461538,0.153846153846154,0.169230769230769,
0.184615384615385,0.2,0.215384615384615,0.230769230769231,0.246153846153846,
0.261538461538462,0.276923076923077,0.292307692307692,0.307692307692308,
0.323076923076923,0.338461538461538,0.353846153846154,0.369230769230769,
0.384615384615385,0.4,0.415384615384615,0.430769230769231,0.446153846153846,
0.461538461538462,0.476923076923077,0.492307692307692,0.507692307692308,
0.523076923076923,0.538461538461538,0.553846153846154,0.569230769230769,
0.584615384615384,0.6,0.615384615384615,0.63076923076923,0.646153846153846,
0.661538461538461,0.676923076923076,0.692307692307692,0.707692307692307,
0.723076923076922,0.738461538461538,0.753846153846153,0.769230769230768,
0.784615384615384,0.799999999999999,0.815384615384614,0.83076923076923,
0.846153846153845,0.86153846153846,0.876923076923076,0.892307692307691,
0.907692307692306,0.923076923076922,0.938461538461537,0.953846153846152,
0.969230769230768,0.984615384615383,1.),.UNSPECIFIED.)
CURVE()
GEOMETRIC_REPRESENTATION_ITEM()
RATIONAL_B_SPLINE_CURVE((1.,1.,1.,1.,1.,1.,1.,1.,1.,1.,1.,1.,1.,1.,1.,1.,
1.,1.,1.,1.,1.,1.,1.,1.,1.,1.,1.,1.,1.,1.,1.,1.,1.,1.,1.,1.,1.,1.,1.,1.,
1.,1.,1.,1.,1.,1.,1.,1.,1.,1.,1.,1.,1.,1.,1.,1.,1.,1.,1.,1.,1.,1.,1.,1.,
1.,1.,1.,1.,1.,1.))
REPRESENTATION_ITEM('')
);
#253=(
BOUNDED_CURVE()
B_SPLINE_CURVE(5,(#37840,#37841,#37842,#37843,#37844,#37845,#37846,#37847,
#37848,#37849,#37850,#37851,#37852,#37853,#37854,#37855,#37856,#37857,#37858,
#37859,#37860,#37861,#37862,#37863,#37864,#37865,#37866,#37867,#37868,#37869,
#37870,#37871,#37872,#37873,#37874,#37875,#37876,#37877,#37878,#37879,#37880,
#37881,#37882,#37883,#37884,#37885,#37886,#37887,#37888,#37889,#37890,#37891,
#37892,#37893,#37894,#37895,#37896,#37897,#37898,#37899,#37900,#37901,#37902,
#37903,#37904,#37905,#37906,#37907,#37908,#37909),.UNSPECIFIED.,.F.,.F.)
B_SPLINE_CURVE_WITH_KNOTS((6,1,1,1,1,1,1,1,1,1,1,1,1,1,1,1,1,1,1,1,1,1,
1,1,1,1,1,1,1,1,1,1,1,1,1,1,1,1,1,1,1,1,1,1,1,1,1,1,1,1,1,1,1,1,1,1,1,1,
1,1,1,1,1,1,1,6),(0.,0.0153846153846154,0.0307692307692308,0.0461538461538462,
0.0615384615384615,0.0769230769230769,0.0923076923076923,0.107692307692308,
0.123076923076923,0.138461538461538,0.153846153846154,0.169230769230769,
0.184615384615385,0.2,0.215384615384615,0.230769230769231,0.246153846153846,
0.261538461538462,0.276923076923077,0.292307692307692,0.307692307692308,
0.323076923076923,0.338461538461538,0.353846153846154,0.369230769230769,
0.384615384615385,0.4,0.415384615384615,0.430769230769231,0.446153846153846,
0.461538461538462,0.476923076923077,0.492307692307692,0.507692307692308,
0.523076923076923,0.538461538461538,0.553846153846154,0.569230769230769,
0.584615384615384,0.6,0.615384615384615,0.63076923076923,0.646153846153846,
0.661538461538461,0.676923076923076,0.692307692307692,0.707692307692307,
0.723076923076922,0.738461538461538,0.753846153846153,0.769230769230768,
0.784615384615384,0.799999999999999,0.815384615384614,0.83076923076923,
0.846153846153845,0.86153846153846,0.876923076923076,0.892307692307691,
0.907692307692306,0.923076923076922,0.938461538461537,0.953846153846152,
0.969230769230768,0.984615384615383,1.),.UNSPECIFIED.)
CURVE()
GEOMETRIC_REPRESENTATION_ITEM()
RATIONAL_B_SPLINE_CURVE((1.,1.,1.,1.,1.,1.,1.,1.,1.,1.,1.,1.,1.,1.,1.,1.,
1.,1.,1.,1.,1.,1.,1.,1.,1.,1.,1.,1.,1.,1.,1.,1.,1.,1.,1.,1.,1.,1.,1.,1.,
1.,1.,1.,1.,1.,1.,1.,1.,1.,1.,1.,1.,1.,1.,1.,1.,1.,1.,1.,1.,1.,1.,1.,1.,
1.,1.,1.,1.,1.,1.))
REPRESENTATION_ITEM('')
);
#254=(
BOUNDED_CURVE()
B_SPLINE_CURVE(5,(#37913,#37914,#37915,#37916,#37917,#37918,#37919,#37920,
#37921,#37922,#37923,#37924,#37925,#37926,#37927,#37928,#37929,#37930,#37931,
#37932,#37933,#37934,#37935,#37936,#37937,#37938,#37939,#37940,#37941,#37942,
#37943,#37944,#37945,#37946,#37947,#37948,#37949,#37950,#37951,#37952,#37953,
#37954,#37955,#37956,#37957,#37958,#37959,#37960,#37961,#37962,#37963,#37964,
#37965,#37966,#37967,#37968,#37969,#37970,#37971,#37972,#37973,#37974,#37975,
#37976,#37977,#37978,#37979,#37980,#37981,#37982),.UNSPECIFIED.,.F.,.F.)
B_SPLINE_CURVE_WITH_KNOTS((6,1,1,1,1,1,1,1,1,1,1,1,1,1,1,1,1,1,1,1,1,1,
1,1,1,1,1,1,1,1,1,1,1,1,1,1,1,1,1,1,1,1,1,1,1,1,1,1,1,1,1,1,1,1,1,1,1,1,
1,1,1,1,1,1,1,6),(0.,0.0153846153846154,0.0307692307692308,0.0461538461538462,
0.0615384615384615,0.0769230769230769,0.0923076923076923,0.107692307692308,
0.123076923076923,0.138461538461538,0.153846153846154,0.169230769230769,
0.184615384615385,0.2,0.215384615384615,0.230769230769231,0.246153846153846,
0.261538461538462,0.276923076923077,0.292307692307692,0.307692307692308,
0.323076923076923,0.338461538461538,0.353846153846154,0.369230769230769,
0.384615384615385,0.4,0.415384615384615,0.430769230769231,0.446153846153846,
0.461538461538462,0.476923076923077,0.492307692307692,0.507692307692308,
0.523076923076923,0.538461538461538,0.553846153846154,0.569230769230769,
0.584615384615384,0.6,0.615384615384615,0.63076923076923,0.646153846153846,
0.661538461538461,0.676923076923076,0.692307692307692,0.707692307692307,
0.723076923076922,0.738461538461538,0.753846153846153,0.769230769230768,
0.784615384615384,0.799999999999999,0.815384615384614,0.83076923076923,
0.846153846153845,0.86153846153846,0.876923076923076,0.892307692307691,
0.907692307692306,0.923076923076922,0.938461538461537,0.953846153846152,
0.969230769230768,0.984615384615383,1.),.UNSPECIFIED.)
CURVE()
GEOMETRIC_REPRESENTATION_ITEM()
RATIONAL_B_SPLINE_CURVE((1.,1.,1.,1.,1.,1.,1.,1.,1.,1.,1.,1.,1.,1.,1.,1.,
1.,1.,1.,1.,1.,1.,1.,1.,1.,1.,1.,1.,1.,1.,1.,1.,1.,1.,1.,1.,1.,1.,1.,1.,
1.,1.,1.,1.,1.,1.,1.,1.,1.,1.,1.,1.,1.,1.,1.,1.,1.,1.,1.,1.,1.,1.,1.,1.,
1.,1.,1.,1.,1.,1.))
REPRESENTATION_ITEM('')
);
#255=(
BOUNDED_CURVE()
B_SPLINE_CURVE(5,(#37986,#37987,#37988,#37989,#37990,#37991,#37992,#37993,
#37994,#37995,#37996,#37997,#37998,#37999,#38000,#38001,#38002,#38003,#38004,
#38005,#38006,#38007,#38008,#38009,#38010,#38011,#38012,#38013,#38014,#38015,
#38016,#38017,#38018,#38019,#38020,#38021,#38022,#38023,#38024,#38025,#38026,
#38027,#38028,#38029,#38030,#38031,#38032,#38033,#38034,#38035,#38036,#38037,
#38038,#38039,#38040,#38041,#38042,#38043,#38044,#38045,#38046,#38047,#38048,
#38049,#38050,#38051,#38052,#38053,#38054,#38055),.UNSPECIFIED.,.F.,.F.)
B_SPLINE_CURVE_WITH_KNOTS((6,1,1,1,1,1,1,1,1,1,1,1,1,1,1,1,1,1,1,1,1,1,
1,1,1,1,1,1,1,1,1,1,1,1,1,1,1,1,1,1,1,1,1,1,1,1,1,1,1,1,1,1,1,1,1,1,1,1,
1,1,1,1,1,1,1,6),(0.,0.0153846153846154,0.0307692307692308,0.0461538461538462,
0.0615384615384615,0.0769230769230769,0.0923076923076923,0.107692307692308,
0.123076923076923,0.138461538461538,0.153846153846154,0.169230769230769,
0.184615384615385,0.2,0.215384615384615,0.230769230769231,0.246153846153846,
0.261538461538462,0.276923076923077,0.292307692307692,0.307692307692308,
0.323076923076923,0.338461538461538,0.353846153846154,0.369230769230769,
0.384615384615385,0.4,0.415384615384615,0.430769230769231,0.446153846153846,
0.461538461538462,0.476923076923077,0.492307692307692,0.507692307692308,
0.523076923076923,0.538461538461538,0.553846153846154,0.569230769230769,
0.584615384615384,0.6,0.615384615384615,0.63076923076923,0.646153846153846,
0.661538461538461,0.676923076923076,0.692307692307692,0.707692307692307,
0.723076923076922,0.738461538461538,0.753846153846153,0.769230769230768,
0.784615384615384,0.799999999999999,0.815384615384614,0.83076923076923,
0.846153846153845,0.86153846153846,0.876923076923076,0.892307692307691,
0.907692307692306,0.923076923076922,0.938461538461537,0.953846153846152,
0.969230769230768,0.984615384615383,1.),.UNSPECIFIED.)
CURVE()
GEOMETRIC_REPRESENTATION_ITEM()
RATIONAL_B_SPLINE_CURVE((1.,1.,1.,1.,1.,1.,1.,1.,1.,1.,1.,1.,1.,1.,1.,1.,
1.,1.,1.,1.,1.,1.,1.,1.,1.,1.,1.,1.,1.,1.,1.,1.,1.,1.,1.,1.,1.,1.,1.,1.,
1.,1.,1.,1.,1.,1.,1.,1.,1.,1.,1.,1.,1.,1.,1.,1.,1.,1.,1.,1.,1.,1.,1.,1.,
1.,1.,1.,1.,1.,1.))
REPRESENTATION_ITEM('')
);
#256=(
BOUNDED_CURVE()
B_SPLINE_CURVE(5,(#38059,#38060,#38061,#38062,#38063,#38064,#38065,#38066,
#38067,#38068,#38069,#38070,#38071,#38072,#38073,#38074,#38075,#38076,#38077,
#38078,#38079,#38080,#38081,#38082,#38083,#38084,#38085,#38086,#38087,#38088,
#38089,#38090,#38091,#38092,#38093,#38094,#38095,#38096,#38097,#38098,#38099,
#38100,#38101,#38102,#38103,#38104,#38105,#38106,#38107,#38108,#38109,#38110,
#38111,#38112,#38113,#38114,#38115,#38116,#38117,#38118,#38119,#38120,#38121,
#38122,#38123,#38124,#38125,#38126,#38127,#38128),.UNSPECIFIED.,.F.,.F.)
B_SPLINE_CURVE_WITH_KNOTS((6,1,1,1,1,1,1,1,1,1,1,1,1,1,1,1,1,1,1,1,1,1,
1,1,1,1,1,1,1,1,1,1,1,1,1,1,1,1,1,1,1,1,1,1,1,1,1,1,1,1,1,1,1,1,1,1,1,1,
1,1,1,1,1,1,1,6),(0.,0.0153846153846154,0.0307692307692308,0.0461538461538462,
0.0615384615384615,0.0769230769230769,0.0923076923076923,0.107692307692308,
0.123076923076923,0.138461538461538,0.153846153846154,0.169230769230769,
0.184615384615385,0.2,0.215384615384615,0.230769230769231,0.246153846153846,
0.261538461538462,0.276923076923077,0.292307692307692,0.307692307692308,
0.323076923076923,0.338461538461538,0.353846153846154,0.369230769230769,
0.384615384615385,0.4,0.415384615384615,0.430769230769231,0.446153846153846,
0.461538461538462,0.476923076923077,0.492307692307692,0.507692307692308,
0.523076923076923,0.538461538461538,0.553846153846154,0.569230769230769,
0.584615384615384,0.6,0.615384615384615,0.63076923076923,0.646153846153846,
0.661538461538461,0.676923076923076,0.692307692307692,0.707692307692307,
0.723076923076922,0.738461538461538,0.753846153846153,0.769230769230768,
0.784615384615384,0.799999999999999,0.815384615384614,0.83076923076923,
0.846153846153845,0.86153846153846,0.876923076923076,0.892307692307691,
0.907692307692306,0.923076923076922,0.938461538461537,0.953846153846152,
0.969230769230768,0.984615384615383,1.),.UNSPECIFIED.)
CURVE()
GEOMETRIC_REPRESENTATION_ITEM()
RATIONAL_B_SPLINE_CURVE((1.,1.,1.,1.,1.,1.,1.,1.,1.,1.,1.,1.,1.,1.,1.,1.,
1.,1.,1.,1.,1.,1.,1.,1.,1.,1.,1.,1.,1.,1.,1.,1.,1.,1.,1.,1.,1.,1.,1.,1.,
1.,1.,1.,1.,1.,1.,1.,1.,1.,1.,1.,1.,1.,1.,1.,1.,1.,1.,1.,1.,1.,1.,1.,1.,
1.,1.,1.,1.,1.,1.))
REPRESENTATION_ITEM('')
);
#257=(
BOUNDED_CURVE()
B_SPLINE_CURVE(5,(#38132,#38133,#38134,#38135,#38136,#38137,#38138,#38139,
#38140,#38141,#38142,#38143,#38144,#38145,#38146,#38147,#38148,#38149,#38150,
#38151,#38152,#38153,#38154,#38155,#38156,#38157,#38158,#38159,#38160,#38161,
#38162,#38163,#38164,#38165,#38166,#38167,#38168,#38169,#38170,#38171,#38172,
#38173,#38174,#38175,#38176,#38177,#38178,#38179,#38180,#38181,#38182,#38183,
#38184,#38185,#38186,#38187,#38188,#38189,#38190,#38191,#38192,#38193,#38194,
#38195,#38196,#38197,#38198,#38199,#38200,#38201),.UNSPECIFIED.,.F.,.F.)
B_SPLINE_CURVE_WITH_KNOTS((6,1,1,1,1,1,1,1,1,1,1,1,1,1,1,1,1,1,1,1,1,1,
1,1,1,1,1,1,1,1,1,1,1,1,1,1,1,1,1,1,1,1,1,1,1,1,1,1,1,1,1,1,1,1,1,1,1,1,
1,1,1,1,1,1,1,6),(0.,0.0153846153846154,0.0307692307692308,0.0461538461538462,
0.0615384615384615,0.0769230769230769,0.0923076923076923,0.107692307692308,
0.123076923076923,0.138461538461538,0.153846153846154,0.169230769230769,
0.184615384615385,0.2,0.215384615384615,0.230769230769231,0.246153846153846,
0.261538461538462,0.276923076923077,0.292307692307692,0.307692307692308,
0.323076923076923,0.338461538461538,0.353846153846154,0.369230769230769,
0.384615384615385,0.4,0.415384615384615,0.430769230769231,0.446153846153846,
0.461538461538462,0.476923076923077,0.492307692307692,0.507692307692308,
0.523076923076923,0.538461538461538,0.553846153846154,0.569230769230769,
0.584615384615384,0.6,0.615384615384615,0.63076923076923,0.646153846153846,
0.661538461538461,0.676923076923076,0.692307692307692,0.707692307692307,
0.723076923076922,0.738461538461538,0.753846153846153,0.769230769230768,
0.784615384615384,0.799999999999999,0.815384615384614,0.83076923076923,
0.846153846153845,0.86153846153846,0.876923076923076,0.892307692307691,
0.907692307692306,0.923076923076922,0.938461538461537,0.953846153846152,
0.969230769230768,0.984615384615383,1.),.UNSPECIFIED.)
CURVE()
GEOMETRIC_REPRESENTATION_ITEM()
RATIONAL_B_SPLINE_CURVE((1.,1.,1.,1.,1.,1.,1.,1.,1.,1.,1.,1.,1.,1.,1.,1.,
1.,1.,1.,1.,1.,1.,1.,1.,1.,1.,1.,1.,1.,1.,1.,1.,1.,1.,1.,1.,1.,1.,1.,1.,
1.,1.,1.,1.,1.,1.,1.,1.,1.,1.,1.,1.,1.,1.,1.,1.,1.,1.,1.,1.,1.,1.,1.,1.,
1.,1.,1.,1.,1.,1.))
REPRESENTATION_ITEM('')
);
#258=(
BOUNDED_CURVE()
B_SPLINE_CURVE(5,(#38205,#38206,#38207,#38208,#38209,#38210,#38211,#38212,
#38213,#38214,#38215,#38216,#38217,#38218,#38219,#38220,#38221,#38222,#38223,
#38224,#38225,#38226,#38227,#38228,#38229,#38230,#38231,#38232,#38233,#38234,
#38235,#38236,#38237,#38238,#38239,#38240,#38241,#38242,#38243,#38244,#38245,
#38246,#38247,#38248,#38249,#38250,#38251,#38252,#38253,#38254,#38255,#38256,
#38257,#38258,#38259,#38260,#38261,#38262,#38263,#38264,#38265,#38266,#38267,
#38268,#38269,#38270,#38271,#38272,#38273,#38274),.UNSPECIFIED.,.F.,.F.)
B_SPLINE_CURVE_WITH_KNOTS((6,1,1,1,1,1,1,1,1,1,1,1,1,1,1,1,1,1,1,1,1,1,
1,1,1,1,1,1,1,1,1,1,1,1,1,1,1,1,1,1,1,1,1,1,1,1,1,1,1,1,1,1,1,1,1,1,1,1,
1,1,1,1,1,1,1,6),(0.,0.0153846153846154,0.0307692307692308,0.0461538461538462,
0.0615384615384615,0.0769230769230769,0.0923076923076923,0.107692307692308,
0.123076923076923,0.138461538461538,0.153846153846154,0.169230769230769,
0.184615384615385,0.2,0.215384615384615,0.230769230769231,0.246153846153846,
0.261538461538462,0.276923076923077,0.292307692307692,0.307692307692308,
0.323076923076923,0.338461538461538,0.353846153846154,0.369230769230769,
0.384615384615385,0.4,0.415384615384615,0.430769230769231,0.446153846153846,
0.461538461538462,0.476923076923077,0.492307692307692,0.507692307692308,
0.523076923076923,0.538461538461538,0.553846153846154,0.569230769230769,
0.584615384615384,0.6,0.615384615384615,0.63076923076923,0.646153846153846,
0.661538461538461,0.676923076923076,0.692307692307692,0.707692307692307,
0.723076923076922,0.738461538461538,0.753846153846153,0.769230769230768,
0.784615384615384,0.799999999999999,0.815384615384614,0.83076923076923,
0.846153846153845,0.86153846153846,0.876923076923076,0.892307692307691,
0.907692307692306,0.923076923076922,0.938461538461537,0.953846153846152,
0.969230769230768,0.984615384615383,1.),.UNSPECIFIED.)
CURVE()
GEOMETRIC_REPRESENTATION_ITEM()
RATIONAL_B_SPLINE_CURVE((1.,1.,1.,1.,1.,1.,1.,1.,1.,1.,1.,1.,1.,1.,1.,1.,
1.,1.,1.,1.,1.,1.,1.,1.,1.,1.,1.,1.,1.,1.,1.,1.,1.,1.,1.,1.,1.,1.,1.,1.,
1.,1.,1.,1.,1.,1.,1.,1.,1.,1.,1.,1.,1.,1.,1.,1.,1.,1.,1.,1.,1.,1.,1.,1.,
1.,1.,1.,1.,1.,1.))
REPRESENTATION_ITEM('')
);
#259=(
BOUNDED_CURVE()
B_SPLINE_CURVE(5,(#38278,#38279,#38280,#38281,#38282,#38283,#38284,#38285,
#38286,#38287,#38288,#38289,#38290,#38291,#38292,#38293,#38294,#38295,#38296,
#38297,#38298,#38299,#38300,#38301,#38302,#38303,#38304,#38305,#38306,#38307,
#38308,#38309,#38310,#38311,#38312,#38313,#38314,#38315,#38316,#38317,#38318,
#38319,#38320,#38321,#38322,#38323,#38324,#38325,#38326,#38327,#38328,#38329,
#38330,#38331,#38332,#38333,#38334,#38335,#38336,#38337,#38338,#38339,#38340,
#38341,#38342,#38343,#38344,#38345,#38346,#38347),.UNSPECIFIED.,.F.,.F.)
B_SPLINE_CURVE_WITH_KNOTS((6,1,1,1,1,1,1,1,1,1,1,1,1,1,1,1,1,1,1,1,1,1,
1,1,1,1,1,1,1,1,1,1,1,1,1,1,1,1,1,1,1,1,1,1,1,1,1,1,1,1,1,1,1,1,1,1,1,1,
1,1,1,1,1,1,1,6),(0.,0.0153846153846154,0.0307692307692308,0.0461538461538462,
0.0615384615384615,0.0769230769230769,0.0923076923076923,0.107692307692308,
0.123076923076923,0.138461538461538,0.153846153846154,0.169230769230769,
0.184615384615385,0.2,0.215384615384615,0.230769230769231,0.246153846153846,
0.261538461538462,0.276923076923077,0.292307692307692,0.307692307692308,
0.323076923076923,0.338461538461538,0.353846153846154,0.369230769230769,
0.384615384615385,0.4,0.415384615384615,0.430769230769231,0.446153846153846,
0.461538461538462,0.476923076923077,0.492307692307692,0.507692307692308,
0.523076923076923,0.538461538461538,0.553846153846154,0.569230769230769,
0.584615384615384,0.6,0.615384615384615,0.63076923076923,0.646153846153846,
0.661538461538461,0.676923076923076,0.692307692307692,0.707692307692307,
0.723076923076922,0.738461538461538,0.753846153846153,0.769230769230768,
0.784615384615384,0.799999999999999,0.815384615384614,0.83076923076923,
0.846153846153845,0.86153846153846,0.876923076923076,0.892307692307691,
0.907692307692306,0.923076923076922,0.938461538461537,0.953846153846152,
0.969230769230768,0.984615384615383,1.),.UNSPECIFIED.)
CURVE()
GEOMETRIC_REPRESENTATION_ITEM()
RATIONAL_B_SPLINE_CURVE((1.,1.,1.,1.,1.,1.,1.,1.,1.,1.,1.,1.,1.,1.,1.,1.,
1.,1.,1.,1.,1.,1.,1.,1.,1.,1.,1.,1.,1.,1.,1.,1.,1.,1.,1.,1.,1.,1.,1.,1.,
1.,1.,1.,1.,1.,1.,1.,1.,1.,1.,1.,1.,1.,1.,1.,1.,1.,1.,1.,1.,1.,1.,1.,1.,
1.,1.,1.,1.,1.,1.))
REPRESENTATION_ITEM('')
);
#260=(
BOUNDED_CURVE()
B_SPLINE_CURVE(5,(#38351,#38352,#38353,#38354,#38355,#38356,#38357,#38358,
#38359,#38360,#38361,#38362,#38363,#38364,#38365,#38366,#38367,#38368,#38369,
#38370,#38371,#38372,#38373,#38374,#38375,#38376,#38377,#38378,#38379,#38380,
#38381,#38382,#38383,#38384,#38385,#38386,#38387,#38388,#38389,#38390,#38391,
#38392,#38393,#38394,#38395,#38396,#38397,#38398,#38399,#38400,#38401,#38402,
#38403,#38404,#38405,#38406,#38407,#38408,#38409,#38410,#38411,#38412,#38413,
#38414,#38415,#38416,#38417,#38418,#38419,#38420),.UNSPECIFIED.,.F.,.F.)
B_SPLINE_CURVE_WITH_KNOTS((6,1,1,1,1,1,1,1,1,1,1,1,1,1,1,1,1,1,1,1,1,1,
1,1,1,1,1,1,1,1,1,1,1,1,1,1,1,1,1,1,1,1,1,1,1,1,1,1,1,1,1,1,1,1,1,1,1,1,
1,1,1,1,1,1,1,6),(0.,0.0153846153846154,0.0307692307692308,0.0461538461538462,
0.0615384615384615,0.0769230769230769,0.0923076923076923,0.107692307692308,
0.123076923076923,0.138461538461538,0.153846153846154,0.169230769230769,
0.184615384615385,0.2,0.215384615384615,0.230769230769231,0.246153846153846,
0.261538461538462,0.276923076923077,0.292307692307692,0.307692307692308,
0.323076923076923,0.338461538461538,0.353846153846154,0.369230769230769,
0.384615384615385,0.4,0.415384615384615,0.430769230769231,0.446153846153846,
0.461538461538462,0.476923076923077,0.492307692307692,0.507692307692308,
0.523076923076923,0.538461538461538,0.553846153846154,0.569230769230769,
0.584615384615384,0.6,0.615384615384615,0.63076923076923,0.646153846153846,
0.661538461538461,0.676923076923076,0.692307692307692,0.707692307692307,
0.723076923076922,0.738461538461538,0.753846153846153,0.769230769230768,
0.784615384615384,0.799999999999999,0.815384615384614,0.83076923076923,
0.846153846153845,0.86153846153846,0.876923076923076,0.892307692307691,
0.907692307692306,0.923076923076922,0.938461538461537,0.953846153846152,
0.969230769230768,0.984615384615383,1.),.UNSPECIFIED.)
CURVE()
GEOMETRIC_REPRESENTATION_ITEM()
RATIONAL_B_SPLINE_CURVE((1.,1.,1.,1.,1.,1.,1.,1.,1.,1.,1.,1.,1.,1.,1.,1.,
1.,1.,1.,1.,1.,1.,1.,1.,1.,1.,1.,1.,1.,1.,1.,1.,1.,1.,1.,1.,1.,1.,1.,1.,
1.,1.,1.,1.,1.,1.,1.,1.,1.,1.,1.,1.,1.,1.,1.,1.,1.,1.,1.,1.,1.,1.,1.,1.,
1.,1.,1.,1.,1.,1.))
REPRESENTATION_ITEM('')
);
#261=(
BOUNDED_CURVE()
B_SPLINE_CURVE(5,(#38424,#38425,#38426,#38427,#38428,#38429,#38430,#38431,
#38432,#38433,#38434,#38435,#38436,#38437,#38438,#38439,#38440,#38441,#38442,
#38443,#38444,#38445,#38446,#38447,#38448,#38449,#38450,#38451,#38452,#38453,
#38454,#38455,#38456,#38457,#38458,#38459,#38460,#38461,#38462,#38463,#38464,
#38465,#38466,#38467,#38468,#38469,#38470,#38471,#38472,#38473,#38474,#38475,
#38476,#38477,#38478,#38479,#38480,#38481,#38482,#38483,#38484,#38485,#38486,
#38487,#38488,#38489,#38490,#38491,#38492,#38493),.UNSPECIFIED.,.F.,.F.)
B_SPLINE_CURVE_WITH_KNOTS((6,1,1,1,1,1,1,1,1,1,1,1,1,1,1,1,1,1,1,1,1,1,
1,1,1,1,1,1,1,1,1,1,1,1,1,1,1,1,1,1,1,1,1,1,1,1,1,1,1,1,1,1,1,1,1,1,1,1,
1,1,1,1,1,1,1,6),(0.,0.0153846153846154,0.0307692307692308,0.0461538461538462,
0.0615384615384615,0.0769230769230769,0.0923076923076923,0.107692307692308,
0.123076923076923,0.138461538461538,0.153846153846154,0.169230769230769,
0.184615384615385,0.2,0.215384615384615,0.230769230769231,0.246153846153846,
0.261538461538462,0.276923076923077,0.292307692307692,0.307692307692308,
0.323076923076923,0.338461538461538,0.353846153846154,0.369230769230769,
0.384615384615385,0.4,0.415384615384615,0.430769230769231,0.446153846153846,
0.461538461538462,0.476923076923077,0.492307692307692,0.507692307692308,
0.523076923076923,0.538461538461538,0.553846153846154,0.569230769230769,
0.584615384615384,0.6,0.615384615384615,0.63076923076923,0.646153846153846,
0.661538461538461,0.676923076923076,0.692307692307692,0.707692307692307,
0.723076923076922,0.738461538461538,0.753846153846153,0.769230769230768,
0.784615384615384,0.799999999999999,0.815384615384614,0.83076923076923,
0.846153846153845,0.86153846153846,0.876923076923076,0.892307692307691,
0.907692307692306,0.923076923076922,0.938461538461537,0.953846153846152,
0.969230769230768,0.984615384615383,1.),.UNSPECIFIED.)
CURVE()
GEOMETRIC_REPRESENTATION_ITEM()
RATIONAL_B_SPLINE_CURVE((1.,1.,1.,1.,1.,1.,1.,1.,1.,1.,1.,1.,1.,1.,1.,1.,
1.,1.,1.,1.,1.,1.,1.,1.,1.,1.,1.,1.,1.,1.,1.,1.,1.,1.,1.,1.,1.,1.,1.,1.,
1.,1.,1.,1.,1.,1.,1.,1.,1.,1.,1.,1.,1.,1.,1.,1.,1.,1.,1.,1.,1.,1.,1.,1.,
1.,1.,1.,1.,1.,1.))
REPRESENTATION_ITEM('')
);
#262=(
BOUNDED_CURVE()
B_SPLINE_CURVE(5,(#38497,#38498,#38499,#38500,#38501,#38502,#38503,#38504,
#38505,#38506,#38507,#38508,#38509,#38510,#38511,#38512,#38513,#38514,#38515,
#38516,#38517,#38518,#38519,#38520,#38521,#38522,#38523,#38524,#38525,#38526,
#38527,#38528,#38529,#38530,#38531,#38532,#38533,#38534,#38535,#38536,#38537,
#38538,#38539,#38540,#38541,#38542,#38543,#38544,#38545,#38546,#38547,#38548,
#38549,#38550,#38551,#38552,#38553,#38554,#38555,#38556,#38557,#38558,#38559,
#38560,#38561,#38562,#38563,#38564,#38565,#38566),.UNSPECIFIED.,.F.,.F.)
B_SPLINE_CURVE_WITH_KNOTS((6,1,1,1,1,1,1,1,1,1,1,1,1,1,1,1,1,1,1,1,1,1,
1,1,1,1,1,1,1,1,1,1,1,1,1,1,1,1,1,1,1,1,1,1,1,1,1,1,1,1,1,1,1,1,1,1,1,1,
1,1,1,1,1,1,1,6),(0.,0.0153846153846154,0.0307692307692308,0.0461538461538462,
0.0615384615384615,0.0769230769230769,0.0923076923076923,0.107692307692308,
0.123076923076923,0.138461538461538,0.153846153846154,0.169230769230769,
0.184615384615385,0.2,0.215384615384615,0.230769230769231,0.246153846153846,
0.261538461538462,0.276923076923077,0.292307692307692,0.307692307692308,
0.323076923076923,0.338461538461538,0.353846153846154,0.369230769230769,
0.384615384615385,0.4,0.415384615384615,0.430769230769231,0.446153846153846,
0.461538461538462,0.476923076923077,0.492307692307692,0.507692307692308,
0.523076923076923,0.538461538461538,0.553846153846154,0.569230769230769,
0.584615384615384,0.6,0.615384615384615,0.63076923076923,0.646153846153846,
0.661538461538461,0.676923076923076,0.692307692307692,0.707692307692307,
0.723076923076922,0.738461538461538,0.753846153846153,0.769230769230768,
0.784615384615384,0.799999999999999,0.815384615384614,0.83076923076923,
0.846153846153845,0.86153846153846,0.876923076923076,0.892307692307691,
0.907692307692306,0.923076923076922,0.938461538461537,0.953846153846152,
0.969230769230768,0.984615384615383,1.),.UNSPECIFIED.)
CURVE()
GEOMETRIC_REPRESENTATION_ITEM()
RATIONAL_B_SPLINE_CURVE((1.,1.,1.,1.,1.,1.,1.,1.,1.,1.,1.,1.,1.,1.,1.,1.,
1.,1.,1.,1.,1.,1.,1.,1.,1.,1.,1.,1.,1.,1.,1.,1.,1.,1.,1.,1.,1.,1.,1.,1.,
1.,1.,1.,1.,1.,1.,1.,1.,1.,1.,1.,1.,1.,1.,1.,1.,1.,1.,1.,1.,1.,1.,1.,1.,
1.,1.,1.,1.,1.,1.))
REPRESENTATION_ITEM('')
);
#263=(
BOUNDED_CURVE()
B_SPLINE_CURVE(5,(#38570,#38571,#38572,#38573,#38574,#38575,#38576,#38577,
#38578,#38579,#38580,#38581,#38582,#38583,#38584,#38585,#38586,#38587,#38588,
#38589,#38590,#38591,#38592,#38593,#38594,#38595,#38596,#38597,#38598,#38599,
#38600,#38601,#38602,#38603,#38604,#38605,#38606,#38607,#38608,#38609,#38610,
#38611,#38612,#38613,#38614,#38615,#38616,#38617,#38618,#38619,#38620,#38621,
#38622,#38623,#38624,#38625,#38626,#38627,#38628,#38629,#38630,#38631,#38632,
#38633,#38634,#38635,#38636,#38637,#38638,#38639),.UNSPECIFIED.,.F.,.F.)
B_SPLINE_CURVE_WITH_KNOTS((6,1,1,1,1,1,1,1,1,1,1,1,1,1,1,1,1,1,1,1,1,1,
1,1,1,1,1,1,1,1,1,1,1,1,1,1,1,1,1,1,1,1,1,1,1,1,1,1,1,1,1,1,1,1,1,1,1,1,
1,1,1,1,1,1,1,6),(0.,0.0153846153846154,0.0307692307692308,0.0461538461538462,
0.0615384615384615,0.0769230769230769,0.0923076923076923,0.107692307692308,
0.123076923076923,0.138461538461538,0.153846153846154,0.169230769230769,
0.184615384615385,0.2,0.215384615384615,0.230769230769231,0.246153846153846,
0.261538461538462,0.276923076923077,0.292307692307692,0.307692307692308,
0.323076923076923,0.338461538461538,0.353846153846154,0.369230769230769,
0.384615384615385,0.4,0.415384615384615,0.430769230769231,0.446153846153846,
0.461538461538462,0.476923076923077,0.492307692307692,0.507692307692308,
0.523076923076923,0.538461538461538,0.553846153846154,0.569230769230769,
0.584615384615384,0.6,0.615384615384615,0.63076923076923,0.646153846153846,
0.661538461538461,0.676923076923076,0.692307692307692,0.707692307692307,
0.723076923076922,0.738461538461538,0.753846153846153,0.769230769230768,
0.784615384615384,0.799999999999999,0.815384615384614,0.83076923076923,
0.846153846153845,0.86153846153846,0.876923076923076,0.892307692307691,
0.907692307692306,0.923076923076922,0.938461538461537,0.953846153846152,
0.969230769230768,0.984615384615383,1.),.UNSPECIFIED.)
CURVE()
GEOMETRIC_REPRESENTATION_ITEM()
RATIONAL_B_SPLINE_CURVE((1.,1.,1.,1.,1.,1.,1.,1.,1.,1.,1.,1.,1.,1.,1.,1.,
1.,1.,1.,1.,1.,1.,1.,1.,1.,1.,1.,1.,1.,1.,1.,1.,1.,1.,1.,1.,1.,1.,1.,1.,
1.,1.,1.,1.,1.,1.,1.,1.,1.,1.,1.,1.,1.,1.,1.,1.,1.,1.,1.,1.,1.,1.,1.,1.,
1.,1.,1.,1.,1.,1.))
REPRESENTATION_ITEM('')
);
#264=(
BOUNDED_CURVE()
B_SPLINE_CURVE(5,(#38643,#38644,#38645,#38646,#38647,#38648,#38649,#38650,
#38651,#38652,#38653,#38654,#38655,#38656,#38657,#38658,#38659,#38660,#38661,
#38662,#38663,#38664,#38665,#38666,#38667,#38668,#38669,#38670,#38671,#38672,
#38673,#38674,#38675,#38676,#38677,#38678,#38679,#38680,#38681,#38682,#38683,
#38684,#38685,#38686,#38687,#38688,#38689,#38690,#38691,#38692,#38693,#38694,
#38695,#38696,#38697,#38698,#38699,#38700,#38701,#38702,#38703,#38704,#38705,
#38706,#38707,#38708,#38709,#38710,#38711,#38712),.UNSPECIFIED.,.F.,.F.)
B_SPLINE_CURVE_WITH_KNOTS((6,1,1,1,1,1,1,1,1,1,1,1,1,1,1,1,1,1,1,1,1,1,
1,1,1,1,1,1,1,1,1,1,1,1,1,1,1,1,1,1,1,1,1,1,1,1,1,1,1,1,1,1,1,1,1,1,1,1,
1,1,1,1,1,1,1,6),(0.,0.0153846153846154,0.0307692307692308,0.0461538461538462,
0.0615384615384615,0.0769230769230769,0.0923076923076923,0.107692307692308,
0.123076923076923,0.138461538461538,0.153846153846154,0.169230769230769,
0.184615384615385,0.2,0.215384615384615,0.230769230769231,0.246153846153846,
0.261538461538462,0.276923076923077,0.292307692307692,0.307692307692308,
0.323076923076923,0.338461538461538,0.353846153846154,0.369230769230769,
0.384615384615385,0.4,0.415384615384615,0.430769230769231,0.446153846153846,
0.461538461538462,0.476923076923077,0.492307692307692,0.507692307692308,
0.523076923076923,0.538461538461538,0.553846153846154,0.569230769230769,
0.584615384615384,0.6,0.615384615384615,0.63076923076923,0.646153846153846,
0.661538461538461,0.676923076923076,0.692307692307692,0.707692307692307,
0.723076923076922,0.738461538461538,0.753846153846153,0.769230769230768,
0.784615384615384,0.799999999999999,0.815384615384614,0.83076923076923,
0.846153846153845,0.86153846153846,0.876923076923076,0.892307692307691,
0.907692307692306,0.923076923076922,0.938461538461537,0.953846153846152,
0.969230769230768,0.984615384615383,1.),.UNSPECIFIED.)
CURVE()
GEOMETRIC_REPRESENTATION_ITEM()
RATIONAL_B_SPLINE_CURVE((1.,1.,1.,1.,1.,1.,1.,1.,1.,1.,1.,1.,1.,1.,1.,1.,
1.,1.,1.,1.,1.,1.,1.,1.,1.,1.,1.,1.,1.,1.,1.,1.,1.,1.,1.,1.,1.,1.,1.,1.,
1.,1.,1.,1.,1.,1.,1.,1.,1.,1.,1.,1.,1.,1.,1.,1.,1.,1.,1.,1.,1.,1.,1.,1.,
1.,1.,1.,1.,1.,1.))
REPRESENTATION_ITEM('')
);
#265=(
BOUNDED_CURVE()
B_SPLINE_CURVE(5,(#38716,#38717,#38718,#38719,#38720,#38721,#38722,#38723,
#38724,#38725,#38726,#38727,#38728,#38729,#38730,#38731,#38732,#38733,#38734,
#38735,#38736,#38737,#38738,#38739,#38740,#38741,#38742,#38743,#38744,#38745,
#38746,#38747,#38748,#38749,#38750,#38751,#38752,#38753,#38754,#38755,#38756,
#38757,#38758,#38759,#38760,#38761,#38762,#38763,#38764,#38765,#38766,#38767,
#38768,#38769,#38770,#38771,#38772,#38773,#38774,#38775,#38776,#38777,#38778,
#38779,#38780,#38781,#38782,#38783,#38784,#38785),.UNSPECIFIED.,.F.,.F.)
B_SPLINE_CURVE_WITH_KNOTS((6,1,1,1,1,1,1,1,1,1,1,1,1,1,1,1,1,1,1,1,1,1,
1,1,1,1,1,1,1,1,1,1,1,1,1,1,1,1,1,1,1,1,1,1,1,1,1,1,1,1,1,1,1,1,1,1,1,1,
1,1,1,1,1,1,1,6),(0.,0.0153846153846154,0.0307692307692308,0.0461538461538462,
0.0615384615384615,0.0769230769230769,0.0923076923076923,0.107692307692308,
0.123076923076923,0.138461538461538,0.153846153846154,0.169230769230769,
0.184615384615385,0.2,0.215384615384615,0.230769230769231,0.246153846153846,
0.261538461538462,0.276923076923077,0.292307692307692,0.307692307692308,
0.323076923076923,0.338461538461538,0.353846153846154,0.369230769230769,
0.384615384615385,0.4,0.415384615384615,0.430769230769231,0.446153846153846,
0.461538461538462,0.476923076923077,0.492307692307692,0.507692307692308,
0.523076923076923,0.538461538461538,0.553846153846154,0.569230769230769,
0.584615384615384,0.6,0.615384615384615,0.63076923076923,0.646153846153846,
0.661538461538461,0.676923076923076,0.692307692307692,0.707692307692307,
0.723076923076922,0.738461538461538,0.753846153846153,0.769230769230768,
0.784615384615384,0.799999999999999,0.815384615384614,0.83076923076923,
0.846153846153845,0.86153846153846,0.876923076923076,0.892307692307691,
0.907692307692306,0.923076923076922,0.938461538461537,0.953846153846152,
0.969230769230768,0.984615384615383,1.),.UNSPECIFIED.)
CURVE()
GEOMETRIC_REPRESENTATION_ITEM()
RATIONAL_B_SPLINE_CURVE((1.,1.,1.,1.,1.,1.,1.,1.,1.,1.,1.,1.,1.,1.,1.,1.,
1.,1.,1.,1.,1.,1.,1.,1.,1.,1.,1.,1.,1.,1.,1.,1.,1.,1.,1.,1.,1.,1.,1.,1.,
1.,1.,1.,1.,1.,1.,1.,1.,1.,1.,1.,1.,1.,1.,1.,1.,1.,1.,1.,1.,1.,1.,1.,1.,
1.,1.,1.,1.,1.,1.))
REPRESENTATION_ITEM('')
);
#266=(
BOUNDED_CURVE()
B_SPLINE_CURVE(5,(#38789,#38790,#38791,#38792,#38793,#38794,#38795,#38796,
#38797,#38798,#38799,#38800,#38801,#38802,#38803,#38804,#38805,#38806,#38807,
#38808,#38809,#38810,#38811,#38812,#38813,#38814,#38815,#38816,#38817,#38818,
#38819,#38820,#38821,#38822,#38823,#38824,#38825,#38826,#38827,#38828,#38829,
#38830,#38831,#38832,#38833,#38834,#38835,#38836,#38837,#38838,#38839,#38840,
#38841,#38842,#38843,#38844,#38845,#38846,#38847,#38848,#38849,#38850,#38851,
#38852,#38853,#38854,#38855,#38856,#38857,#38858),.UNSPECIFIED.,.F.,.F.)
B_SPLINE_CURVE_WITH_KNOTS((6,1,1,1,1,1,1,1,1,1,1,1,1,1,1,1,1,1,1,1,1,1,
1,1,1,1,1,1,1,1,1,1,1,1,1,1,1,1,1,1,1,1,1,1,1,1,1,1,1,1,1,1,1,1,1,1,1,1,
1,1,1,1,1,1,1,6),(0.,0.0153846153846154,0.0307692307692308,0.0461538461538462,
0.0615384615384615,0.0769230769230769,0.0923076923076923,0.107692307692308,
0.123076923076923,0.138461538461538,0.153846153846154,0.169230769230769,
0.184615384615385,0.2,0.215384615384615,0.230769230769231,0.246153846153846,
0.261538461538462,0.276923076923077,0.292307692307692,0.307692307692308,
0.323076923076923,0.338461538461538,0.353846153846154,0.369230769230769,
0.384615384615385,0.4,0.415384615384615,0.430769230769231,0.446153846153846,
0.461538461538462,0.476923076923077,0.492307692307692,0.507692307692308,
0.523076923076923,0.538461538461538,0.553846153846154,0.569230769230769,
0.584615384615384,0.6,0.615384615384615,0.63076923076923,0.646153846153846,
0.661538461538461,0.676923076923076,0.692307692307692,0.707692307692307,
0.723076923076922,0.738461538461538,0.753846153846153,0.769230769230768,
0.784615384615384,0.799999999999999,0.815384615384614,0.83076923076923,
0.846153846153845,0.86153846153846,0.876923076923076,0.892307692307691,
0.907692307692306,0.923076923076922,0.938461538461537,0.953846153846152,
0.969230769230768,0.984615384615383,1.),.UNSPECIFIED.)
CURVE()
GEOMETRIC_REPRESENTATION_ITEM()
RATIONAL_B_SPLINE_CURVE((1.,1.,1.,1.,1.,1.,1.,1.,1.,1.,1.,1.,1.,1.,1.,1.,
1.,1.,1.,1.,1.,1.,1.,1.,1.,1.,1.,1.,1.,1.,1.,1.,1.,1.,1.,1.,1.,1.,1.,1.,
1.,1.,1.,1.,1.,1.,1.,1.,1.,1.,1.,1.,1.,1.,1.,1.,1.,1.,1.,1.,1.,1.,1.,1.,
1.,1.,1.,1.,1.,1.))
REPRESENTATION_ITEM('')
);
#267=(
BOUNDED_CURVE()
B_SPLINE_CURVE(5,(#38862,#38863,#38864,#38865,#38866,#38867,#38868,#38869,
#38870,#38871,#38872,#38873,#38874,#38875,#38876,#38877,#38878,#38879,#38880,
#38881,#38882,#38883,#38884,#38885,#38886,#38887,#38888,#38889,#38890,#38891,
#38892,#38893,#38894,#38895,#38896,#38897,#38898,#38899,#38900,#38901,#38902,
#38903,#38904,#38905,#38906,#38907,#38908,#38909,#38910,#38911,#38912,#38913,
#38914,#38915,#38916,#38917,#38918,#38919,#38920,#38921,#38922,#38923,#38924,
#38925,#38926,#38927,#38928,#38929,#38930,#38931),.UNSPECIFIED.,.F.,.F.)
B_SPLINE_CURVE_WITH_KNOTS((6,1,1,1,1,1,1,1,1,1,1,1,1,1,1,1,1,1,1,1,1,1,
1,1,1,1,1,1,1,1,1,1,1,1,1,1,1,1,1,1,1,1,1,1,1,1,1,1,1,1,1,1,1,1,1,1,1,1,
1,1,1,1,1,1,1,6),(0.,0.0153846153846154,0.0307692307692308,0.0461538461538462,
0.0615384615384615,0.0769230769230769,0.0923076923076923,0.107692307692308,
0.123076923076923,0.138461538461538,0.153846153846154,0.169230769230769,
0.184615384615385,0.2,0.215384615384615,0.230769230769231,0.246153846153846,
0.261538461538462,0.276923076923077,0.292307692307692,0.307692307692308,
0.323076923076923,0.338461538461538,0.353846153846154,0.369230769230769,
0.384615384615385,0.4,0.415384615384615,0.430769230769231,0.446153846153846,
0.461538461538462,0.476923076923077,0.492307692307692,0.507692307692308,
0.523076923076923,0.538461538461538,0.553846153846154,0.569230769230769,
0.584615384615384,0.6,0.615384615384615,0.63076923076923,0.646153846153846,
0.661538461538461,0.676923076923076,0.692307692307692,0.707692307692307,
0.723076923076922,0.738461538461538,0.753846153846153,0.769230769230768,
0.784615384615384,0.799999999999999,0.815384615384614,0.83076923076923,
0.846153846153845,0.86153846153846,0.876923076923076,0.892307692307691,
0.907692307692306,0.923076923076922,0.938461538461537,0.953846153846152,
0.969230769230768,0.984615384615383,1.),.UNSPECIFIED.)
CURVE()
GEOMETRIC_REPRESENTATION_ITEM()
RATIONAL_B_SPLINE_CURVE((1.,1.,1.,1.,1.,1.,1.,1.,1.,1.,1.,1.,1.,1.,1.,1.,
1.,1.,1.,1.,1.,1.,1.,1.,1.,1.,1.,1.,1.,1.,1.,1.,1.,1.,1.,1.,1.,1.,1.,1.,
1.,1.,1.,1.,1.,1.,1.,1.,1.,1.,1.,1.,1.,1.,1.,1.,1.,1.,1.,1.,1.,1.,1.,1.,
1.,1.,1.,1.,1.,1.))
REPRESENTATION_ITEM('')
);
#268=(
BOUNDED_CURVE()
B_SPLINE_CURVE(5,(#38935,#38936,#38937,#38938,#38939,#38940,#38941,#38942,
#38943,#38944,#38945,#38946,#38947,#38948,#38949,#38950,#38951,#38952,#38953,
#38954,#38955,#38956,#38957,#38958,#38959,#38960,#38961,#38962,#38963,#38964,
#38965,#38966,#38967,#38968,#38969,#38970,#38971,#38972,#38973,#38974,#38975,
#38976,#38977,#38978,#38979,#38980,#38981,#38982,#38983,#38984,#38985,#38986,
#38987,#38988,#38989,#38990,#38991,#38992,#38993,#38994,#38995,#38996,#38997,
#38998,#38999,#39000,#39001,#39002,#39003,#39004),.UNSPECIFIED.,.F.,.F.)
B_SPLINE_CURVE_WITH_KNOTS((6,1,1,1,1,1,1,1,1,1,1,1,1,1,1,1,1,1,1,1,1,1,
1,1,1,1,1,1,1,1,1,1,1,1,1,1,1,1,1,1,1,1,1,1,1,1,1,1,1,1,1,1,1,1,1,1,1,1,
1,1,1,1,1,1,1,6),(0.,0.0153846153846154,0.0307692307692308,0.0461538461538462,
0.0615384615384615,0.0769230769230769,0.0923076923076923,0.107692307692308,
0.123076923076923,0.138461538461538,0.153846153846154,0.169230769230769,
0.184615384615385,0.2,0.215384615384615,0.230769230769231,0.246153846153846,
0.261538461538462,0.276923076923077,0.292307692307692,0.307692307692308,
0.323076923076923,0.338461538461538,0.353846153846154,0.369230769230769,
0.384615384615385,0.4,0.415384615384615,0.430769230769231,0.446153846153846,
0.461538461538462,0.476923076923077,0.492307692307692,0.507692307692308,
0.523076923076923,0.538461538461538,0.553846153846154,0.569230769230769,
0.584615384615384,0.6,0.615384615384615,0.63076923076923,0.646153846153846,
0.661538461538461,0.676923076923076,0.692307692307692,0.707692307692307,
0.723076923076922,0.738461538461538,0.753846153846153,0.769230769230768,
0.784615384615384,0.799999999999999,0.815384615384614,0.83076923076923,
0.846153846153845,0.86153846153846,0.876923076923076,0.892307692307691,
0.907692307692306,0.923076923076922,0.938461538461537,0.953846153846152,
0.969230769230768,0.984615384615383,1.),.UNSPECIFIED.)
CURVE()
GEOMETRIC_REPRESENTATION_ITEM()
RATIONAL_B_SPLINE_CURVE((1.,1.,1.,1.,1.,1.,1.,1.,1.,1.,1.,1.,1.,1.,1.,1.,
1.,1.,1.,1.,1.,1.,1.,1.,1.,1.,1.,1.,1.,1.,1.,1.,1.,1.,1.,1.,1.,1.,1.,1.,
1.,1.,1.,1.,1.,1.,1.,1.,1.,1.,1.,1.,1.,1.,1.,1.,1.,1.,1.,1.,1.,1.,1.,1.,
1.,1.,1.,1.,1.,1.))
REPRESENTATION_ITEM('')
);
#269=(
BOUNDED_CURVE()
B_SPLINE_CURVE(5,(#39008,#39009,#39010,#39011,#39012,#39013,#39014,#39015,
#39016,#39017,#39018,#39019,#39020,#39021,#39022,#39023,#39024,#39025,#39026,
#39027,#39028,#39029,#39030,#39031,#39032,#39033,#39034,#39035,#39036,#39037,
#39038,#39039,#39040,#39041,#39042,#39043,#39044,#39045,#39046,#39047,#39048,
#39049,#39050,#39051,#39052,#39053,#39054,#39055,#39056,#39057,#39058,#39059,
#39060,#39061,#39062,#39063,#39064,#39065,#39066,#39067,#39068,#39069,#39070,
#39071,#39072,#39073,#39074,#39075,#39076,#39077),.UNSPECIFIED.,.F.,.F.)
B_SPLINE_CURVE_WITH_KNOTS((6,1,1,1,1,1,1,1,1,1,1,1,1,1,1,1,1,1,1,1,1,1,
1,1,1,1,1,1,1,1,1,1,1,1,1,1,1,1,1,1,1,1,1,1,1,1,1,1,1,1,1,1,1,1,1,1,1,1,
1,1,1,1,1,1,1,6),(0.,0.0153846153846154,0.0307692307692308,0.0461538461538462,
0.0615384615384615,0.0769230769230769,0.0923076923076923,0.107692307692308,
0.123076923076923,0.138461538461538,0.153846153846154,0.169230769230769,
0.184615384615385,0.2,0.215384615384615,0.230769230769231,0.246153846153846,
0.261538461538462,0.276923076923077,0.292307692307692,0.307692307692308,
0.323076923076923,0.338461538461538,0.353846153846154,0.369230769230769,
0.384615384615385,0.4,0.415384615384615,0.430769230769231,0.446153846153846,
0.461538461538462,0.476923076923077,0.492307692307692,0.507692307692308,
0.523076923076923,0.538461538461538,0.553846153846154,0.569230769230769,
0.584615384615384,0.6,0.615384615384615,0.63076923076923,0.646153846153846,
0.661538461538461,0.676923076923076,0.692307692307692,0.707692307692307,
0.723076923076922,0.738461538461538,0.753846153846153,0.769230769230768,
0.784615384615384,0.799999999999999,0.815384615384614,0.83076923076923,
0.846153846153845,0.86153846153846,0.876923076923076,0.892307692307691,
0.907692307692306,0.923076923076922,0.938461538461537,0.953846153846152,
0.969230769230768,0.984615384615383,1.),.UNSPECIFIED.)
CURVE()
GEOMETRIC_REPRESENTATION_ITEM()
RATIONAL_B_SPLINE_CURVE((1.,1.,1.,1.,1.,1.,1.,1.,1.,1.,1.,1.,1.,1.,1.,1.,
1.,1.,1.,1.,1.,1.,1.,1.,1.,1.,1.,1.,1.,1.,1.,1.,1.,1.,1.,1.,1.,1.,1.,1.,
1.,1.,1.,1.,1.,1.,1.,1.,1.,1.,1.,1.,1.,1.,1.,1.,1.,1.,1.,1.,1.,1.,1.,1.,
1.,1.,1.,1.,1.,1.))
REPRESENTATION_ITEM('')
);
#270=(
BOUNDED_CURVE()
B_SPLINE_CURVE(5,(#39081,#39082,#39083,#39084,#39085,#39086,#39087,#39088,
#39089,#39090,#39091,#39092,#39093,#39094,#39095,#39096,#39097,#39098,#39099,
#39100,#39101,#39102,#39103,#39104,#39105,#39106,#39107,#39108,#39109,#39110,
#39111,#39112,#39113,#39114,#39115,#39116,#39117,#39118,#39119,#39120,#39121,
#39122,#39123,#39124,#39125,#39126,#39127,#39128,#39129,#39130,#39131,#39132,
#39133,#39134,#39135,#39136,#39137,#39138,#39139,#39140,#39141,#39142,#39143,
#39144,#39145,#39146,#39147,#39148,#39149,#39150),.UNSPECIFIED.,.F.,.F.)
B_SPLINE_CURVE_WITH_KNOTS((6,1,1,1,1,1,1,1,1,1,1,1,1,1,1,1,1,1,1,1,1,1,
1,1,1,1,1,1,1,1,1,1,1,1,1,1,1,1,1,1,1,1,1,1,1,1,1,1,1,1,1,1,1,1,1,1,1,1,
1,1,1,1,1,1,1,6),(0.,0.0153846153846154,0.0307692307692308,0.0461538461538462,
0.0615384615384615,0.0769230769230769,0.0923076923076923,0.107692307692308,
0.123076923076923,0.138461538461538,0.153846153846154,0.169230769230769,
0.184615384615385,0.2,0.215384615384615,0.230769230769231,0.246153846153846,
0.261538461538462,0.276923076923077,0.292307692307692,0.307692307692308,
0.323076923076923,0.338461538461538,0.353846153846154,0.369230769230769,
0.384615384615385,0.4,0.415384615384615,0.430769230769231,0.446153846153846,
0.461538461538462,0.476923076923077,0.492307692307692,0.507692307692308,
0.523076923076923,0.538461538461538,0.553846153846154,0.569230769230769,
0.584615384615384,0.6,0.615384615384615,0.63076923076923,0.646153846153846,
0.661538461538461,0.676923076923076,0.692307692307692,0.707692307692307,
0.723076923076922,0.738461538461538,0.753846153846153,0.769230769230768,
0.784615384615384,0.799999999999999,0.815384615384614,0.83076923076923,
0.846153846153845,0.86153846153846,0.876923076923076,0.892307692307691,
0.907692307692306,0.923076923076922,0.938461538461537,0.953846153846152,
0.969230769230768,0.984615384615383,1.),.UNSPECIFIED.)
CURVE()
GEOMETRIC_REPRESENTATION_ITEM()
RATIONAL_B_SPLINE_CURVE((1.,1.,1.,1.,1.,1.,1.,1.,1.,1.,1.,1.,1.,1.,1.,1.,
1.,1.,1.,1.,1.,1.,1.,1.,1.,1.,1.,1.,1.,1.,1.,1.,1.,1.,1.,1.,1.,1.,1.,1.,
1.,1.,1.,1.,1.,1.,1.,1.,1.,1.,1.,1.,1.,1.,1.,1.,1.,1.,1.,1.,1.,1.,1.,1.,
1.,1.,1.,1.,1.,1.))
REPRESENTATION_ITEM('')
);
#271=(
BOUNDED_CURVE()
B_SPLINE_CURVE(5,(#39154,#39155,#39156,#39157,#39158,#39159,#39160,#39161,
#39162,#39163,#39164,#39165,#39166,#39167,#39168,#39169,#39170,#39171,#39172,
#39173,#39174,#39175,#39176,#39177,#39178,#39179,#39180,#39181,#39182,#39183,
#39184,#39185,#39186,#39187,#39188,#39189,#39190,#39191,#39192,#39193,#39194,
#39195,#39196,#39197,#39198,#39199,#39200,#39201,#39202,#39203,#39204,#39205,
#39206,#39207,#39208,#39209,#39210,#39211,#39212,#39213,#39214,#39215,#39216,
#39217,#39218,#39219,#39220,#39221,#39222,#39223),.UNSPECIFIED.,.F.,.F.)
B_SPLINE_CURVE_WITH_KNOTS((6,1,1,1,1,1,1,1,1,1,1,1,1,1,1,1,1,1,1,1,1,1,
1,1,1,1,1,1,1,1,1,1,1,1,1,1,1,1,1,1,1,1,1,1,1,1,1,1,1,1,1,1,1,1,1,1,1,1,
1,1,1,1,1,1,1,6),(0.,0.0153846153846154,0.0307692307692308,0.0461538461538462,
0.0615384615384615,0.0769230769230769,0.0923076923076923,0.107692307692308,
0.123076923076923,0.138461538461538,0.153846153846154,0.169230769230769,
0.184615384615385,0.2,0.215384615384615,0.230769230769231,0.246153846153846,
0.261538461538462,0.276923076923077,0.292307692307692,0.307692307692308,
0.323076923076923,0.338461538461538,0.353846153846154,0.369230769230769,
0.384615384615385,0.4,0.415384615384615,0.430769230769231,0.446153846153846,
0.461538461538462,0.476923076923077,0.492307692307692,0.507692307692308,
0.523076923076923,0.538461538461538,0.553846153846154,0.569230769230769,
0.584615384615384,0.6,0.615384615384615,0.63076923076923,0.646153846153846,
0.661538461538461,0.676923076923076,0.692307692307692,0.707692307692307,
0.723076923076922,0.738461538461538,0.753846153846153,0.769230769230768,
0.784615384615384,0.799999999999999,0.815384615384614,0.83076923076923,
0.846153846153845,0.86153846153846,0.876923076923076,0.892307692307691,
0.907692307692306,0.923076923076922,0.938461538461537,0.953846153846152,
0.969230769230768,0.984615384615383,1.),.UNSPECIFIED.)
CURVE()
GEOMETRIC_REPRESENTATION_ITEM()
RATIONAL_B_SPLINE_CURVE((1.,1.,1.,1.,1.,1.,1.,1.,1.,1.,1.,1.,1.,1.,1.,1.,
1.,1.,1.,1.,1.,1.,1.,1.,1.,1.,1.,1.,1.,1.,1.,1.,1.,1.,1.,1.,1.,1.,1.,1.,
1.,1.,1.,1.,1.,1.,1.,1.,1.,1.,1.,1.,1.,1.,1.,1.,1.,1.,1.,1.,1.,1.,1.,1.,
1.,1.,1.,1.,1.,1.))
REPRESENTATION_ITEM('')
);
#272=(
BOUNDED_CURVE()
B_SPLINE_CURVE(5,(#39227,#39228,#39229,#39230,#39231,#39232,#39233,#39234,
#39235,#39236,#39237,#39238,#39239,#39240,#39241,#39242,#39243,#39244,#39245,
#39246,#39247,#39248,#39249,#39250,#39251,#39252,#39253,#39254,#39255,#39256,
#39257,#39258,#39259,#39260,#39261,#39262,#39263,#39264,#39265,#39266,#39267,
#39268,#39269,#39270,#39271,#39272,#39273,#39274,#39275,#39276,#39277,#39278,
#39279,#39280,#39281,#39282,#39283,#39284,#39285,#39286,#39287,#39288,#39289,
#39290,#39291,#39292,#39293,#39294,#39295,#39296),.UNSPECIFIED.,.F.,.F.)
B_SPLINE_CURVE_WITH_KNOTS((6,1,1,1,1,1,1,1,1,1,1,1,1,1,1,1,1,1,1,1,1,1,
1,1,1,1,1,1,1,1,1,1,1,1,1,1,1,1,1,1,1,1,1,1,1,1,1,1,1,1,1,1,1,1,1,1,1,1,
1,1,1,1,1,1,1,6),(0.,0.0153846153846154,0.0307692307692308,0.0461538461538462,
0.0615384615384615,0.0769230769230769,0.0923076923076923,0.107692307692308,
0.123076923076923,0.138461538461538,0.153846153846154,0.169230769230769,
0.184615384615385,0.2,0.215384615384615,0.230769230769231,0.246153846153846,
0.261538461538462,0.276923076923077,0.292307692307692,0.307692307692308,
0.323076923076923,0.338461538461538,0.353846153846154,0.369230769230769,
0.384615384615385,0.4,0.415384615384615,0.430769230769231,0.446153846153846,
0.461538461538462,0.476923076923077,0.492307692307692,0.507692307692308,
0.523076923076923,0.538461538461538,0.553846153846154,0.569230769230769,
0.584615384615384,0.6,0.615384615384615,0.63076923076923,0.646153846153846,
0.661538461538461,0.676923076923076,0.692307692307692,0.707692307692307,
0.723076923076922,0.738461538461538,0.753846153846153,0.769230769230768,
0.784615384615384,0.799999999999999,0.815384615384614,0.83076923076923,
0.846153846153845,0.86153846153846,0.876923076923076,0.892307692307691,
0.907692307692306,0.923076923076922,0.938461538461537,0.953846153846152,
0.969230769230768,0.984615384615383,1.),.UNSPECIFIED.)
CURVE()
GEOMETRIC_REPRESENTATION_ITEM()
RATIONAL_B_SPLINE_CURVE((1.,1.,1.,1.,1.,1.,1.,1.,1.,1.,1.,1.,1.,1.,1.,1.,
1.,1.,1.,1.,1.,1.,1.,1.,1.,1.,1.,1.,1.,1.,1.,1.,1.,1.,1.,1.,1.,1.,1.,1.,
1.,1.,1.,1.,1.,1.,1.,1.,1.,1.,1.,1.,1.,1.,1.,1.,1.,1.,1.,1.,1.,1.,1.,1.,
1.,1.,1.,1.,1.,1.))
REPRESENTATION_ITEM('')
);
#273=(
BOUNDED_CURVE()
B_SPLINE_CURVE(5,(#39300,#39301,#39302,#39303,#39304,#39305,#39306,#39307,
#39308,#39309,#39310,#39311,#39312,#39313,#39314,#39315,#39316,#39317,#39318,
#39319,#39320,#39321,#39322,#39323,#39324,#39325,#39326,#39327,#39328,#39329,
#39330,#39331,#39332,#39333,#39334,#39335,#39336,#39337,#39338,#39339,#39340,
#39341,#39342,#39343,#39344,#39345,#39346,#39347,#39348,#39349,#39350,#39351,
#39352,#39353,#39354,#39355,#39356,#39357,#39358,#39359,#39360,#39361,#39362,
#39363,#39364,#39365,#39366,#39367,#39368,#39369),.UNSPECIFIED.,.F.,.F.)
B_SPLINE_CURVE_WITH_KNOTS((6,1,1,1,1,1,1,1,1,1,1,1,1,1,1,1,1,1,1,1,1,1,
1,1,1,1,1,1,1,1,1,1,1,1,1,1,1,1,1,1,1,1,1,1,1,1,1,1,1,1,1,1,1,1,1,1,1,1,
1,1,1,1,1,1,1,6),(0.,0.0153846153846154,0.0307692307692308,0.0461538461538462,
0.0615384615384615,0.0769230769230769,0.0923076923076923,0.107692307692308,
0.123076923076923,0.138461538461538,0.153846153846154,0.169230769230769,
0.184615384615385,0.2,0.215384615384615,0.230769230769231,0.246153846153846,
0.261538461538462,0.276923076923077,0.292307692307692,0.307692307692308,
0.323076923076923,0.338461538461538,0.353846153846154,0.369230769230769,
0.384615384615385,0.4,0.415384615384615,0.430769230769231,0.446153846153846,
0.461538461538462,0.476923076923077,0.492307692307692,0.507692307692308,
0.523076923076923,0.538461538461538,0.553846153846154,0.569230769230769,
0.584615384615384,0.6,0.615384615384615,0.63076923076923,0.646153846153846,
0.661538461538461,0.676923076923076,0.692307692307692,0.707692307692307,
0.723076923076922,0.738461538461538,0.753846153846153,0.769230769230768,
0.784615384615384,0.799999999999999,0.815384615384614,0.83076923076923,
0.846153846153845,0.86153846153846,0.876923076923076,0.892307692307691,
0.907692307692306,0.923076923076922,0.938461538461537,0.953846153846152,
0.969230769230768,0.984615384615383,1.),.UNSPECIFIED.)
CURVE()
GEOMETRIC_REPRESENTATION_ITEM()
RATIONAL_B_SPLINE_CURVE((1.,1.,1.,1.,1.,1.,1.,1.,1.,1.,1.,1.,1.,1.,1.,1.,
1.,1.,1.,1.,1.,1.,1.,1.,1.,1.,1.,1.,1.,1.,1.,1.,1.,1.,1.,1.,1.,1.,1.,1.,
1.,1.,1.,1.,1.,1.,1.,1.,1.,1.,1.,1.,1.,1.,1.,1.,1.,1.,1.,1.,1.,1.,1.,1.,
1.,1.,1.,1.,1.,1.))
REPRESENTATION_ITEM('')
);
#274=(
BOUNDED_CURVE()
B_SPLINE_CURVE(5,(#39373,#39374,#39375,#39376,#39377,#39378,#39379,#39380,
#39381,#39382,#39383,#39384,#39385,#39386,#39387,#39388,#39389,#39390,#39391,
#39392,#39393,#39394,#39395,#39396,#39397,#39398,#39399,#39400,#39401,#39402,
#39403,#39404,#39405,#39406,#39407,#39408,#39409,#39410,#39411,#39412,#39413,
#39414,#39415,#39416,#39417,#39418,#39419,#39420,#39421,#39422,#39423,#39424,
#39425,#39426,#39427,#39428,#39429,#39430,#39431,#39432,#39433,#39434,#39435,
#39436,#39437,#39438,#39439,#39440,#39441,#39442),.UNSPECIFIED.,.F.,.F.)
B_SPLINE_CURVE_WITH_KNOTS((6,1,1,1,1,1,1,1,1,1,1,1,1,1,1,1,1,1,1,1,1,1,
1,1,1,1,1,1,1,1,1,1,1,1,1,1,1,1,1,1,1,1,1,1,1,1,1,1,1,1,1,1,1,1,1,1,1,1,
1,1,1,1,1,1,1,6),(0.,0.0153846153846154,0.0307692307692308,0.0461538461538462,
0.0615384615384615,0.0769230769230769,0.0923076923076923,0.107692307692308,
0.123076923076923,0.138461538461538,0.153846153846154,0.169230769230769,
0.184615384615385,0.2,0.215384615384615,0.230769230769231,0.246153846153846,
0.261538461538462,0.276923076923077,0.292307692307692,0.307692307692308,
0.323076923076923,0.338461538461538,0.353846153846154,0.369230769230769,
0.384615384615385,0.4,0.415384615384615,0.430769230769231,0.446153846153846,
0.461538461538462,0.476923076923077,0.492307692307692,0.507692307692308,
0.523076923076923,0.538461538461538,0.553846153846154,0.569230769230769,
0.584615384615384,0.6,0.615384615384615,0.63076923076923,0.646153846153846,
0.661538461538461,0.676923076923076,0.692307692307692,0.707692307692307,
0.723076923076922,0.738461538461538,0.753846153846153,0.769230769230768,
0.784615384615384,0.799999999999999,0.815384615384614,0.83076923076923,
0.846153846153845,0.86153846153846,0.876923076923076,0.892307692307691,
0.907692307692306,0.923076923076922,0.938461538461537,0.953846153846152,
0.969230769230768,0.984615384615383,1.),.UNSPECIFIED.)
CURVE()
GEOMETRIC_REPRESENTATION_ITEM()
RATIONAL_B_SPLINE_CURVE((1.,1.,1.,1.,1.,1.,1.,1.,1.,1.,1.,1.,1.,1.,1.,1.,
1.,1.,1.,1.,1.,1.,1.,1.,1.,1.,1.,1.,1.,1.,1.,1.,1.,1.,1.,1.,1.,1.,1.,1.,
1.,1.,1.,1.,1.,1.,1.,1.,1.,1.,1.,1.,1.,1.,1.,1.,1.,1.,1.,1.,1.,1.,1.,1.,
1.,1.,1.,1.,1.,1.))
REPRESENTATION_ITEM('')
);
#275=(
BOUNDED_CURVE()
B_SPLINE_CURVE(5,(#39446,#39447,#39448,#39449,#39450,#39451,#39452,#39453,
#39454,#39455,#39456,#39457,#39458,#39459,#39460,#39461,#39462,#39463,#39464,
#39465,#39466,#39467,#39468,#39469,#39470,#39471,#39472,#39473,#39474,#39475,
#39476,#39477,#39478,#39479,#39480,#39481,#39482,#39483,#39484,#39485,#39486,
#39487,#39488,#39489,#39490,#39491,#39492,#39493,#39494,#39495,#39496,#39497,
#39498,#39499,#39500,#39501,#39502,#39503,#39504,#39505,#39506,#39507,#39508,
#39509,#39510,#39511,#39512,#39513,#39514,#39515),.UNSPECIFIED.,.F.,.F.)
B_SPLINE_CURVE_WITH_KNOTS((6,1,1,1,1,1,1,1,1,1,1,1,1,1,1,1,1,1,1,1,1,1,
1,1,1,1,1,1,1,1,1,1,1,1,1,1,1,1,1,1,1,1,1,1,1,1,1,1,1,1,1,1,1,1,1,1,1,1,
1,1,1,1,1,1,1,6),(0.,0.0153846153846154,0.0307692307692308,0.0461538461538462,
0.0615384615384615,0.0769230769230769,0.0923076923076923,0.107692307692308,
0.123076923076923,0.138461538461538,0.153846153846154,0.169230769230769,
0.184615384615385,0.2,0.215384615384615,0.230769230769231,0.246153846153846,
0.261538461538462,0.276923076923077,0.292307692307692,0.307692307692308,
0.323076923076923,0.338461538461538,0.353846153846154,0.369230769230769,
0.384615384615385,0.4,0.415384615384615,0.430769230769231,0.446153846153846,
0.461538461538462,0.476923076923077,0.492307692307692,0.507692307692308,
0.523076923076923,0.538461538461538,0.553846153846154,0.569230769230769,
0.584615384615384,0.6,0.615384615384615,0.63076923076923,0.646153846153846,
0.661538461538461,0.676923076923076,0.692307692307692,0.707692307692307,
0.723076923076922,0.738461538461538,0.753846153846153,0.769230769230768,
0.784615384615384,0.799999999999999,0.815384615384614,0.83076923076923,
0.846153846153845,0.86153846153846,0.876923076923076,0.892307692307691,
0.907692307692306,0.923076923076922,0.938461538461537,0.953846153846152,
0.969230769230768,0.984615384615383,1.),.UNSPECIFIED.)
CURVE()
GEOMETRIC_REPRESENTATION_ITEM()
RATIONAL_B_SPLINE_CURVE((1.,1.,1.,1.,1.,1.,1.,1.,1.,1.,1.,1.,1.,1.,1.,1.,
1.,1.,1.,1.,1.,1.,1.,1.,1.,1.,1.,1.,1.,1.,1.,1.,1.,1.,1.,1.,1.,1.,1.,1.,
1.,1.,1.,1.,1.,1.,1.,1.,1.,1.,1.,1.,1.,1.,1.,1.,1.,1.,1.,1.,1.,1.,1.,1.,
1.,1.,1.,1.,1.,1.))
REPRESENTATION_ITEM('')
);
#276=(
BOUNDED_CURVE()
B_SPLINE_CURVE(5,(#39519,#39520,#39521,#39522,#39523,#39524,#39525,#39526,
#39527,#39528,#39529,#39530,#39531,#39532,#39533,#39534,#39535,#39536,#39537,
#39538,#39539,#39540,#39541,#39542,#39543,#39544,#39545,#39546,#39547,#39548,
#39549,#39550,#39551,#39552,#39553,#39554,#39555,#39556,#39557,#39558,#39559,
#39560,#39561,#39562,#39563,#39564,#39565,#39566,#39567,#39568,#39569,#39570,
#39571,#39572,#39573,#39574,#39575,#39576,#39577,#39578,#39579,#39580,#39581,
#39582,#39583,#39584,#39585,#39586,#39587,#39588),.UNSPECIFIED.,.F.,.F.)
B_SPLINE_CURVE_WITH_KNOTS((6,1,1,1,1,1,1,1,1,1,1,1,1,1,1,1,1,1,1,1,1,1,
1,1,1,1,1,1,1,1,1,1,1,1,1,1,1,1,1,1,1,1,1,1,1,1,1,1,1,1,1,1,1,1,1,1,1,1,
1,1,1,1,1,1,1,6),(0.,0.0153846153846154,0.0307692307692308,0.0461538461538462,
0.0615384615384615,0.0769230769230769,0.0923076923076923,0.107692307692308,
0.123076923076923,0.138461538461538,0.153846153846154,0.169230769230769,
0.184615384615385,0.2,0.215384615384615,0.230769230769231,0.246153846153846,
0.261538461538462,0.276923076923077,0.292307692307692,0.307692307692308,
0.323076923076923,0.338461538461538,0.353846153846154,0.369230769230769,
0.384615384615385,0.4,0.415384615384615,0.430769230769231,0.446153846153846,
0.461538461538462,0.476923076923077,0.492307692307692,0.507692307692308,
0.523076923076923,0.538461538461538,0.553846153846154,0.569230769230769,
0.584615384615384,0.6,0.615384615384615,0.63076923076923,0.646153846153846,
0.661538461538461,0.676923076923076,0.692307692307692,0.707692307692307,
0.723076923076922,0.738461538461538,0.753846153846153,0.769230769230768,
0.784615384615384,0.799999999999999,0.815384615384614,0.83076923076923,
0.846153846153845,0.86153846153846,0.876923076923076,0.892307692307691,
0.907692307692306,0.923076923076922,0.938461538461537,0.953846153846152,
0.969230769230768,0.984615384615383,1.),.UNSPECIFIED.)
CURVE()
GEOMETRIC_REPRESENTATION_ITEM()
RATIONAL_B_SPLINE_CURVE((1.,1.,1.,1.,1.,1.,1.,1.,1.,1.,1.,1.,1.,1.,1.,1.,
1.,1.,1.,1.,1.,1.,1.,1.,1.,1.,1.,1.,1.,1.,1.,1.,1.,1.,1.,1.,1.,1.,1.,1.,
1.,1.,1.,1.,1.,1.,1.,1.,1.,1.,1.,1.,1.,1.,1.,1.,1.,1.,1.,1.,1.,1.,1.,1.,
1.,1.,1.,1.,1.,1.))
REPRESENTATION_ITEM('')
);
#277=(
BOUNDED_CURVE()
B_SPLINE_CURVE(5,(#39592,#39593,#39594,#39595,#39596,#39597,#39598,#39599,
#39600,#39601,#39602,#39603,#39604,#39605,#39606,#39607,#39608,#39609,#39610,
#39611,#39612,#39613,#39614,#39615,#39616,#39617,#39618,#39619,#39620,#39621,
#39622,#39623,#39624,#39625,#39626,#39627,#39628,#39629,#39630,#39631,#39632,
#39633,#39634,#39635,#39636,#39637,#39638,#39639,#39640,#39641,#39642,#39643,
#39644,#39645,#39646,#39647,#39648,#39649,#39650,#39651,#39652,#39653,#39654,
#39655,#39656,#39657,#39658,#39659,#39660,#39661),.UNSPECIFIED.,.F.,.F.)
B_SPLINE_CURVE_WITH_KNOTS((6,1,1,1,1,1,1,1,1,1,1,1,1,1,1,1,1,1,1,1,1,1,
1,1,1,1,1,1,1,1,1,1,1,1,1,1,1,1,1,1,1,1,1,1,1,1,1,1,1,1,1,1,1,1,1,1,1,1,
1,1,1,1,1,1,1,6),(0.,0.0153846153846154,0.0307692307692308,0.0461538461538462,
0.0615384615384615,0.0769230769230769,0.0923076923076923,0.107692307692308,
0.123076923076923,0.138461538461538,0.153846153846154,0.169230769230769,
0.184615384615385,0.2,0.215384615384615,0.230769230769231,0.246153846153846,
0.261538461538462,0.276923076923077,0.292307692307692,0.307692307692308,
0.323076923076923,0.338461538461538,0.353846153846154,0.369230769230769,
0.384615384615385,0.4,0.415384615384615,0.430769230769231,0.446153846153846,
0.461538461538462,0.476923076923077,0.492307692307692,0.507692307692308,
0.523076923076923,0.538461538461538,0.553846153846154,0.569230769230769,
0.584615384615384,0.6,0.615384615384615,0.63076923076923,0.646153846153846,
0.661538461538461,0.676923076923076,0.692307692307692,0.707692307692307,
0.723076923076922,0.738461538461538,0.753846153846153,0.769230769230768,
0.784615384615384,0.799999999999999,0.815384615384614,0.83076923076923,
0.846153846153845,0.86153846153846,0.876923076923076,0.892307692307691,
0.907692307692306,0.923076923076922,0.938461538461537,0.953846153846152,
0.969230769230768,0.984615384615383,1.),.UNSPECIFIED.)
CURVE()
GEOMETRIC_REPRESENTATION_ITEM()
RATIONAL_B_SPLINE_CURVE((1.,1.,1.,1.,1.,1.,1.,1.,1.,1.,1.,1.,1.,1.,1.,1.,
1.,1.,1.,1.,1.,1.,1.,1.,1.,1.,1.,1.,1.,1.,1.,1.,1.,1.,1.,1.,1.,1.,1.,1.,
1.,1.,1.,1.,1.,1.,1.,1.,1.,1.,1.,1.,1.,1.,1.,1.,1.,1.,1.,1.,1.,1.,1.,1.,
1.,1.,1.,1.,1.,1.))
REPRESENTATION_ITEM('')
);
#278=(
BOUNDED_CURVE()
B_SPLINE_CURVE(5,(#39665,#39666,#39667,#39668,#39669,#39670,#39671,#39672,
#39673,#39674,#39675,#39676,#39677,#39678,#39679,#39680,#39681,#39682,#39683,
#39684,#39685,#39686,#39687,#39688,#39689,#39690,#39691,#39692,#39693,#39694,
#39695,#39696,#39697,#39698,#39699,#39700,#39701,#39702,#39703,#39704,#39705,
#39706,#39707,#39708,#39709,#39710,#39711,#39712,#39713,#39714,#39715,#39716,
#39717,#39718,#39719,#39720,#39721,#39722,#39723,#39724,#39725,#39726,#39727,
#39728,#39729,#39730,#39731,#39732,#39733,#39734),.UNSPECIFIED.,.F.,.F.)
B_SPLINE_CURVE_WITH_KNOTS((6,1,1,1,1,1,1,1,1,1,1,1,1,1,1,1,1,1,1,1,1,1,
1,1,1,1,1,1,1,1,1,1,1,1,1,1,1,1,1,1,1,1,1,1,1,1,1,1,1,1,1,1,1,1,1,1,1,1,
1,1,1,1,1,1,1,6),(0.,0.0153846153846154,0.0307692307692308,0.0461538461538462,
0.0615384615384615,0.0769230769230769,0.0923076923076923,0.107692307692308,
0.123076923076923,0.138461538461538,0.153846153846154,0.169230769230769,
0.184615384615385,0.2,0.215384615384615,0.230769230769231,0.246153846153846,
0.261538461538462,0.276923076923077,0.292307692307692,0.307692307692308,
0.323076923076923,0.338461538461538,0.353846153846154,0.369230769230769,
0.384615384615385,0.4,0.415384615384615,0.430769230769231,0.446153846153846,
0.461538461538462,0.476923076923077,0.492307692307692,0.507692307692308,
0.523076923076923,0.538461538461538,0.553846153846154,0.569230769230769,
0.584615384615384,0.6,0.615384615384615,0.63076923076923,0.646153846153846,
0.661538461538461,0.676923076923076,0.692307692307692,0.707692307692307,
0.723076923076922,0.738461538461538,0.753846153846153,0.769230769230768,
0.784615384615384,0.799999999999999,0.815384615384614,0.83076923076923,
0.846153846153845,0.86153846153846,0.876923076923076,0.892307692307691,
0.907692307692306,0.923076923076922,0.938461538461537,0.953846153846152,
0.969230769230768,0.984615384615383,1.),.UNSPECIFIED.)
CURVE()
GEOMETRIC_REPRESENTATION_ITEM()
RATIONAL_B_SPLINE_CURVE((1.,1.,1.,1.,1.,1.,1.,1.,1.,1.,1.,1.,1.,1.,1.,1.,
1.,1.,1.,1.,1.,1.,1.,1.,1.,1.,1.,1.,1.,1.,1.,1.,1.,1.,1.,1.,1.,1.,1.,1.,
1.,1.,1.,1.,1.,1.,1.,1.,1.,1.,1.,1.,1.,1.,1.,1.,1.,1.,1.,1.,1.,1.,1.,1.,
1.,1.,1.,1.,1.,1.))
REPRESENTATION_ITEM('')
);
#279=(
BOUNDED_CURVE()
B_SPLINE_CURVE(5,(#39738,#39739,#39740,#39741,#39742,#39743,#39744,#39745,
#39746,#39747,#39748,#39749,#39750,#39751,#39752,#39753,#39754,#39755,#39756,
#39757,#39758,#39759,#39760,#39761,#39762,#39763,#39764,#39765,#39766,#39767,
#39768,#39769,#39770,#39771,#39772,#39773,#39774,#39775,#39776,#39777,#39778,
#39779,#39780,#39781,#39782,#39783,#39784,#39785,#39786,#39787,#39788,#39789,
#39790,#39791,#39792,#39793,#39794,#39795,#39796,#39797,#39798,#39799,#39800,
#39801,#39802,#39803,#39804,#39805,#39806,#39807),.UNSPECIFIED.,.F.,.F.)
B_SPLINE_CURVE_WITH_KNOTS((6,1,1,1,1,1,1,1,1,1,1,1,1,1,1,1,1,1,1,1,1,1,
1,1,1,1,1,1,1,1,1,1,1,1,1,1,1,1,1,1,1,1,1,1,1,1,1,1,1,1,1,1,1,1,1,1,1,1,
1,1,1,1,1,1,1,6),(0.,0.0153846153846154,0.0307692307692308,0.0461538461538462,
0.0615384615384615,0.0769230769230769,0.0923076923076923,0.107692307692308,
0.123076923076923,0.138461538461538,0.153846153846154,0.169230769230769,
0.184615384615385,0.2,0.215384615384615,0.230769230769231,0.246153846153846,
0.261538461538462,0.276923076923077,0.292307692307692,0.307692307692308,
0.323076923076923,0.338461538461538,0.353846153846154,0.369230769230769,
0.384615384615385,0.4,0.415384615384615,0.430769230769231,0.446153846153846,
0.461538461538462,0.476923076923077,0.492307692307692,0.507692307692308,
0.523076923076923,0.538461538461538,0.553846153846154,0.569230769230769,
0.584615384615384,0.6,0.615384615384615,0.63076923076923,0.646153846153846,
0.661538461538461,0.676923076923076,0.692307692307692,0.707692307692307,
0.723076923076922,0.738461538461538,0.753846153846153,0.769230769230768,
0.784615384615384,0.799999999999999,0.815384615384614,0.83076923076923,
0.846153846153845,0.86153846153846,0.876923076923076,0.892307692307691,
0.907692307692306,0.923076923076922,0.938461538461537,0.953846153846152,
0.969230769230768,0.984615384615383,1.),.UNSPECIFIED.)
CURVE()
GEOMETRIC_REPRESENTATION_ITEM()
RATIONAL_B_SPLINE_CURVE((1.,1.,1.,1.,1.,1.,1.,1.,1.,1.,1.,1.,1.,1.,1.,1.,
1.,1.,1.,1.,1.,1.,1.,1.,1.,1.,1.,1.,1.,1.,1.,1.,1.,1.,1.,1.,1.,1.,1.,1.,
1.,1.,1.,1.,1.,1.,1.,1.,1.,1.,1.,1.,1.,1.,1.,1.,1.,1.,1.,1.,1.,1.,1.,1.,
1.,1.,1.,1.,1.,1.))
REPRESENTATION_ITEM('')
);
#280=(
BOUNDED_CURVE()
B_SPLINE_CURVE(5,(#39811,#39812,#39813,#39814,#39815,#39816,#39817,#39818,
#39819,#39820,#39821,#39822,#39823,#39824,#39825,#39826,#39827,#39828,#39829,
#39830,#39831,#39832,#39833,#39834,#39835,#39836,#39837,#39838,#39839,#39840,
#39841,#39842,#39843,#39844,#39845,#39846,#39847,#39848,#39849,#39850,#39851,
#39852,#39853,#39854,#39855,#39856,#39857,#39858,#39859,#39860,#39861,#39862,
#39863,#39864,#39865,#39866,#39867,#39868,#39869,#39870,#39871,#39872,#39873,
#39874,#39875,#39876,#39877,#39878,#39879,#39880),.UNSPECIFIED.,.F.,.F.)
B_SPLINE_CURVE_WITH_KNOTS((6,1,1,1,1,1,1,1,1,1,1,1,1,1,1,1,1,1,1,1,1,1,
1,1,1,1,1,1,1,1,1,1,1,1,1,1,1,1,1,1,1,1,1,1,1,1,1,1,1,1,1,1,1,1,1,1,1,1,
1,1,1,1,1,1,1,6),(0.,0.0153846153846154,0.0307692307692308,0.0461538461538462,
0.0615384615384615,0.0769230769230769,0.0923076923076923,0.107692307692308,
0.123076923076923,0.138461538461538,0.153846153846154,0.169230769230769,
0.184615384615385,0.2,0.215384615384615,0.230769230769231,0.246153846153846,
0.261538461538462,0.276923076923077,0.292307692307692,0.307692307692308,
0.323076923076923,0.338461538461538,0.353846153846154,0.369230769230769,
0.384615384615385,0.4,0.415384615384615,0.430769230769231,0.446153846153846,
0.461538461538462,0.476923076923077,0.492307692307692,0.507692307692308,
0.523076923076923,0.538461538461538,0.553846153846154,0.569230769230769,
0.584615384615384,0.6,0.615384615384615,0.63076923076923,0.646153846153846,
0.661538461538461,0.676923076923076,0.692307692307692,0.707692307692307,
0.723076923076922,0.738461538461538,0.753846153846153,0.769230769230768,
0.784615384615384,0.799999999999999,0.815384615384614,0.83076923076923,
0.846153846153845,0.86153846153846,0.876923076923076,0.892307692307691,
0.907692307692306,0.923076923076922,0.938461538461537,0.953846153846152,
0.969230769230768,0.984615384615383,1.),.UNSPECIFIED.)
CURVE()
GEOMETRIC_REPRESENTATION_ITEM()
RATIONAL_B_SPLINE_CURVE((1.,1.,1.,1.,1.,1.,1.,1.,1.,1.,1.,1.,1.,1.,1.,1.,
1.,1.,1.,1.,1.,1.,1.,1.,1.,1.,1.,1.,1.,1.,1.,1.,1.,1.,1.,1.,1.,1.,1.,1.,
1.,1.,1.,1.,1.,1.,1.,1.,1.,1.,1.,1.,1.,1.,1.,1.,1.,1.,1.,1.,1.,1.,1.,1.,
1.,1.,1.,1.,1.,1.))
REPRESENTATION_ITEM('')
);
#281=(
BOUNDED_CURVE()
B_SPLINE_CURVE(5,(#39884,#39885,#39886,#39887,#39888,#39889,#39890,#39891,
#39892,#39893,#39894,#39895,#39896,#39897,#39898,#39899,#39900,#39901,#39902,
#39903,#39904,#39905,#39906,#39907,#39908,#39909,#39910,#39911,#39912,#39913,
#39914,#39915,#39916,#39917,#39918,#39919,#39920,#39921,#39922,#39923,#39924,
#39925,#39926,#39927,#39928,#39929,#39930,#39931,#39932,#39933,#39934,#39935,
#39936,#39937,#39938,#39939,#39940,#39941,#39942,#39943,#39944,#39945,#39946,
#39947,#39948,#39949,#39950,#39951,#39952,#39953),.UNSPECIFIED.,.F.,.F.)
B_SPLINE_CURVE_WITH_KNOTS((6,1,1,1,1,1,1,1,1,1,1,1,1,1,1,1,1,1,1,1,1,1,
1,1,1,1,1,1,1,1,1,1,1,1,1,1,1,1,1,1,1,1,1,1,1,1,1,1,1,1,1,1,1,1,1,1,1,1,
1,1,1,1,1,1,1,6),(0.,0.0153846153846154,0.0307692307692308,0.0461538461538462,
0.0615384615384615,0.0769230769230769,0.0923076923076923,0.107692307692308,
0.123076923076923,0.138461538461538,0.153846153846154,0.169230769230769,
0.184615384615385,0.2,0.215384615384615,0.230769230769231,0.246153846153846,
0.261538461538462,0.276923076923077,0.292307692307692,0.307692307692308,
0.323076923076923,0.338461538461538,0.353846153846154,0.369230769230769,
0.384615384615385,0.4,0.415384615384615,0.430769230769231,0.446153846153846,
0.461538461538462,0.476923076923077,0.492307692307692,0.507692307692308,
0.523076923076923,0.538461538461538,0.553846153846154,0.569230769230769,
0.584615384615384,0.6,0.615384615384615,0.63076923076923,0.646153846153846,
0.661538461538461,0.676923076923076,0.692307692307692,0.707692307692307,
0.723076923076922,0.738461538461538,0.753846153846153,0.769230769230768,
0.784615384615384,0.799999999999999,0.815384615384614,0.83076923076923,
0.846153846153845,0.86153846153846,0.876923076923076,0.892307692307691,
0.907692307692306,0.923076923076922,0.938461538461537,0.953846153846152,
0.969230769230768,0.984615384615383,1.),.UNSPECIFIED.)
CURVE()
GEOMETRIC_REPRESENTATION_ITEM()
RATIONAL_B_SPLINE_CURVE((1.,1.,1.,1.,1.,1.,1.,1.,1.,1.,1.,1.,1.,1.,1.,1.,
1.,1.,1.,1.,1.,1.,1.,1.,1.,1.,1.,1.,1.,1.,1.,1.,1.,1.,1.,1.,1.,1.,1.,1.,
1.,1.,1.,1.,1.,1.,1.,1.,1.,1.,1.,1.,1.,1.,1.,1.,1.,1.,1.,1.,1.,1.,1.,1.,
1.,1.,1.,1.,1.,1.))
REPRESENTATION_ITEM('')
);
#282=(
BOUNDED_CURVE()
B_SPLINE_CURVE(5,(#39957,#39958,#39959,#39960,#39961,#39962,#39963,#39964,
#39965,#39966,#39967,#39968,#39969,#39970,#39971,#39972,#39973,#39974,#39975,
#39976,#39977,#39978,#39979,#39980,#39981,#39982,#39983,#39984,#39985,#39986,
#39987,#39988,#39989,#39990,#39991,#39992,#39993,#39994,#39995,#39996,#39997,
#39998,#39999,#40000,#40001,#40002,#40003,#40004,#40005,#40006,#40007,#40008,
#40009,#40010,#40011,#40012,#40013,#40014,#40015,#40016,#40017,#40018,#40019,
#40020,#40021,#40022,#40023,#40024,#40025,#40026),.UNSPECIFIED.,.F.,.F.)
B_SPLINE_CURVE_WITH_KNOTS((6,1,1,1,1,1,1,1,1,1,1,1,1,1,1,1,1,1,1,1,1,1,
1,1,1,1,1,1,1,1,1,1,1,1,1,1,1,1,1,1,1,1,1,1,1,1,1,1,1,1,1,1,1,1,1,1,1,1,
1,1,1,1,1,1,1,6),(0.,0.0153846153846154,0.0307692307692308,0.0461538461538462,
0.0615384615384615,0.0769230769230769,0.0923076923076923,0.107692307692308,
0.123076923076923,0.138461538461538,0.153846153846154,0.169230769230769,
0.184615384615385,0.2,0.215384615384615,0.230769230769231,0.246153846153846,
0.261538461538462,0.276923076923077,0.292307692307692,0.307692307692308,
0.323076923076923,0.338461538461538,0.353846153846154,0.369230769230769,
0.384615384615385,0.4,0.415384615384615,0.430769230769231,0.446153846153846,
0.461538461538462,0.476923076923077,0.492307692307692,0.507692307692308,
0.523076923076923,0.538461538461538,0.553846153846154,0.569230769230769,
0.584615384615384,0.6,0.615384615384615,0.63076923076923,0.646153846153846,
0.661538461538461,0.676923076923076,0.692307692307692,0.707692307692307,
0.723076923076922,0.738461538461538,0.753846153846153,0.769230769230768,
0.784615384615384,0.799999999999999,0.815384615384614,0.83076923076923,
0.846153846153845,0.86153846153846,0.876923076923076,0.892307692307691,
0.907692307692306,0.923076923076922,0.938461538461537,0.953846153846152,
0.969230769230768,0.984615384615383,1.),.UNSPECIFIED.)
CURVE()
GEOMETRIC_REPRESENTATION_ITEM()
RATIONAL_B_SPLINE_CURVE((1.,1.,1.,1.,1.,1.,1.,1.,1.,1.,1.,1.,1.,1.,1.,1.,
1.,1.,1.,1.,1.,1.,1.,1.,1.,1.,1.,1.,1.,1.,1.,1.,1.,1.,1.,1.,1.,1.,1.,1.,
1.,1.,1.,1.,1.,1.,1.,1.,1.,1.,1.,1.,1.,1.,1.,1.,1.,1.,1.,1.,1.,1.,1.,1.,
1.,1.,1.,1.,1.,1.))
REPRESENTATION_ITEM('')
);
#283=(
BOUNDED_CURVE()
B_SPLINE_CURVE(5,(#40030,#40031,#40032,#40033,#40034,#40035,#40036,#40037,
#40038,#40039,#40040,#40041,#40042,#40043,#40044,#40045,#40046,#40047,#40048,
#40049,#40050,#40051,#40052,#40053,#40054,#40055,#40056,#40057,#40058,#40059,
#40060,#40061,#40062,#40063,#40064,#40065,#40066,#40067,#40068,#40069,#40070,
#40071,#40072,#40073,#40074,#40075,#40076,#40077,#40078,#40079,#40080,#40081,
#40082,#40083,#40084,#40085,#40086,#40087,#40088,#40089,#40090,#40091,#40092,
#40093,#40094,#40095,#40096,#40097,#40098,#40099),.UNSPECIFIED.,.F.,.F.)
B_SPLINE_CURVE_WITH_KNOTS((6,1,1,1,1,1,1,1,1,1,1,1,1,1,1,1,1,1,1,1,1,1,
1,1,1,1,1,1,1,1,1,1,1,1,1,1,1,1,1,1,1,1,1,1,1,1,1,1,1,1,1,1,1,1,1,1,1,1,
1,1,1,1,1,1,1,6),(0.,0.0153846153846154,0.0307692307692308,0.0461538461538462,
0.0615384615384615,0.0769230769230769,0.0923076923076923,0.107692307692308,
0.123076923076923,0.138461538461538,0.153846153846154,0.169230769230769,
0.184615384615385,0.2,0.215384615384615,0.230769230769231,0.246153846153846,
0.261538461538462,0.276923076923077,0.292307692307692,0.307692307692308,
0.323076923076923,0.338461538461538,0.353846153846154,0.369230769230769,
0.384615384615385,0.4,0.415384615384615,0.430769230769231,0.446153846153846,
0.461538461538462,0.476923076923077,0.492307692307692,0.507692307692308,
0.523076923076923,0.538461538461538,0.553846153846154,0.569230769230769,
0.584615384615384,0.6,0.615384615384615,0.63076923076923,0.646153846153846,
0.661538461538461,0.676923076923076,0.692307692307692,0.707692307692307,
0.723076923076922,0.738461538461538,0.753846153846153,0.769230769230768,
0.784615384615384,0.799999999999999,0.815384615384614,0.83076923076923,
0.846153846153845,0.86153846153846,0.876923076923076,0.892307692307691,
0.907692307692306,0.923076923076922,0.938461538461537,0.953846153846152,
0.969230769230768,0.984615384615383,1.),.UNSPECIFIED.)
CURVE()
GEOMETRIC_REPRESENTATION_ITEM()
RATIONAL_B_SPLINE_CURVE((1.,1.,1.,1.,1.,1.,1.,1.,1.,1.,1.,1.,1.,1.,1.,1.,
1.,1.,1.,1.,1.,1.,1.,1.,1.,1.,1.,1.,1.,1.,1.,1.,1.,1.,1.,1.,1.,1.,1.,1.,
1.,1.,1.,1.,1.,1.,1.,1.,1.,1.,1.,1.,1.,1.,1.,1.,1.,1.,1.,1.,1.,1.,1.,1.,
1.,1.,1.,1.,1.,1.))
REPRESENTATION_ITEM('')
);
#284=(
BOUNDED_CURVE()
B_SPLINE_CURVE(5,(#40103,#40104,#40105,#40106,#40107,#40108,#40109,#40110,
#40111,#40112,#40113,#40114,#40115,#40116,#40117,#40118,#40119,#40120,#40121,
#40122,#40123,#40124,#40125,#40126,#40127,#40128,#40129,#40130,#40131,#40132,
#40133,#40134,#40135,#40136,#40137,#40138,#40139,#40140,#40141,#40142,#40143,
#40144,#40145,#40146,#40147,#40148,#40149,#40150,#40151,#40152,#40153,#40154,
#40155,#40156,#40157,#40158,#40159,#40160,#40161,#40162,#40163,#40164,#40165,
#40166,#40167,#40168,#40169,#40170,#40171,#40172),.UNSPECIFIED.,.F.,.F.)
B_SPLINE_CURVE_WITH_KNOTS((6,1,1,1,1,1,1,1,1,1,1,1,1,1,1,1,1,1,1,1,1,1,
1,1,1,1,1,1,1,1,1,1,1,1,1,1,1,1,1,1,1,1,1,1,1,1,1,1,1,1,1,1,1,1,1,1,1,1,
1,1,1,1,1,1,1,6),(0.,0.0153846153846154,0.0307692307692308,0.0461538461538462,
0.0615384615384615,0.0769230769230769,0.0923076923076923,0.107692307692308,
0.123076923076923,0.138461538461538,0.153846153846154,0.169230769230769,
0.184615384615385,0.2,0.215384615384615,0.230769230769231,0.246153846153846,
0.261538461538462,0.276923076923077,0.292307692307692,0.307692307692308,
0.323076923076923,0.338461538461538,0.353846153846154,0.369230769230769,
0.384615384615385,0.4,0.415384615384615,0.430769230769231,0.446153846153846,
0.461538461538462,0.476923076923077,0.492307692307692,0.507692307692308,
0.523076923076923,0.538461538461538,0.553846153846154,0.569230769230769,
0.584615384615384,0.6,0.615384615384615,0.63076923076923,0.646153846153846,
0.661538461538461,0.676923076923076,0.692307692307692,0.707692307692307,
0.723076923076922,0.738461538461538,0.753846153846153,0.769230769230768,
0.784615384615384,0.799999999999999,0.815384615384614,0.83076923076923,
0.846153846153845,0.86153846153846,0.876923076923076,0.892307692307691,
0.907692307692306,0.923076923076922,0.938461538461537,0.953846153846152,
0.969230769230768,0.984615384615383,1.),.UNSPECIFIED.)
CURVE()
GEOMETRIC_REPRESENTATION_ITEM()
RATIONAL_B_SPLINE_CURVE((1.,1.,1.,1.,1.,1.,1.,1.,1.,1.,1.,1.,1.,1.,1.,1.,
1.,1.,1.,1.,1.,1.,1.,1.,1.,1.,1.,1.,1.,1.,1.,1.,1.,1.,1.,1.,1.,1.,1.,1.,
1.,1.,1.,1.,1.,1.,1.,1.,1.,1.,1.,1.,1.,1.,1.,1.,1.,1.,1.,1.,1.,1.,1.,1.,
1.,1.,1.,1.,1.,1.))
REPRESENTATION_ITEM('')
);
#285=(
BOUNDED_CURVE()
B_SPLINE_CURVE(5,(#40176,#40177,#40178,#40179,#40180,#40181,#40182,#40183,
#40184,#40185,#40186,#40187,#40188,#40189,#40190,#40191,#40192,#40193,#40194,
#40195,#40196,#40197,#40198,#40199,#40200,#40201,#40202,#40203,#40204,#40205,
#40206,#40207,#40208,#40209,#40210,#40211,#40212,#40213,#40214,#40215,#40216,
#40217,#40218,#40219,#40220,#40221,#40222,#40223,#40224,#40225,#40226,#40227,
#40228,#40229,#40230,#40231,#40232,#40233,#40234,#40235,#40236,#40237,#40238,
#40239,#40240,#40241,#40242,#40243,#40244,#40245),.UNSPECIFIED.,.F.,.F.)
B_SPLINE_CURVE_WITH_KNOTS((6,1,1,1,1,1,1,1,1,1,1,1,1,1,1,1,1,1,1,1,1,1,
1,1,1,1,1,1,1,1,1,1,1,1,1,1,1,1,1,1,1,1,1,1,1,1,1,1,1,1,1,1,1,1,1,1,1,1,
1,1,1,1,1,1,1,6),(0.,0.0153846153846154,0.0307692307692308,0.0461538461538462,
0.0615384615384615,0.0769230769230769,0.0923076923076923,0.107692307692308,
0.123076923076923,0.138461538461538,0.153846153846154,0.169230769230769,
0.184615384615385,0.2,0.215384615384615,0.230769230769231,0.246153846153846,
0.261538461538462,0.276923076923077,0.292307692307692,0.307692307692308,
0.323076923076923,0.338461538461538,0.353846153846154,0.369230769230769,
0.384615384615385,0.4,0.415384615384615,0.430769230769231,0.446153846153846,
0.461538461538462,0.476923076923077,0.492307692307692,0.507692307692308,
0.523076923076923,0.538461538461538,0.553846153846154,0.569230769230769,
0.584615384615384,0.6,0.615384615384615,0.63076923076923,0.646153846153846,
0.661538461538461,0.676923076923076,0.692307692307692,0.707692307692307,
0.723076923076922,0.738461538461538,0.753846153846153,0.769230769230768,
0.784615384615384,0.799999999999999,0.815384615384614,0.83076923076923,
0.846153846153845,0.86153846153846,0.876923076923076,0.892307692307691,
0.907692307692306,0.923076923076922,0.938461538461537,0.953846153846152,
0.969230769230768,0.984615384615383,1.),.UNSPECIFIED.)
CURVE()
GEOMETRIC_REPRESENTATION_ITEM()
RATIONAL_B_SPLINE_CURVE((1.,1.,1.,1.,1.,1.,1.,1.,1.,1.,1.,1.,1.,1.,1.,1.,
1.,1.,1.,1.,1.,1.,1.,1.,1.,1.,1.,1.,1.,1.,1.,1.,1.,1.,1.,1.,1.,1.,1.,1.,
1.,1.,1.,1.,1.,1.,1.,1.,1.,1.,1.,1.,1.,1.,1.,1.,1.,1.,1.,1.,1.,1.,1.,1.,
1.,1.,1.,1.,1.,1.))
REPRESENTATION_ITEM('')
);
#286=(
BOUNDED_CURVE()
B_SPLINE_CURVE(5,(#40249,#40250,#40251,#40252,#40253,#40254,#40255,#40256,
#40257,#40258,#40259,#40260,#40261,#40262,#40263,#40264,#40265,#40266,#40267,
#40268,#40269,#40270,#40271,#40272,#40273,#40274,#40275,#40276,#40277,#40278,
#40279,#40280,#40281,#40282,#40283,#40284,#40285,#40286,#40287,#40288,#40289,
#40290,#40291,#40292,#40293,#40294,#40295,#40296,#40297,#40298,#40299,#40300,
#40301,#40302,#40303,#40304,#40305,#40306,#40307,#40308,#40309,#40310,#40311,
#40312,#40313,#40314,#40315,#40316,#40317,#40318),.UNSPECIFIED.,.F.,.F.)
B_SPLINE_CURVE_WITH_KNOTS((6,1,1,1,1,1,1,1,1,1,1,1,1,1,1,1,1,1,1,1,1,1,
1,1,1,1,1,1,1,1,1,1,1,1,1,1,1,1,1,1,1,1,1,1,1,1,1,1,1,1,1,1,1,1,1,1,1,1,
1,1,1,1,1,1,1,6),(0.,0.0153846153846154,0.0307692307692308,0.0461538461538462,
0.0615384615384615,0.0769230769230769,0.0923076923076923,0.107692307692308,
0.123076923076923,0.138461538461538,0.153846153846154,0.169230769230769,
0.184615384615385,0.2,0.215384615384615,0.230769230769231,0.246153846153846,
0.261538461538462,0.276923076923077,0.292307692307692,0.307692307692308,
0.323076923076923,0.338461538461538,0.353846153846154,0.369230769230769,
0.384615384615385,0.4,0.415384615384615,0.430769230769231,0.446153846153846,
0.461538461538462,0.476923076923077,0.492307692307692,0.507692307692308,
0.523076923076923,0.538461538461538,0.553846153846154,0.569230769230769,
0.584615384615384,0.6,0.615384615384615,0.63076923076923,0.646153846153846,
0.661538461538461,0.676923076923076,0.692307692307692,0.707692307692307,
0.723076923076922,0.738461538461538,0.753846153846153,0.769230769230768,
0.784615384615384,0.799999999999999,0.815384615384614,0.83076923076923,
0.846153846153845,0.86153846153846,0.876923076923076,0.892307692307691,
0.907692307692306,0.923076923076922,0.938461538461537,0.953846153846152,
0.969230769230768,0.984615384615383,1.),.UNSPECIFIED.)
CURVE()
GEOMETRIC_REPRESENTATION_ITEM()
RATIONAL_B_SPLINE_CURVE((1.,1.,1.,1.,1.,1.,1.,1.,1.,1.,1.,1.,1.,1.,1.,1.,
1.,1.,1.,1.,1.,1.,1.,1.,1.,1.,1.,1.,1.,1.,1.,1.,1.,1.,1.,1.,1.,1.,1.,1.,
1.,1.,1.,1.,1.,1.,1.,1.,1.,1.,1.,1.,1.,1.,1.,1.,1.,1.,1.,1.,1.,1.,1.,1.,
1.,1.,1.,1.,1.,1.))
REPRESENTATION_ITEM('')
);
#287=(
BOUNDED_CURVE()
B_SPLINE_CURVE(5,(#40322,#40323,#40324,#40325,#40326,#40327,#40328,#40329,
#40330,#40331,#40332,#40333,#40334,#40335,#40336,#40337,#40338,#40339,#40340,
#40341,#40342,#40343,#40344,#40345,#40346,#40347,#40348,#40349,#40350,#40351,
#40352,#40353,#40354,#40355,#40356,#40357,#40358,#40359,#40360,#40361,#40362,
#40363,#40364,#40365,#40366,#40367,#40368,#40369,#40370,#40371,#40372,#40373,
#40374,#40375,#40376,#40377,#40378,#40379,#40380,#40381,#40382,#40383,#40384,
#40385,#40386,#40387,#40388,#40389,#40390,#40391),.UNSPECIFIED.,.F.,.F.)
B_SPLINE_CURVE_WITH_KNOTS((6,1,1,1,1,1,1,1,1,1,1,1,1,1,1,1,1,1,1,1,1,1,
1,1,1,1,1,1,1,1,1,1,1,1,1,1,1,1,1,1,1,1,1,1,1,1,1,1,1,1,1,1,1,1,1,1,1,1,
1,1,1,1,1,1,1,6),(0.,0.0153846153846154,0.0307692307692308,0.0461538461538462,
0.0615384615384615,0.0769230769230769,0.0923076923076923,0.107692307692308,
0.123076923076923,0.138461538461538,0.153846153846154,0.169230769230769,
0.184615384615385,0.2,0.215384615384615,0.230769230769231,0.246153846153846,
0.261538461538462,0.276923076923077,0.292307692307692,0.307692307692308,
0.323076923076923,0.338461538461538,0.353846153846154,0.369230769230769,
0.384615384615385,0.4,0.415384615384615,0.430769230769231,0.446153846153846,
0.461538461538462,0.476923076923077,0.492307692307692,0.507692307692308,
0.523076923076923,0.538461538461538,0.553846153846154,0.569230769230769,
0.584615384615384,0.6,0.615384615384615,0.63076923076923,0.646153846153846,
0.661538461538461,0.676923076923076,0.692307692307692,0.707692307692307,
0.723076923076922,0.738461538461538,0.753846153846153,0.769230769230768,
0.784615384615384,0.799999999999999,0.815384615384614,0.83076923076923,
0.846153846153845,0.86153846153846,0.876923076923076,0.892307692307691,
0.907692307692306,0.923076923076922,0.938461538461537,0.953846153846152,
0.969230769230768,0.984615384615383,1.),.UNSPECIFIED.)
CURVE()
GEOMETRIC_REPRESENTATION_ITEM()
RATIONAL_B_SPLINE_CURVE((1.,1.,1.,1.,1.,1.,1.,1.,1.,1.,1.,1.,1.,1.,1.,1.,
1.,1.,1.,1.,1.,1.,1.,1.,1.,1.,1.,1.,1.,1.,1.,1.,1.,1.,1.,1.,1.,1.,1.,1.,
1.,1.,1.,1.,1.,1.,1.,1.,1.,1.,1.,1.,1.,1.,1.,1.,1.,1.,1.,1.,1.,1.,1.,1.,
1.,1.,1.,1.,1.,1.))
REPRESENTATION_ITEM('')
);
#288=(
BOUNDED_CURVE()
B_SPLINE_CURVE(5,(#40395,#40396,#40397,#40398,#40399,#40400,#40401,#40402,
#40403,#40404,#40405,#40406,#40407,#40408,#40409,#40410,#40411,#40412,#40413,
#40414,#40415,#40416,#40417,#40418,#40419,#40420,#40421,#40422,#40423,#40424,
#40425,#40426,#40427,#40428,#40429,#40430,#40431,#40432,#40433,#40434,#40435,
#40436,#40437,#40438,#40439,#40440,#40441,#40442,#40443,#40444,#40445,#40446,
#40447,#40448,#40449,#40450,#40451,#40452,#40453,#40454,#40455,#40456,#40457,
#40458,#40459,#40460,#40461,#40462,#40463,#40464),.UNSPECIFIED.,.F.,.F.)
B_SPLINE_CURVE_WITH_KNOTS((6,1,1,1,1,1,1,1,1,1,1,1,1,1,1,1,1,1,1,1,1,1,
1,1,1,1,1,1,1,1,1,1,1,1,1,1,1,1,1,1,1,1,1,1,1,1,1,1,1,1,1,1,1,1,1,1,1,1,
1,1,1,1,1,1,1,6),(0.,0.0153846153846154,0.0307692307692308,0.0461538461538462,
0.0615384615384615,0.0769230769230769,0.0923076923076923,0.107692307692308,
0.123076923076923,0.138461538461538,0.153846153846154,0.169230769230769,
0.184615384615385,0.2,0.215384615384615,0.230769230769231,0.246153846153846,
0.261538461538462,0.276923076923077,0.292307692307692,0.307692307692308,
0.323076923076923,0.338461538461538,0.353846153846154,0.369230769230769,
0.384615384615385,0.4,0.415384615384615,0.430769230769231,0.446153846153846,
0.461538461538462,0.476923076923077,0.492307692307692,0.507692307692308,
0.523076923076923,0.538461538461538,0.553846153846154,0.569230769230769,
0.584615384615384,0.6,0.615384615384615,0.63076923076923,0.646153846153846,
0.661538461538461,0.676923076923076,0.692307692307692,0.707692307692307,
0.723076923076922,0.738461538461538,0.753846153846153,0.769230769230768,
0.784615384615384,0.799999999999999,0.815384615384614,0.83076923076923,
0.846153846153845,0.86153846153846,0.876923076923076,0.892307692307691,
0.907692307692306,0.923076923076922,0.938461538461537,0.953846153846152,
0.969230769230768,0.984615384615383,1.),.UNSPECIFIED.)
CURVE()
GEOMETRIC_REPRESENTATION_ITEM()
RATIONAL_B_SPLINE_CURVE((1.,1.,1.,1.,1.,1.,1.,1.,1.,1.,1.,1.,1.,1.,1.,1.,
1.,1.,1.,1.,1.,1.,1.,1.,1.,1.,1.,1.,1.,1.,1.,1.,1.,1.,1.,1.,1.,1.,1.,1.,
1.,1.,1.,1.,1.,1.,1.,1.,1.,1.,1.,1.,1.,1.,1.,1.,1.,1.,1.,1.,1.,1.,1.,1.,
1.,1.,1.,1.,1.,1.))
REPRESENTATION_ITEM('')
);
#289=(
BOUNDED_CURVE()
B_SPLINE_CURVE(5,(#40468,#40469,#40470,#40471,#40472,#40473,#40474,#40475,
#40476,#40477,#40478,#40479,#40480,#40481,#40482,#40483,#40484,#40485,#40486,
#40487,#40488,#40489,#40490,#40491,#40492,#40493,#40494,#40495,#40496,#40497,
#40498,#40499,#40500,#40501,#40502,#40503,#40504,#40505,#40506,#40507,#40508,
#40509,#40510,#40511,#40512,#40513,#40514,#40515,#40516,#40517,#40518,#40519,
#40520,#40521,#40522,#40523,#40524,#40525,#40526,#40527,#40528,#40529,#40530,
#40531,#40532,#40533,#40534,#40535,#40536,#40537),.UNSPECIFIED.,.F.,.F.)
B_SPLINE_CURVE_WITH_KNOTS((6,1,1,1,1,1,1,1,1,1,1,1,1,1,1,1,1,1,1,1,1,1,
1,1,1,1,1,1,1,1,1,1,1,1,1,1,1,1,1,1,1,1,1,1,1,1,1,1,1,1,1,1,1,1,1,1,1,1,
1,1,1,1,1,1,1,6),(0.,0.0153846153846154,0.0307692307692308,0.0461538461538462,
0.0615384615384615,0.0769230769230769,0.0923076923076923,0.107692307692308,
0.123076923076923,0.138461538461538,0.153846153846154,0.169230769230769,
0.184615384615385,0.2,0.215384615384615,0.230769230769231,0.246153846153846,
0.261538461538462,0.276923076923077,0.292307692307692,0.307692307692308,
0.323076923076923,0.338461538461538,0.353846153846154,0.369230769230769,
0.384615384615385,0.4,0.415384615384615,0.430769230769231,0.446153846153846,
0.461538461538462,0.476923076923077,0.492307692307692,0.507692307692308,
0.523076923076923,0.538461538461538,0.553846153846154,0.569230769230769,
0.584615384615384,0.6,0.615384615384615,0.63076923076923,0.646153846153846,
0.661538461538461,0.676923076923076,0.692307692307692,0.707692307692307,
0.723076923076922,0.738461538461538,0.753846153846153,0.769230769230768,
0.784615384615384,0.799999999999999,0.815384615384614,0.83076923076923,
0.846153846153845,0.86153846153846,0.876923076923076,0.892307692307691,
0.907692307692306,0.923076923076922,0.938461538461537,0.953846153846152,
0.969230769230768,0.984615384615383,1.),.UNSPECIFIED.)
CURVE()
GEOMETRIC_REPRESENTATION_ITEM()
RATIONAL_B_SPLINE_CURVE((1.,1.,1.,1.,1.,1.,1.,1.,1.,1.,1.,1.,1.,1.,1.,1.,
1.,1.,1.,1.,1.,1.,1.,1.,1.,1.,1.,1.,1.,1.,1.,1.,1.,1.,1.,1.,1.,1.,1.,1.,
1.,1.,1.,1.,1.,1.,1.,1.,1.,1.,1.,1.,1.,1.,1.,1.,1.,1.,1.,1.,1.,1.,1.,1.,
1.,1.,1.,1.,1.,1.))
REPRESENTATION_ITEM('')
);
#290=(
BOUNDED_CURVE()
B_SPLINE_CURVE(5,(#40540,#40541,#40542,#40543,#40544,#40545,#40546,#40547,
#40548,#40549,#40550,#40551,#40552,#40553,#40554,#40555,#40556,#40557,#40558,
#40559,#40560,#40561,#40562,#40563,#40564,#40565,#40566,#40567,#40568,#40569,
#40570,#40571,#40572,#40573,#40574,#40575,#40576,#40577,#40578,#40579,#40580,
#40581,#40582,#40583,#40584,#40585,#40586,#40587,#40588,#40589,#40590,#40591,
#40592,#40593,#40594,#40595,#40596,#40597,#40598,#40599,#40600,#40601,#40602,
#40603,#40604,#40605,#40606,#40607,#40608,#40609),.UNSPECIFIED.,.F.,.F.)
B_SPLINE_CURVE_WITH_KNOTS((6,1,1,1,1,1,1,1,1,1,1,1,1,1,1,1,1,1,1,1,1,1,
1,1,1,1,1,1,1,1,1,1,1,1,1,1,1,1,1,1,1,1,1,1,1,1,1,1,1,1,1,1,1,1,1,1,1,1,
1,1,1,1,1,1,1,6),(0.,0.0153846153846154,0.0307692307692308,0.0461538461538462,
0.0615384615384615,0.0769230769230769,0.0923076923076923,0.107692307692308,
0.123076923076923,0.138461538461538,0.153846153846154,0.169230769230769,
0.184615384615385,0.2,0.215384615384615,0.230769230769231,0.246153846153846,
0.261538461538462,0.276923076923077,0.292307692307692,0.307692307692308,
0.323076923076923,0.338461538461538,0.353846153846154,0.369230769230769,
0.384615384615385,0.4,0.415384615384615,0.430769230769231,0.446153846153846,
0.461538461538462,0.476923076923077,0.492307692307692,0.507692307692308,
0.523076923076923,0.538461538461538,0.553846153846154,0.569230769230769,
0.584615384615384,0.6,0.615384615384615,0.63076923076923,0.646153846153846,
0.661538461538461,0.676923076923076,0.692307692307692,0.707692307692307,
0.723076923076922,0.738461538461538,0.753846153846153,0.769230769230768,
0.784615384615384,0.799999999999999,0.815384615384614,0.83076923076923,
0.846153846153845,0.86153846153846,0.876923076923076,0.892307692307691,
0.907692307692306,0.923076923076922,0.938461538461537,0.953846153846152,
0.969230769230768,0.984615384615383,1.),.UNSPECIFIED.)
CURVE()
GEOMETRIC_REPRESENTATION_ITEM()
RATIONAL_B_SPLINE_CURVE((1.,1.,1.,1.,1.,1.,1.,1.,1.,1.,1.,1.,1.,1.,1.,1.,
1.,1.,1.,1.,1.,1.,1.,1.,1.,1.,1.,1.,1.,1.,1.,1.,1.,1.,1.,1.,1.,1.,1.,1.,
1.,1.,1.,1.,1.,1.,1.,1.,1.,1.,1.,1.,1.,1.,1.,1.,1.,1.,1.,1.,1.,1.,1.,1.,
1.,1.,1.,1.,1.,1.))
REPRESENTATION_ITEM('')
);
#291=(
BOUNDED_CURVE()
B_SPLINE_CURVE(5,(#40757,#40758,#40759,#40760,#40761,#40762,#40763,#40764,
#40765,#40766,#40767,#40768,#40769,#40770,#40771,#40772,#40773,#40774,#40775,
#40776,#40777,#40778,#40779,#40780,#40781,#40782,#40783,#40784,#40785,#40786,
#40787,#40788,#40789,#40790,#40791,#40792,#40793,#40794,#40795,#40796,#40797,
#40798,#40799,#40800,#40801,#40802,#40803,#40804,#40805,#40806,#40807,#40808,
#40809,#40810,#40811,#40812,#40813,#40814,#40815,#40816,#40817,#40818,#40819,
#40820,#40821,#40822,#40823,#40824,#40825,#40826),.UNSPECIFIED.,.F.,.F.)
B_SPLINE_CURVE_WITH_KNOTS((6,1,1,1,1,1,1,1,1,1,1,1,1,1,1,1,1,1,1,1,1,1,
1,1,1,1,1,1,1,1,1,1,1,1,1,1,1,1,1,1,1,1,1,1,1,1,1,1,1,1,1,1,1,1,1,1,1,1,
1,1,1,1,1,1,1,6),(-1.,-0.984615384615383,-0.969230769230768,-0.953846153846152,
-0.938461538461537,-0.923076923076922,-0.907692307692306,-0.892307692307691,
-0.876923076923076,-0.86153846153846,-0.846153846153845,-0.83076923076923,
-0.815384615384614,-0.799999999999999,-0.784615384615384,-0.769230769230768,
-0.753846153846153,-0.738461538461538,-0.723076923076922,-0.707692307692307,
-0.692307692307692,-0.676923076923076,-0.661538461538461,-0.646153846153846,
-0.63076923076923,-0.615384615384615,-0.6,-0.584615384615384,-0.569230769230769,
-0.553846153846154,-0.538461538461538,-0.523076923076923,-0.507692307692308,
-0.492307692307692,-0.476923076923077,-0.461538461538462,-0.446153846153846,
-0.430769230769231,-0.415384615384615,-0.4,-0.384615384615385,-0.369230769230769,
-0.353846153846154,-0.338461538461538,-0.323076923076923,-0.307692307692308,
-0.292307692307692,-0.276923076923077,-0.261538461538462,-0.246153846153846,
-0.230769230769231,-0.215384615384615,-0.2,-0.184615384615385,-0.169230769230769,
-0.153846153846154,-0.138461538461538,-0.123076923076923,-0.107692307692308,
-0.0923076923076923,-0.0769230769230769,-0.0615384615384615,-0.0461538461538462,
-0.0307692307692308,-0.0153846153846154,0.),.UNSPECIFIED.)
CURVE()
GEOMETRIC_REPRESENTATION_ITEM()
RATIONAL_B_SPLINE_CURVE((1.,1.,1.,1.,1.,1.,1.,1.,1.,1.,1.,1.,1.,1.,1.,1.,
1.,1.,1.,1.,1.,1.,1.,1.,1.,1.,1.,1.,1.,1.,1.,1.,1.,1.,1.,1.,1.,1.,1.,1.,
1.,1.,1.,1.,1.,1.,1.,1.,1.,1.,1.,1.,1.,1.,1.,1.,1.,1.,1.,1.,1.,1.,1.,1.,
1.,1.,1.,1.,1.,1.))
REPRESENTATION_ITEM('')
);
#292=(
BOUNDED_CURVE()
B_SPLINE_CURVE(5,(#40973,#40974,#40975,#40976,#40977,#40978,#40979,#40980,
#40981,#40982,#40983,#40984,#40985,#40986,#40987,#40988,#40989,#40990,#40991,
#40992,#40993,#40994,#40995,#40996,#40997,#40998,#40999,#41000,#41001,#41002,
#41003,#41004,#41005,#41006,#41007,#41008,#41009,#41010,#41011,#41012,#41013,
#41014,#41015,#41016,#41017,#41018,#41019,#41020,#41021,#41022,#41023,#41024,
#41025,#41026,#41027,#41028,#41029,#41030,#41031,#41032,#41033,#41034,#41035,
#41036,#41037,#41038,#41039,#41040,#41041,#41042),.UNSPECIFIED.,.F.,.F.)
B_SPLINE_CURVE_WITH_KNOTS((6,1,1,1,1,1,1,1,1,1,1,1,1,1,1,1,1,1,1,1,1,1,
1,1,1,1,1,1,1,1,1,1,1,1,1,1,1,1,1,1,1,1,1,1,1,1,1,1,1,1,1,1,1,1,1,1,1,1,
1,1,1,1,1,1,1,6),(-1.,-0.984615384615383,-0.969230769230768,-0.953846153846152,
-0.938461538461537,-0.923076923076922,-0.907692307692306,-0.892307692307691,
-0.876923076923076,-0.86153846153846,-0.846153846153845,-0.83076923076923,
-0.815384615384614,-0.799999999999999,-0.784615384615384,-0.769230769230768,
-0.753846153846153,-0.738461538461538,-0.723076923076922,-0.707692307692307,
-0.692307692307692,-0.676923076923076,-0.661538461538461,-0.646153846153846,
-0.63076923076923,-0.615384615384615,-0.6,-0.584615384615384,-0.569230769230769,
-0.553846153846154,-0.538461538461538,-0.523076923076923,-0.507692307692308,
-0.492307692307692,-0.476923076923077,-0.461538461538462,-0.446153846153846,
-0.430769230769231,-0.415384615384615,-0.4,-0.384615384615385,-0.369230769230769,
-0.353846153846154,-0.338461538461538,-0.323076923076923,-0.307692307692308,
-0.292307692307692,-0.276923076923077,-0.261538461538462,-0.246153846153846,
-0.230769230769231,-0.215384615384615,-0.2,-0.184615384615385,-0.169230769230769,
-0.153846153846154,-0.138461538461538,-0.123076923076923,-0.107692307692308,
-0.0923076923076923,-0.0769230769230769,-0.0615384615384615,-0.0461538461538462,
-0.0307692307692308,-0.0153846153846154,0.),.UNSPECIFIED.)
CURVE()
GEOMETRIC_REPRESENTATION_ITEM()
RATIONAL_B_SPLINE_CURVE((1.,1.,1.,1.,1.,1.,1.,1.,1.,1.,1.,1.,1.,1.,1.,1.,
1.,1.,1.,1.,1.,1.,1.,1.,1.,1.,1.,1.,1.,1.,1.,1.,1.,1.,1.,1.,1.,1.,1.,1.,
1.,1.,1.,1.,1.,1.,1.,1.,1.,1.,1.,1.,1.,1.,1.,1.,1.,1.,1.,1.,1.,1.,1.,1.,
1.,1.,1.,1.,1.,1.))
REPRESENTATION_ITEM('')
);
#293=(
BOUNDED_CURVE()
B_SPLINE_CURVE(5,(#41189,#41190,#41191,#41192,#41193,#41194,#41195,#41196,
#41197,#41198,#41199,#41200,#41201,#41202,#41203,#41204,#41205,#41206,#41207,
#41208,#41209,#41210,#41211,#41212,#41213,#41214,#41215,#41216,#41217,#41218,
#41219,#41220,#41221,#41222,#41223,#41224,#41225,#41226,#41227,#41228,#41229,
#41230,#41231,#41232,#41233,#41234,#41235,#41236,#41237,#41238,#41239,#41240,
#41241,#41242,#41243,#41244,#41245,#41246,#41247,#41248,#41249,#41250,#41251,
#41252,#41253,#41254,#41255,#41256,#41257,#41258),.UNSPECIFIED.,.F.,.F.)
B_SPLINE_CURVE_WITH_KNOTS((6,1,1,1,1,1,1,1,1,1,1,1,1,1,1,1,1,1,1,1,1,1,
1,1,1,1,1,1,1,1,1,1,1,1,1,1,1,1,1,1,1,1,1,1,1,1,1,1,1,1,1,1,1,1,1,1,1,1,
1,1,1,1,1,1,1,6),(-1.,-0.984615384615383,-0.969230769230768,-0.953846153846152,
-0.938461538461537,-0.923076923076922,-0.907692307692306,-0.892307692307691,
-0.876923076923076,-0.86153846153846,-0.846153846153845,-0.83076923076923,
-0.815384615384614,-0.799999999999999,-0.784615384615384,-0.769230769230768,
-0.753846153846153,-0.738461538461538,-0.723076923076922,-0.707692307692307,
-0.692307692307692,-0.676923076923076,-0.661538461538461,-0.646153846153846,
-0.63076923076923,-0.615384615384615,-0.6,-0.584615384615384,-0.569230769230769,
-0.553846153846154,-0.538461538461538,-0.523076923076923,-0.507692307692308,
-0.492307692307692,-0.476923076923077,-0.461538461538462,-0.446153846153846,
-0.430769230769231,-0.415384615384615,-0.4,-0.384615384615385,-0.369230769230769,
-0.353846153846154,-0.338461538461538,-0.323076923076923,-0.307692307692308,
-0.292307692307692,-0.276923076923077,-0.261538461538462,-0.246153846153846,
-0.230769230769231,-0.215384615384615,-0.2,-0.184615384615385,-0.169230769230769,
-0.153846153846154,-0.138461538461538,-0.123076923076923,-0.107692307692308,
-0.0923076923076923,-0.0769230769230769,-0.0615384615384615,-0.0461538461538462,
-0.0307692307692308,-0.0153846153846154,0.),.UNSPECIFIED.)
CURVE()
GEOMETRIC_REPRESENTATION_ITEM()
RATIONAL_B_SPLINE_CURVE((1.,1.,1.,1.,1.,1.,1.,1.,1.,1.,1.,1.,1.,1.,1.,1.,
1.,1.,1.,1.,1.,1.,1.,1.,1.,1.,1.,1.,1.,1.,1.,1.,1.,1.,1.,1.,1.,1.,1.,1.,
1.,1.,1.,1.,1.,1.,1.,1.,1.,1.,1.,1.,1.,1.,1.,1.,1.,1.,1.,1.,1.,1.,1.,1.,
1.,1.,1.,1.,1.,1.))
REPRESENTATION_ITEM('')
);
#294=(
BOUNDED_CURVE()
B_SPLINE_CURVE(5,(#41405,#41406,#41407,#41408,#41409,#41410,#41411,#41412,
#41413,#41414,#41415,#41416,#41417,#41418,#41419,#41420,#41421,#41422,#41423,
#41424,#41425,#41426,#41427,#41428,#41429,#41430,#41431,#41432,#41433,#41434,
#41435,#41436,#41437,#41438,#41439,#41440,#41441,#41442,#41443,#41444,#41445,
#41446,#41447,#41448,#41449,#41450,#41451,#41452,#41453,#41454,#41455,#41456,
#41457,#41458,#41459,#41460,#41461,#41462,#41463,#41464,#41465,#41466,#41467,
#41468,#41469,#41470,#41471,#41472,#41473,#41474),.UNSPECIFIED.,.F.,.F.)
B_SPLINE_CURVE_WITH_KNOTS((6,1,1,1,1,1,1,1,1,1,1,1,1,1,1,1,1,1,1,1,1,1,
1,1,1,1,1,1,1,1,1,1,1,1,1,1,1,1,1,1,1,1,1,1,1,1,1,1,1,1,1,1,1,1,1,1,1,1,
1,1,1,1,1,1,1,6),(-1.,-0.984615384615383,-0.969230769230768,-0.953846153846152,
-0.938461538461537,-0.923076923076922,-0.907692307692306,-0.892307692307691,
-0.876923076923076,-0.86153846153846,-0.846153846153845,-0.83076923076923,
-0.815384615384614,-0.799999999999999,-0.784615384615384,-0.769230769230768,
-0.753846153846153,-0.738461538461538,-0.723076923076922,-0.707692307692307,
-0.692307692307692,-0.676923076923076,-0.661538461538461,-0.646153846153846,
-0.63076923076923,-0.615384615384615,-0.6,-0.584615384615384,-0.569230769230769,
-0.553846153846154,-0.538461538461538,-0.523076923076923,-0.507692307692308,
-0.492307692307692,-0.476923076923077,-0.461538461538462,-0.446153846153846,
-0.430769230769231,-0.415384615384615,-0.4,-0.384615384615385,-0.369230769230769,
-0.353846153846154,-0.338461538461538,-0.323076923076923,-0.307692307692308,
-0.292307692307692,-0.276923076923077,-0.261538461538462,-0.246153846153846,
-0.230769230769231,-0.215384615384615,-0.2,-0.184615384615385,-0.169230769230769,
-0.153846153846154,-0.138461538461538,-0.123076923076923,-0.107692307692308,
-0.0923076923076923,-0.0769230769230769,-0.0615384615384615,-0.0461538461538462,
-0.0307692307692308,-0.0153846153846154,0.),.UNSPECIFIED.)
CURVE()
GEOMETRIC_REPRESENTATION_ITEM()
RATIONAL_B_SPLINE_CURVE((1.,1.,1.,1.,1.,1.,1.,1.,1.,1.,1.,1.,1.,1.,1.,1.,
1.,1.,1.,1.,1.,1.,1.,1.,1.,1.,1.,1.,1.,1.,1.,1.,1.,1.,1.,1.,1.,1.,1.,1.,
1.,1.,1.,1.,1.,1.,1.,1.,1.,1.,1.,1.,1.,1.,1.,1.,1.,1.,1.,1.,1.,1.,1.,1.,
1.,1.,1.,1.,1.,1.))
REPRESENTATION_ITEM('')
);
#295=(
BOUNDED_CURVE()
B_SPLINE_CURVE(5,(#41621,#41622,#41623,#41624,#41625,#41626,#41627,#41628,
#41629,#41630,#41631,#41632,#41633,#41634,#41635,#41636,#41637,#41638,#41639,
#41640,#41641,#41642,#41643,#41644,#41645,#41646,#41647,#41648,#41649,#41650,
#41651,#41652,#41653,#41654,#41655,#41656,#41657,#41658,#41659,#41660,#41661,
#41662,#41663,#41664,#41665,#41666,#41667,#41668,#41669,#41670,#41671,#41672,
#41673,#41674,#41675,#41676,#41677,#41678,#41679,#41680,#41681,#41682,#41683,
#41684,#41685,#41686,#41687,#41688,#41689,#41690),.UNSPECIFIED.,.F.,.F.)
B_SPLINE_CURVE_WITH_KNOTS((6,1,1,1,1,1,1,1,1,1,1,1,1,1,1,1,1,1,1,1,1,1,
1,1,1,1,1,1,1,1,1,1,1,1,1,1,1,1,1,1,1,1,1,1,1,1,1,1,1,1,1,1,1,1,1,1,1,1,
1,1,1,1,1,1,1,6),(-1.,-0.984615384615383,-0.969230769230768,-0.953846153846152,
-0.938461538461537,-0.923076923076922,-0.907692307692306,-0.892307692307691,
-0.876923076923076,-0.86153846153846,-0.846153846153845,-0.83076923076923,
-0.815384615384614,-0.799999999999999,-0.784615384615384,-0.769230769230768,
-0.753846153846153,-0.738461538461538,-0.723076923076922,-0.707692307692307,
-0.692307692307692,-0.676923076923076,-0.661538461538461,-0.646153846153846,
-0.63076923076923,-0.615384615384615,-0.6,-0.584615384615384,-0.569230769230769,
-0.553846153846154,-0.538461538461538,-0.523076923076923,-0.507692307692308,
-0.492307692307692,-0.476923076923077,-0.461538461538462,-0.446153846153846,
-0.430769230769231,-0.415384615384615,-0.4,-0.384615384615385,-0.369230769230769,
-0.353846153846154,-0.338461538461538,-0.323076923076923,-0.307692307692308,
-0.292307692307692,-0.276923076923077,-0.261538461538462,-0.246153846153846,
-0.230769230769231,-0.215384615384615,-0.2,-0.184615384615385,-0.169230769230769,
-0.153846153846154,-0.138461538461538,-0.123076923076923,-0.107692307692308,
-0.0923076923076923,-0.0769230769230769,-0.0615384615384615,-0.0461538461538462,
-0.0307692307692308,-0.0153846153846154,0.),.UNSPECIFIED.)
CURVE()
GEOMETRIC_REPRESENTATION_ITEM()
RATIONAL_B_SPLINE_CURVE((1.,1.,1.,1.,1.,1.,1.,1.,1.,1.,1.,1.,1.,1.,1.,1.,
1.,1.,1.,1.,1.,1.,1.,1.,1.,1.,1.,1.,1.,1.,1.,1.,1.,1.,1.,1.,1.,1.,1.,1.,
1.,1.,1.,1.,1.,1.,1.,1.,1.,1.,1.,1.,1.,1.,1.,1.,1.,1.,1.,1.,1.,1.,1.,1.,
1.,1.,1.,1.,1.,1.))
REPRESENTATION_ITEM('')
);
#296=(
BOUNDED_CURVE()
B_SPLINE_CURVE(5,(#41837,#41838,#41839,#41840,#41841,#41842,#41843,#41844,
#41845,#41846,#41847,#41848,#41849,#41850,#41851,#41852,#41853,#41854,#41855,
#41856,#41857,#41858,#41859,#41860,#41861,#41862,#41863,#41864,#41865,#41866,
#41867,#41868,#41869,#41870,#41871,#41872,#41873,#41874,#41875,#41876,#41877,
#41878,#41879,#41880,#41881,#41882,#41883,#41884,#41885,#41886,#41887,#41888,
#41889,#41890,#41891,#41892,#41893,#41894,#41895,#41896,#41897,#41898,#41899,
#41900,#41901,#41902,#41903,#41904,#41905,#41906),.UNSPECIFIED.,.F.,.F.)
B_SPLINE_CURVE_WITH_KNOTS((6,1,1,1,1,1,1,1,1,1,1,1,1,1,1,1,1,1,1,1,1,1,
1,1,1,1,1,1,1,1,1,1,1,1,1,1,1,1,1,1,1,1,1,1,1,1,1,1,1,1,1,1,1,1,1,1,1,1,
1,1,1,1,1,1,1,6),(-1.,-0.984615384615383,-0.969230769230768,-0.953846153846152,
-0.938461538461537,-0.923076923076922,-0.907692307692306,-0.892307692307691,
-0.876923076923076,-0.86153846153846,-0.846153846153845,-0.83076923076923,
-0.815384615384614,-0.799999999999999,-0.784615384615384,-0.769230769230768,
-0.753846153846153,-0.738461538461538,-0.723076923076922,-0.707692307692307,
-0.692307692307692,-0.676923076923076,-0.661538461538461,-0.646153846153846,
-0.63076923076923,-0.615384615384615,-0.6,-0.584615384615384,-0.569230769230769,
-0.553846153846154,-0.538461538461538,-0.523076923076923,-0.507692307692308,
-0.492307692307692,-0.476923076923077,-0.461538461538462,-0.446153846153846,
-0.430769230769231,-0.415384615384615,-0.4,-0.384615384615385,-0.369230769230769,
-0.353846153846154,-0.338461538461538,-0.323076923076923,-0.307692307692308,
-0.292307692307692,-0.276923076923077,-0.261538461538462,-0.246153846153846,
-0.230769230769231,-0.215384615384615,-0.2,-0.184615384615385,-0.169230769230769,
-0.153846153846154,-0.138461538461538,-0.123076923076923,-0.107692307692308,
-0.0923076923076923,-0.0769230769230769,-0.0615384615384615,-0.0461538461538462,
-0.0307692307692308,-0.0153846153846154,0.),.UNSPECIFIED.)
CURVE()
GEOMETRIC_REPRESENTATION_ITEM()
RATIONAL_B_SPLINE_CURVE((1.,1.,1.,1.,1.,1.,1.,1.,1.,1.,1.,1.,1.,1.,1.,1.,
1.,1.,1.,1.,1.,1.,1.,1.,1.,1.,1.,1.,1.,1.,1.,1.,1.,1.,1.,1.,1.,1.,1.,1.,
1.,1.,1.,1.,1.,1.,1.,1.,1.,1.,1.,1.,1.,1.,1.,1.,1.,1.,1.,1.,1.,1.,1.,1.,
1.,1.,1.,1.,1.,1.))
REPRESENTATION_ITEM('')
);
#297=(
BOUNDED_CURVE()
B_SPLINE_CURVE(5,(#42053,#42054,#42055,#42056,#42057,#42058,#42059,#42060,
#42061,#42062,#42063,#42064,#42065,#42066,#42067,#42068,#42069,#42070,#42071,
#42072,#42073,#42074,#42075,#42076,#42077,#42078,#42079,#42080,#42081,#42082,
#42083,#42084,#42085,#42086,#42087,#42088,#42089,#42090,#42091,#42092,#42093,
#42094,#42095,#42096,#42097,#42098,#42099,#42100,#42101,#42102,#42103,#42104,
#42105,#42106,#42107,#42108,#42109,#42110,#42111,#42112,#42113,#42114,#42115,
#42116,#42117,#42118,#42119,#42120,#42121,#42122),.UNSPECIFIED.,.F.,.F.)
B_SPLINE_CURVE_WITH_KNOTS((6,1,1,1,1,1,1,1,1,1,1,1,1,1,1,1,1,1,1,1,1,1,
1,1,1,1,1,1,1,1,1,1,1,1,1,1,1,1,1,1,1,1,1,1,1,1,1,1,1,1,1,1,1,1,1,1,1,1,
1,1,1,1,1,1,1,6),(-1.,-0.984615384615383,-0.969230769230768,-0.953846153846152,
-0.938461538461537,-0.923076923076922,-0.907692307692306,-0.892307692307691,
-0.876923076923076,-0.86153846153846,-0.846153846153845,-0.83076923076923,
-0.815384615384614,-0.799999999999999,-0.784615384615384,-0.769230769230768,
-0.753846153846153,-0.738461538461538,-0.723076923076922,-0.707692307692307,
-0.692307692307692,-0.676923076923076,-0.661538461538461,-0.646153846153846,
-0.63076923076923,-0.615384615384615,-0.6,-0.584615384615384,-0.569230769230769,
-0.553846153846154,-0.538461538461538,-0.523076923076923,-0.507692307692308,
-0.492307692307692,-0.476923076923077,-0.461538461538462,-0.446153846153846,
-0.430769230769231,-0.415384615384615,-0.4,-0.384615384615385,-0.369230769230769,
-0.353846153846154,-0.338461538461538,-0.323076923076923,-0.307692307692308,
-0.292307692307692,-0.276923076923077,-0.261538461538462,-0.246153846153846,
-0.230769230769231,-0.215384615384615,-0.2,-0.184615384615385,-0.169230769230769,
-0.153846153846154,-0.138461538461538,-0.123076923076923,-0.107692307692308,
-0.0923076923076923,-0.0769230769230769,-0.0615384615384615,-0.0461538461538462,
-0.0307692307692308,-0.0153846153846154,0.),.UNSPECIFIED.)
CURVE()
GEOMETRIC_REPRESENTATION_ITEM()
RATIONAL_B_SPLINE_CURVE((1.,1.,1.,1.,1.,1.,1.,1.,1.,1.,1.,1.,1.,1.,1.,1.,
1.,1.,1.,1.,1.,1.,1.,1.,1.,1.,1.,1.,1.,1.,1.,1.,1.,1.,1.,1.,1.,1.,1.,1.,
1.,1.,1.,1.,1.,1.,1.,1.,1.,1.,1.,1.,1.,1.,1.,1.,1.,1.,1.,1.,1.,1.,1.,1.,
1.,1.,1.,1.,1.,1.))
REPRESENTATION_ITEM('')
);
#298=(
BOUNDED_CURVE()
B_SPLINE_CURVE(5,(#42269,#42270,#42271,#42272,#42273,#42274,#42275,#42276,
#42277,#42278,#42279,#42280,#42281,#42282,#42283,#42284,#42285,#42286,#42287,
#42288,#42289,#42290,#42291,#42292,#42293,#42294,#42295,#42296,#42297,#42298,
#42299,#42300,#42301,#42302,#42303,#42304,#42305,#42306,#42307,#42308,#42309,
#42310,#42311,#42312,#42313,#42314,#42315,#42316,#42317,#42318,#42319,#42320,
#42321,#42322,#42323,#42324,#42325,#42326,#42327,#42328,#42329,#42330,#42331,
#42332,#42333,#42334,#42335,#42336,#42337,#42338),.UNSPECIFIED.,.F.,.F.)
B_SPLINE_CURVE_WITH_KNOTS((6,1,1,1,1,1,1,1,1,1,1,1,1,1,1,1,1,1,1,1,1,1,
1,1,1,1,1,1,1,1,1,1,1,1,1,1,1,1,1,1,1,1,1,1,1,1,1,1,1,1,1,1,1,1,1,1,1,1,
1,1,1,1,1,1,1,6),(-1.,-0.984615384615383,-0.969230769230768,-0.953846153846152,
-0.938461538461537,-0.923076923076922,-0.907692307692306,-0.892307692307691,
-0.876923076923076,-0.86153846153846,-0.846153846153845,-0.83076923076923,
-0.815384615384614,-0.799999999999999,-0.784615384615384,-0.769230769230768,
-0.753846153846153,-0.738461538461538,-0.723076923076922,-0.707692307692307,
-0.692307692307692,-0.676923076923076,-0.661538461538461,-0.646153846153846,
-0.63076923076923,-0.615384615384615,-0.6,-0.584615384615384,-0.569230769230769,
-0.553846153846154,-0.538461538461538,-0.523076923076923,-0.507692307692308,
-0.492307692307692,-0.476923076923077,-0.461538461538462,-0.446153846153846,
-0.430769230769231,-0.415384615384615,-0.4,-0.384615384615385,-0.369230769230769,
-0.353846153846154,-0.338461538461538,-0.323076923076923,-0.307692307692308,
-0.292307692307692,-0.276923076923077,-0.261538461538462,-0.246153846153846,
-0.230769230769231,-0.215384615384615,-0.2,-0.184615384615385,-0.169230769230769,
-0.153846153846154,-0.138461538461538,-0.123076923076923,-0.107692307692308,
-0.0923076923076923,-0.0769230769230769,-0.0615384615384615,-0.0461538461538462,
-0.0307692307692308,-0.0153846153846154,0.),.UNSPECIFIED.)
CURVE()
GEOMETRIC_REPRESENTATION_ITEM()
RATIONAL_B_SPLINE_CURVE((1.,1.,1.,1.,1.,1.,1.,1.,1.,1.,1.,1.,1.,1.,1.,1.,
1.,1.,1.,1.,1.,1.,1.,1.,1.,1.,1.,1.,1.,1.,1.,1.,1.,1.,1.,1.,1.,1.,1.,1.,
1.,1.,1.,1.,1.,1.,1.,1.,1.,1.,1.,1.,1.,1.,1.,1.,1.,1.,1.,1.,1.,1.,1.,1.,
1.,1.,1.,1.,1.,1.))
REPRESENTATION_ITEM('')
);
#299=(
BOUNDED_CURVE()
B_SPLINE_CURVE(5,(#42485,#42486,#42487,#42488,#42489,#42490,#42491,#42492,
#42493,#42494,#42495,#42496,#42497,#42498,#42499,#42500,#42501,#42502,#42503,
#42504,#42505,#42506,#42507,#42508,#42509,#42510,#42511,#42512,#42513,#42514,
#42515,#42516,#42517,#42518,#42519,#42520,#42521,#42522,#42523,#42524,#42525,
#42526,#42527,#42528,#42529,#42530,#42531,#42532,#42533,#42534,#42535,#42536,
#42537,#42538,#42539,#42540,#42541,#42542,#42543,#42544,#42545,#42546,#42547,
#42548,#42549,#42550,#42551,#42552,#42553,#42554),.UNSPECIFIED.,.F.,.F.)
B_SPLINE_CURVE_WITH_KNOTS((6,1,1,1,1,1,1,1,1,1,1,1,1,1,1,1,1,1,1,1,1,1,
1,1,1,1,1,1,1,1,1,1,1,1,1,1,1,1,1,1,1,1,1,1,1,1,1,1,1,1,1,1,1,1,1,1,1,1,
1,1,1,1,1,1,1,6),(-1.,-0.984615384615383,-0.969230769230768,-0.953846153846152,
-0.938461538461537,-0.923076923076922,-0.907692307692306,-0.892307692307691,
-0.876923076923076,-0.86153846153846,-0.846153846153845,-0.83076923076923,
-0.815384615384614,-0.799999999999999,-0.784615384615384,-0.769230769230768,
-0.753846153846153,-0.738461538461538,-0.723076923076922,-0.707692307692307,
-0.692307692307692,-0.676923076923076,-0.661538461538461,-0.646153846153846,
-0.63076923076923,-0.615384615384615,-0.6,-0.584615384615384,-0.569230769230769,
-0.553846153846154,-0.538461538461538,-0.523076923076923,-0.507692307692308,
-0.492307692307692,-0.476923076923077,-0.461538461538462,-0.446153846153846,
-0.430769230769231,-0.415384615384615,-0.4,-0.384615384615385,-0.369230769230769,
-0.353846153846154,-0.338461538461538,-0.323076923076923,-0.307692307692308,
-0.292307692307692,-0.276923076923077,-0.261538461538462,-0.246153846153846,
-0.230769230769231,-0.215384615384615,-0.2,-0.184615384615385,-0.169230769230769,
-0.153846153846154,-0.138461538461538,-0.123076923076923,-0.107692307692308,
-0.0923076923076923,-0.0769230769230769,-0.0615384615384615,-0.0461538461538462,
-0.0307692307692308,-0.0153846153846154,0.),.UNSPECIFIED.)
CURVE()
GEOMETRIC_REPRESENTATION_ITEM()
RATIONAL_B_SPLINE_CURVE((1.,1.,1.,1.,1.,1.,1.,1.,1.,1.,1.,1.,1.,1.,1.,1.,
1.,1.,1.,1.,1.,1.,1.,1.,1.,1.,1.,1.,1.,1.,1.,1.,1.,1.,1.,1.,1.,1.,1.,1.,
1.,1.,1.,1.,1.,1.,1.,1.,1.,1.,1.,1.,1.,1.,1.,1.,1.,1.,1.,1.,1.,1.,1.,1.,
1.,1.,1.,1.,1.,1.))
REPRESENTATION_ITEM('')
);
#300=(
BOUNDED_CURVE()
B_SPLINE_CURVE(5,(#42701,#42702,#42703,#42704,#42705,#42706,#42707,#42708,
#42709,#42710,#42711,#42712,#42713,#42714,#42715,#42716,#42717,#42718,#42719,
#42720,#42721,#42722,#42723,#42724,#42725,#42726,#42727,#42728,#42729,#42730,
#42731,#42732,#42733,#42734,#42735,#42736,#42737,#42738,#42739,#42740,#42741,
#42742,#42743,#42744,#42745,#42746,#42747,#42748,#42749,#42750,#42751,#42752,
#42753,#42754,#42755,#42756,#42757,#42758,#42759,#42760,#42761,#42762,#42763,
#42764,#42765,#42766,#42767,#42768,#42769,#42770),.UNSPECIFIED.,.F.,.F.)
B_SPLINE_CURVE_WITH_KNOTS((6,1,1,1,1,1,1,1,1,1,1,1,1,1,1,1,1,1,1,1,1,1,
1,1,1,1,1,1,1,1,1,1,1,1,1,1,1,1,1,1,1,1,1,1,1,1,1,1,1,1,1,1,1,1,1,1,1,1,
1,1,1,1,1,1,1,6),(-1.,-0.984615384615383,-0.969230769230768,-0.953846153846152,
-0.938461538461537,-0.923076923076922,-0.907692307692306,-0.892307692307691,
-0.876923076923076,-0.86153846153846,-0.846153846153845,-0.83076923076923,
-0.815384615384614,-0.799999999999999,-0.784615384615384,-0.769230769230768,
-0.753846153846153,-0.738461538461538,-0.723076923076922,-0.707692307692307,
-0.692307692307692,-0.676923076923076,-0.661538461538461,-0.646153846153846,
-0.63076923076923,-0.615384615384615,-0.6,-0.584615384615384,-0.569230769230769,
-0.553846153846154,-0.538461538461538,-0.523076923076923,-0.507692307692308,
-0.492307692307692,-0.476923076923077,-0.461538461538462,-0.446153846153846,
-0.430769230769231,-0.415384615384615,-0.4,-0.384615384615385,-0.369230769230769,
-0.353846153846154,-0.338461538461538,-0.323076923076923,-0.307692307692308,
-0.292307692307692,-0.276923076923077,-0.261538461538462,-0.246153846153846,
-0.230769230769231,-0.215384615384615,-0.2,-0.184615384615385,-0.169230769230769,
-0.153846153846154,-0.138461538461538,-0.123076923076923,-0.107692307692308,
-0.0923076923076923,-0.0769230769230769,-0.0615384615384615,-0.0461538461538462,
-0.0307692307692308,-0.0153846153846154,0.),.UNSPECIFIED.)
CURVE()
GEOMETRIC_REPRESENTATION_ITEM()
RATIONAL_B_SPLINE_CURVE((1.,1.,1.,1.,1.,1.,1.,1.,1.,1.,1.,1.,1.,1.,1.,1.,
1.,1.,1.,1.,1.,1.,1.,1.,1.,1.,1.,1.,1.,1.,1.,1.,1.,1.,1.,1.,1.,1.,1.,1.,
1.,1.,1.,1.,1.,1.,1.,1.,1.,1.,1.,1.,1.,1.,1.,1.,1.,1.,1.,1.,1.,1.,1.,1.,
1.,1.,1.,1.,1.,1.))
REPRESENTATION_ITEM('')
);
#301=(
BOUNDED_CURVE()
B_SPLINE_CURVE(5,(#42917,#42918,#42919,#42920,#42921,#42922,#42923,#42924,
#42925,#42926,#42927,#42928,#42929,#42930,#42931,#42932,#42933,#42934,#42935,
#42936,#42937,#42938,#42939,#42940,#42941,#42942,#42943,#42944,#42945,#42946,
#42947,#42948,#42949,#42950,#42951,#42952,#42953,#42954,#42955,#42956,#42957,
#42958,#42959,#42960,#42961,#42962,#42963,#42964,#42965,#42966,#42967,#42968,
#42969,#42970,#42971,#42972,#42973,#42974,#42975,#42976,#42977,#42978,#42979,
#42980,#42981,#42982,#42983,#42984,#42985,#42986),.UNSPECIFIED.,.F.,.F.)
B_SPLINE_CURVE_WITH_KNOTS((6,1,1,1,1,1,1,1,1,1,1,1,1,1,1,1,1,1,1,1,1,1,
1,1,1,1,1,1,1,1,1,1,1,1,1,1,1,1,1,1,1,1,1,1,1,1,1,1,1,1,1,1,1,1,1,1,1,1,
1,1,1,1,1,1,1,6),(-1.,-0.984615384615383,-0.969230769230768,-0.953846153846152,
-0.938461538461537,-0.923076923076922,-0.907692307692306,-0.892307692307691,
-0.876923076923076,-0.86153846153846,-0.846153846153845,-0.83076923076923,
-0.815384615384614,-0.799999999999999,-0.784615384615384,-0.769230769230768,
-0.753846153846153,-0.738461538461538,-0.723076923076922,-0.707692307692307,
-0.692307692307692,-0.676923076923076,-0.661538461538461,-0.646153846153846,
-0.63076923076923,-0.615384615384615,-0.6,-0.584615384615384,-0.569230769230769,
-0.553846153846154,-0.538461538461538,-0.523076923076923,-0.507692307692308,
-0.492307692307692,-0.476923076923077,-0.461538461538462,-0.446153846153846,
-0.430769230769231,-0.415384615384615,-0.4,-0.384615384615385,-0.369230769230769,
-0.353846153846154,-0.338461538461538,-0.323076923076923,-0.307692307692308,
-0.292307692307692,-0.276923076923077,-0.261538461538462,-0.246153846153846,
-0.230769230769231,-0.215384615384615,-0.2,-0.184615384615385,-0.169230769230769,
-0.153846153846154,-0.138461538461538,-0.123076923076923,-0.107692307692308,
-0.0923076923076923,-0.0769230769230769,-0.0615384615384615,-0.0461538461538462,
-0.0307692307692308,-0.0153846153846154,0.),.UNSPECIFIED.)
CURVE()
GEOMETRIC_REPRESENTATION_ITEM()
RATIONAL_B_SPLINE_CURVE((1.,1.,1.,1.,1.,1.,1.,1.,1.,1.,1.,1.,1.,1.,1.,1.,
1.,1.,1.,1.,1.,1.,1.,1.,1.,1.,1.,1.,1.,1.,1.,1.,1.,1.,1.,1.,1.,1.,1.,1.,
1.,1.,1.,1.,1.,1.,1.,1.,1.,1.,1.,1.,1.,1.,1.,1.,1.,1.,1.,1.,1.,1.,1.,1.,
1.,1.,1.,1.,1.,1.))
REPRESENTATION_ITEM('')
);
#302=(
BOUNDED_CURVE()
B_SPLINE_CURVE(5,(#43133,#43134,#43135,#43136,#43137,#43138,#43139,#43140,
#43141,#43142,#43143,#43144,#43145,#43146,#43147,#43148,#43149,#43150,#43151,
#43152,#43153,#43154,#43155,#43156,#43157,#43158,#43159,#43160,#43161,#43162,
#43163,#43164,#43165,#43166,#43167,#43168,#43169,#43170,#43171,#43172,#43173,
#43174,#43175,#43176,#43177,#43178,#43179,#43180,#43181,#43182,#43183,#43184,
#43185,#43186,#43187,#43188,#43189,#43190,#43191,#43192,#43193,#43194,#43195,
#43196,#43197,#43198,#43199,#43200,#43201,#43202),.UNSPECIFIED.,.F.,.F.)
B_SPLINE_CURVE_WITH_KNOTS((6,1,1,1,1,1,1,1,1,1,1,1,1,1,1,1,1,1,1,1,1,1,
1,1,1,1,1,1,1,1,1,1,1,1,1,1,1,1,1,1,1,1,1,1,1,1,1,1,1,1,1,1,1,1,1,1,1,1,
1,1,1,1,1,1,1,6),(-1.,-0.984615384615383,-0.969230769230768,-0.953846153846152,
-0.938461538461537,-0.923076923076922,-0.907692307692306,-0.892307692307691,
-0.876923076923076,-0.86153846153846,-0.846153846153845,-0.83076923076923,
-0.815384615384614,-0.799999999999999,-0.784615384615384,-0.769230769230768,
-0.753846153846153,-0.738461538461538,-0.723076923076922,-0.707692307692307,
-0.692307692307692,-0.676923076923076,-0.661538461538461,-0.646153846153846,
-0.63076923076923,-0.615384615384615,-0.6,-0.584615384615384,-0.569230769230769,
-0.553846153846154,-0.538461538461538,-0.523076923076923,-0.507692307692308,
-0.492307692307692,-0.476923076923077,-0.461538461538462,-0.446153846153846,
-0.430769230769231,-0.415384615384615,-0.4,-0.384615384615385,-0.369230769230769,
-0.353846153846154,-0.338461538461538,-0.323076923076923,-0.307692307692308,
-0.292307692307692,-0.276923076923077,-0.261538461538462,-0.246153846153846,
-0.230769230769231,-0.215384615384615,-0.2,-0.184615384615385,-0.169230769230769,
-0.153846153846154,-0.138461538461538,-0.123076923076923,-0.107692307692308,
-0.0923076923076923,-0.0769230769230769,-0.0615384615384615,-0.0461538461538462,
-0.0307692307692308,-0.0153846153846154,0.),.UNSPECIFIED.)
CURVE()
GEOMETRIC_REPRESENTATION_ITEM()
RATIONAL_B_SPLINE_CURVE((1.,1.,1.,1.,1.,1.,1.,1.,1.,1.,1.,1.,1.,1.,1.,1.,
1.,1.,1.,1.,1.,1.,1.,1.,1.,1.,1.,1.,1.,1.,1.,1.,1.,1.,1.,1.,1.,1.,1.,1.,
1.,1.,1.,1.,1.,1.,1.,1.,1.,1.,1.,1.,1.,1.,1.,1.,1.,1.,1.,1.,1.,1.,1.,1.,
1.,1.,1.,1.,1.,1.))
REPRESENTATION_ITEM('')
);
#303=(
BOUNDED_CURVE()
B_SPLINE_CURVE(5,(#43349,#43350,#43351,#43352,#43353,#43354,#43355,#43356,
#43357,#43358,#43359,#43360,#43361,#43362,#43363,#43364,#43365,#43366,#43367,
#43368,#43369,#43370,#43371,#43372,#43373,#43374,#43375,#43376,#43377,#43378,
#43379,#43380,#43381,#43382,#43383,#43384,#43385,#43386,#43387,#43388,#43389,
#43390,#43391,#43392,#43393,#43394,#43395,#43396,#43397,#43398,#43399,#43400,
#43401,#43402,#43403,#43404,#43405,#43406,#43407,#43408,#43409,#43410,#43411,
#43412,#43413,#43414,#43415,#43416,#43417,#43418),.UNSPECIFIED.,.F.,.F.)
B_SPLINE_CURVE_WITH_KNOTS((6,1,1,1,1,1,1,1,1,1,1,1,1,1,1,1,1,1,1,1,1,1,
1,1,1,1,1,1,1,1,1,1,1,1,1,1,1,1,1,1,1,1,1,1,1,1,1,1,1,1,1,1,1,1,1,1,1,1,
1,1,1,1,1,1,1,6),(-1.,-0.984615384615383,-0.969230769230768,-0.953846153846152,
-0.938461538461537,-0.923076923076922,-0.907692307692306,-0.892307692307691,
-0.876923076923076,-0.86153846153846,-0.846153846153845,-0.83076923076923,
-0.815384615384614,-0.799999999999999,-0.784615384615384,-0.769230769230768,
-0.753846153846153,-0.738461538461538,-0.723076923076922,-0.707692307692307,
-0.692307692307692,-0.676923076923076,-0.661538461538461,-0.646153846153846,
-0.63076923076923,-0.615384615384615,-0.6,-0.584615384615384,-0.569230769230769,
-0.553846153846154,-0.538461538461538,-0.523076923076923,-0.507692307692308,
-0.492307692307692,-0.476923076923077,-0.461538461538462,-0.446153846153846,
-0.430769230769231,-0.415384615384615,-0.4,-0.384615384615385,-0.369230769230769,
-0.353846153846154,-0.338461538461538,-0.323076923076923,-0.307692307692308,
-0.292307692307692,-0.276923076923077,-0.261538461538462,-0.246153846153846,
-0.230769230769231,-0.215384615384615,-0.2,-0.184615384615385,-0.169230769230769,
-0.153846153846154,-0.138461538461538,-0.123076923076923,-0.107692307692308,
-0.0923076923076923,-0.0769230769230769,-0.0615384615384615,-0.0461538461538462,
-0.0307692307692308,-0.0153846153846154,0.),.UNSPECIFIED.)
CURVE()
GEOMETRIC_REPRESENTATION_ITEM()
RATIONAL_B_SPLINE_CURVE((1.,1.,1.,1.,1.,1.,1.,1.,1.,1.,1.,1.,1.,1.,1.,1.,
1.,1.,1.,1.,1.,1.,1.,1.,1.,1.,1.,1.,1.,1.,1.,1.,1.,1.,1.,1.,1.,1.,1.,1.,
1.,1.,1.,1.,1.,1.,1.,1.,1.,1.,1.,1.,1.,1.,1.,1.,1.,1.,1.,1.,1.,1.,1.,1.,
1.,1.,1.,1.,1.,1.))
REPRESENTATION_ITEM('')
);
#304=(
BOUNDED_CURVE()
B_SPLINE_CURVE(5,(#43565,#43566,#43567,#43568,#43569,#43570,#43571,#43572,
#43573,#43574,#43575,#43576,#43577,#43578,#43579,#43580,#43581,#43582,#43583,
#43584,#43585,#43586,#43587,#43588,#43589,#43590,#43591,#43592,#43593,#43594,
#43595,#43596,#43597,#43598,#43599,#43600,#43601,#43602,#43603,#43604,#43605,
#43606,#43607,#43608,#43609,#43610,#43611,#43612,#43613,#43614,#43615,#43616,
#43617,#43618,#43619,#43620,#43621,#43622,#43623,#43624,#43625,#43626,#43627,
#43628,#43629,#43630,#43631,#43632,#43633,#43634),.UNSPECIFIED.,.F.,.F.)
B_SPLINE_CURVE_WITH_KNOTS((6,1,1,1,1,1,1,1,1,1,1,1,1,1,1,1,1,1,1,1,1,1,
1,1,1,1,1,1,1,1,1,1,1,1,1,1,1,1,1,1,1,1,1,1,1,1,1,1,1,1,1,1,1,1,1,1,1,1,
1,1,1,1,1,1,1,6),(-1.,-0.984615384615383,-0.969230769230768,-0.953846153846152,
-0.938461538461537,-0.923076923076922,-0.907692307692306,-0.892307692307691,
-0.876923076923076,-0.86153846153846,-0.846153846153845,-0.83076923076923,
-0.815384615384614,-0.799999999999999,-0.784615384615384,-0.769230769230768,
-0.753846153846153,-0.738461538461538,-0.723076923076922,-0.707692307692307,
-0.692307692307692,-0.676923076923076,-0.661538461538461,-0.646153846153846,
-0.63076923076923,-0.615384615384615,-0.6,-0.584615384615384,-0.569230769230769,
-0.553846153846154,-0.538461538461538,-0.523076923076923,-0.507692307692308,
-0.492307692307692,-0.476923076923077,-0.461538461538462,-0.446153846153846,
-0.430769230769231,-0.415384615384615,-0.4,-0.384615384615385,-0.369230769230769,
-0.353846153846154,-0.338461538461538,-0.323076923076923,-0.307692307692308,
-0.292307692307692,-0.276923076923077,-0.261538461538462,-0.246153846153846,
-0.230769230769231,-0.215384615384615,-0.2,-0.184615384615385,-0.169230769230769,
-0.153846153846154,-0.138461538461538,-0.123076923076923,-0.107692307692308,
-0.0923076923076923,-0.0769230769230769,-0.0615384615384615,-0.0461538461538462,
-0.0307692307692308,-0.0153846153846154,0.),.UNSPECIFIED.)
CURVE()
GEOMETRIC_REPRESENTATION_ITEM()
RATIONAL_B_SPLINE_CURVE((1.,1.,1.,1.,1.,1.,1.,1.,1.,1.,1.,1.,1.,1.,1.,1.,
1.,1.,1.,1.,1.,1.,1.,1.,1.,1.,1.,1.,1.,1.,1.,1.,1.,1.,1.,1.,1.,1.,1.,1.,
1.,1.,1.,1.,1.,1.,1.,1.,1.,1.,1.,1.,1.,1.,1.,1.,1.,1.,1.,1.,1.,1.,1.,1.,
1.,1.,1.,1.,1.,1.))
REPRESENTATION_ITEM('')
);
#305=(
BOUNDED_CURVE()
B_SPLINE_CURVE(5,(#43781,#43782,#43783,#43784,#43785,#43786,#43787,#43788,
#43789,#43790,#43791,#43792,#43793,#43794,#43795,#43796,#43797,#43798,#43799,
#43800,#43801,#43802,#43803,#43804,#43805,#43806,#43807,#43808,#43809,#43810,
#43811,#43812,#43813,#43814,#43815,#43816,#43817,#43818,#43819,#43820,#43821,
#43822,#43823,#43824,#43825,#43826,#43827,#43828,#43829,#43830,#43831,#43832,
#43833,#43834,#43835,#43836,#43837,#43838,#43839,#43840,#43841,#43842,#43843,
#43844,#43845,#43846,#43847,#43848,#43849,#43850),.UNSPECIFIED.,.F.,.F.)
B_SPLINE_CURVE_WITH_KNOTS((6,1,1,1,1,1,1,1,1,1,1,1,1,1,1,1,1,1,1,1,1,1,
1,1,1,1,1,1,1,1,1,1,1,1,1,1,1,1,1,1,1,1,1,1,1,1,1,1,1,1,1,1,1,1,1,1,1,1,
1,1,1,1,1,1,1,6),(-1.,-0.984615384615383,-0.969230769230768,-0.953846153846152,
-0.938461538461537,-0.923076923076922,-0.907692307692306,-0.892307692307691,
-0.876923076923076,-0.86153846153846,-0.846153846153845,-0.83076923076923,
-0.815384615384614,-0.799999999999999,-0.784615384615384,-0.769230769230768,
-0.753846153846153,-0.738461538461538,-0.723076923076922,-0.707692307692307,
-0.692307692307692,-0.676923076923076,-0.661538461538461,-0.646153846153846,
-0.63076923076923,-0.615384615384615,-0.6,-0.584615384615384,-0.569230769230769,
-0.553846153846154,-0.538461538461538,-0.523076923076923,-0.507692307692308,
-0.492307692307692,-0.476923076923077,-0.461538461538462,-0.446153846153846,
-0.430769230769231,-0.415384615384615,-0.4,-0.384615384615385,-0.369230769230769,
-0.353846153846154,-0.338461538461538,-0.323076923076923,-0.307692307692308,
-0.292307692307692,-0.276923076923077,-0.261538461538462,-0.246153846153846,
-0.230769230769231,-0.215384615384615,-0.2,-0.184615384615385,-0.169230769230769,
-0.153846153846154,-0.138461538461538,-0.123076923076923,-0.107692307692308,
-0.0923076923076923,-0.0769230769230769,-0.0615384615384615,-0.0461538461538462,
-0.0307692307692308,-0.0153846153846154,0.),.UNSPECIFIED.)
CURVE()
GEOMETRIC_REPRESENTATION_ITEM()
RATIONAL_B_SPLINE_CURVE((1.,1.,1.,1.,1.,1.,1.,1.,1.,1.,1.,1.,1.,1.,1.,1.,
1.,1.,1.,1.,1.,1.,1.,1.,1.,1.,1.,1.,1.,1.,1.,1.,1.,1.,1.,1.,1.,1.,1.,1.,
1.,1.,1.,1.,1.,1.,1.,1.,1.,1.,1.,1.,1.,1.,1.,1.,1.,1.,1.,1.,1.,1.,1.,1.,
1.,1.,1.,1.,1.,1.))
REPRESENTATION_ITEM('')
);
#306=(
BOUNDED_CURVE()
B_SPLINE_CURVE(5,(#43997,#43998,#43999,#44000,#44001,#44002,#44003,#44004,
#44005,#44006,#44007,#44008,#44009,#44010,#44011,#44012,#44013,#44014,#44015,
#44016,#44017,#44018,#44019,#44020,#44021,#44022,#44023,#44024,#44025,#44026,
#44027,#44028,#44029,#44030,#44031,#44032,#44033,#44034,#44035,#44036,#44037,
#44038,#44039,#44040,#44041,#44042,#44043,#44044,#44045,#44046,#44047,#44048,
#44049,#44050,#44051,#44052,#44053,#44054,#44055,#44056,#44057,#44058,#44059,
#44060,#44061,#44062,#44063,#44064,#44065,#44066),.UNSPECIFIED.,.F.,.F.)
B_SPLINE_CURVE_WITH_KNOTS((6,1,1,1,1,1,1,1,1,1,1,1,1,1,1,1,1,1,1,1,1,1,
1,1,1,1,1,1,1,1,1,1,1,1,1,1,1,1,1,1,1,1,1,1,1,1,1,1,1,1,1,1,1,1,1,1,1,1,
1,1,1,1,1,1,1,6),(-1.,-0.984615384615383,-0.969230769230768,-0.953846153846152,
-0.938461538461537,-0.923076923076922,-0.907692307692306,-0.892307692307691,
-0.876923076923076,-0.86153846153846,-0.846153846153845,-0.83076923076923,
-0.815384615384614,-0.799999999999999,-0.784615384615384,-0.769230769230768,
-0.753846153846153,-0.738461538461538,-0.723076923076922,-0.707692307692307,
-0.692307692307692,-0.676923076923076,-0.661538461538461,-0.646153846153846,
-0.63076923076923,-0.615384615384615,-0.6,-0.584615384615384,-0.569230769230769,
-0.553846153846154,-0.538461538461538,-0.523076923076923,-0.507692307692308,
-0.492307692307692,-0.476923076923077,-0.461538461538462,-0.446153846153846,
-0.430769230769231,-0.415384615384615,-0.4,-0.384615384615385,-0.369230769230769,
-0.353846153846154,-0.338461538461538,-0.323076923076923,-0.307692307692308,
-0.292307692307692,-0.276923076923077,-0.261538461538462,-0.246153846153846,
-0.230769230769231,-0.215384615384615,-0.2,-0.184615384615385,-0.169230769230769,
-0.153846153846154,-0.138461538461538,-0.123076923076923,-0.107692307692308,
-0.0923076923076923,-0.0769230769230769,-0.0615384615384615,-0.0461538461538462,
-0.0307692307692308,-0.0153846153846154,0.),.UNSPECIFIED.)
CURVE()
GEOMETRIC_REPRESENTATION_ITEM()
RATIONAL_B_SPLINE_CURVE((1.,1.,1.,1.,1.,1.,1.,1.,1.,1.,1.,1.,1.,1.,1.,1.,
1.,1.,1.,1.,1.,1.,1.,1.,1.,1.,1.,1.,1.,1.,1.,1.,1.,1.,1.,1.,1.,1.,1.,1.,
1.,1.,1.,1.,1.,1.,1.,1.,1.,1.,1.,1.,1.,1.,1.,1.,1.,1.,1.,1.,1.,1.,1.,1.,
1.,1.,1.,1.,1.,1.))
REPRESENTATION_ITEM('')
);
#307=(
BOUNDED_CURVE()
B_SPLINE_CURVE(5,(#44213,#44214,#44215,#44216,#44217,#44218,#44219,#44220,
#44221,#44222,#44223,#44224,#44225,#44226,#44227,#44228,#44229,#44230,#44231,
#44232,#44233,#44234,#44235,#44236,#44237,#44238,#44239,#44240,#44241,#44242,
#44243,#44244,#44245,#44246,#44247,#44248,#44249,#44250,#44251,#44252,#44253,
#44254,#44255,#44256,#44257,#44258,#44259,#44260,#44261,#44262,#44263,#44264,
#44265,#44266,#44267,#44268,#44269,#44270,#44271,#44272,#44273,#44274,#44275,
#44276,#44277,#44278,#44279,#44280,#44281,#44282),.UNSPECIFIED.,.F.,.F.)
B_SPLINE_CURVE_WITH_KNOTS((6,1,1,1,1,1,1,1,1,1,1,1,1,1,1,1,1,1,1,1,1,1,
1,1,1,1,1,1,1,1,1,1,1,1,1,1,1,1,1,1,1,1,1,1,1,1,1,1,1,1,1,1,1,1,1,1,1,1,
1,1,1,1,1,1,1,6),(-1.,-0.984615384615383,-0.969230769230768,-0.953846153846152,
-0.938461538461537,-0.923076923076922,-0.907692307692306,-0.892307692307691,
-0.876923076923076,-0.86153846153846,-0.846153846153845,-0.83076923076923,
-0.815384615384614,-0.799999999999999,-0.784615384615384,-0.769230769230768,
-0.753846153846153,-0.738461538461538,-0.723076923076922,-0.707692307692307,
-0.692307692307692,-0.676923076923076,-0.661538461538461,-0.646153846153846,
-0.63076923076923,-0.615384615384615,-0.6,-0.584615384615384,-0.569230769230769,
-0.553846153846154,-0.538461538461538,-0.523076923076923,-0.507692307692308,
-0.492307692307692,-0.476923076923077,-0.461538461538462,-0.446153846153846,
-0.430769230769231,-0.415384615384615,-0.4,-0.384615384615385,-0.369230769230769,
-0.353846153846154,-0.338461538461538,-0.323076923076923,-0.307692307692308,
-0.292307692307692,-0.276923076923077,-0.261538461538462,-0.246153846153846,
-0.230769230769231,-0.215384615384615,-0.2,-0.184615384615385,-0.169230769230769,
-0.153846153846154,-0.138461538461538,-0.123076923076923,-0.107692307692308,
-0.0923076923076923,-0.0769230769230769,-0.0615384615384615,-0.0461538461538462,
-0.0307692307692308,-0.0153846153846154,0.),.UNSPECIFIED.)
CURVE()
GEOMETRIC_REPRESENTATION_ITEM()
RATIONAL_B_SPLINE_CURVE((1.,1.,1.,1.,1.,1.,1.,1.,1.,1.,1.,1.,1.,1.,1.,1.,
1.,1.,1.,1.,1.,1.,1.,1.,1.,1.,1.,1.,1.,1.,1.,1.,1.,1.,1.,1.,1.,1.,1.,1.,
1.,1.,1.,1.,1.,1.,1.,1.,1.,1.,1.,1.,1.,1.,1.,1.,1.,1.,1.,1.,1.,1.,1.,1.,
1.,1.,1.,1.,1.,1.))
REPRESENTATION_ITEM('')
);
#308=(
BOUNDED_CURVE()
B_SPLINE_CURVE(5,(#44429,#44430,#44431,#44432,#44433,#44434,#44435,#44436,
#44437,#44438,#44439,#44440,#44441,#44442,#44443,#44444,#44445,#44446,#44447,
#44448,#44449,#44450,#44451,#44452,#44453,#44454,#44455,#44456,#44457,#44458,
#44459,#44460,#44461,#44462,#44463,#44464,#44465,#44466,#44467,#44468,#44469,
#44470,#44471,#44472,#44473,#44474,#44475,#44476,#44477,#44478,#44479,#44480,
#44481,#44482,#44483,#44484,#44485,#44486,#44487,#44488,#44489,#44490,#44491,
#44492,#44493,#44494,#44495,#44496,#44497,#44498),.UNSPECIFIED.,.F.,.F.)
B_SPLINE_CURVE_WITH_KNOTS((6,1,1,1,1,1,1,1,1,1,1,1,1,1,1,1,1,1,1,1,1,1,
1,1,1,1,1,1,1,1,1,1,1,1,1,1,1,1,1,1,1,1,1,1,1,1,1,1,1,1,1,1,1,1,1,1,1,1,
1,1,1,1,1,1,1,6),(-1.,-0.984615384615383,-0.969230769230768,-0.953846153846152,
-0.938461538461537,-0.923076923076922,-0.907692307692306,-0.892307692307691,
-0.876923076923076,-0.86153846153846,-0.846153846153845,-0.83076923076923,
-0.815384615384614,-0.799999999999999,-0.784615384615384,-0.769230769230768,
-0.753846153846153,-0.738461538461538,-0.723076923076922,-0.707692307692307,
-0.692307692307692,-0.676923076923076,-0.661538461538461,-0.646153846153846,
-0.63076923076923,-0.615384615384615,-0.6,-0.584615384615384,-0.569230769230769,
-0.553846153846154,-0.538461538461538,-0.523076923076923,-0.507692307692308,
-0.492307692307692,-0.476923076923077,-0.461538461538462,-0.446153846153846,
-0.430769230769231,-0.415384615384615,-0.4,-0.384615384615385,-0.369230769230769,
-0.353846153846154,-0.338461538461538,-0.323076923076923,-0.307692307692308,
-0.292307692307692,-0.276923076923077,-0.261538461538462,-0.246153846153846,
-0.230769230769231,-0.215384615384615,-0.2,-0.184615384615385,-0.169230769230769,
-0.153846153846154,-0.138461538461538,-0.123076923076923,-0.107692307692308,
-0.0923076923076923,-0.0769230769230769,-0.0615384615384615,-0.0461538461538462,
-0.0307692307692308,-0.0153846153846154,0.),.UNSPECIFIED.)
CURVE()
GEOMETRIC_REPRESENTATION_ITEM()
RATIONAL_B_SPLINE_CURVE((1.,1.,1.,1.,1.,1.,1.,1.,1.,1.,1.,1.,1.,1.,1.,1.,
1.,1.,1.,1.,1.,1.,1.,1.,1.,1.,1.,1.,1.,1.,1.,1.,1.,1.,1.,1.,1.,1.,1.,1.,
1.,1.,1.,1.,1.,1.,1.,1.,1.,1.,1.,1.,1.,1.,1.,1.,1.,1.,1.,1.,1.,1.,1.,1.,
1.,1.,1.,1.,1.,1.))
REPRESENTATION_ITEM('')
);
#309=(
BOUNDED_CURVE()
B_SPLINE_CURVE(5,(#44645,#44646,#44647,#44648,#44649,#44650,#44651,#44652,
#44653,#44654,#44655,#44656,#44657,#44658,#44659,#44660,#44661,#44662,#44663,
#44664,#44665,#44666,#44667,#44668,#44669,#44670,#44671,#44672,#44673,#44674,
#44675,#44676,#44677,#44678,#44679,#44680,#44681,#44682,#44683,#44684,#44685,
#44686,#44687,#44688,#44689,#44690,#44691,#44692,#44693,#44694,#44695,#44696,
#44697,#44698,#44699,#44700,#44701,#44702,#44703,#44704,#44705,#44706,#44707,
#44708,#44709,#44710,#44711,#44712,#44713,#44714),.UNSPECIFIED.,.F.,.F.)
B_SPLINE_CURVE_WITH_KNOTS((6,1,1,1,1,1,1,1,1,1,1,1,1,1,1,1,1,1,1,1,1,1,
1,1,1,1,1,1,1,1,1,1,1,1,1,1,1,1,1,1,1,1,1,1,1,1,1,1,1,1,1,1,1,1,1,1,1,1,
1,1,1,1,1,1,1,6),(-1.,-0.984615384615383,-0.969230769230768,-0.953846153846152,
-0.938461538461537,-0.923076923076922,-0.907692307692306,-0.892307692307691,
-0.876923076923076,-0.86153846153846,-0.846153846153845,-0.83076923076923,
-0.815384615384614,-0.799999999999999,-0.784615384615384,-0.769230769230768,
-0.753846153846153,-0.738461538461538,-0.723076923076922,-0.707692307692307,
-0.692307692307692,-0.676923076923076,-0.661538461538461,-0.646153846153846,
-0.63076923076923,-0.615384615384615,-0.6,-0.584615384615384,-0.569230769230769,
-0.553846153846154,-0.538461538461538,-0.523076923076923,-0.507692307692308,
-0.492307692307692,-0.476923076923077,-0.461538461538462,-0.446153846153846,
-0.430769230769231,-0.415384615384615,-0.4,-0.384615384615385,-0.369230769230769,
-0.353846153846154,-0.338461538461538,-0.323076923076923,-0.307692307692308,
-0.292307692307692,-0.276923076923077,-0.261538461538462,-0.246153846153846,
-0.230769230769231,-0.215384615384615,-0.2,-0.184615384615385,-0.169230769230769,
-0.153846153846154,-0.138461538461538,-0.123076923076923,-0.107692307692308,
-0.0923076923076923,-0.0769230769230769,-0.0615384615384615,-0.0461538461538462,
-0.0307692307692308,-0.0153846153846154,0.),.UNSPECIFIED.)
CURVE()
GEOMETRIC_REPRESENTATION_ITEM()
RATIONAL_B_SPLINE_CURVE((1.,1.,1.,1.,1.,1.,1.,1.,1.,1.,1.,1.,1.,1.,1.,1.,
1.,1.,1.,1.,1.,1.,1.,1.,1.,1.,1.,1.,1.,1.,1.,1.,1.,1.,1.,1.,1.,1.,1.,1.,
1.,1.,1.,1.,1.,1.,1.,1.,1.,1.,1.,1.,1.,1.,1.,1.,1.,1.,1.,1.,1.,1.,1.,1.,
1.,1.,1.,1.,1.,1.))
REPRESENTATION_ITEM('')
);
#310=(
BOUNDED_CURVE()
B_SPLINE_CURVE(5,(#44861,#44862,#44863,#44864,#44865,#44866,#44867,#44868,
#44869,#44870,#44871,#44872,#44873,#44874,#44875,#44876,#44877,#44878,#44879,
#44880,#44881,#44882,#44883,#44884,#44885,#44886,#44887,#44888,#44889,#44890,
#44891,#44892,#44893,#44894,#44895,#44896,#44897,#44898,#44899,#44900,#44901,
#44902,#44903,#44904,#44905,#44906,#44907,#44908,#44909,#44910,#44911,#44912,
#44913,#44914,#44915,#44916,#44917,#44918,#44919,#44920,#44921,#44922,#44923,
#44924,#44925,#44926,#44927,#44928,#44929,#44930),.UNSPECIFIED.,.F.,.F.)
B_SPLINE_CURVE_WITH_KNOTS((6,1,1,1,1,1,1,1,1,1,1,1,1,1,1,1,1,1,1,1,1,1,
1,1,1,1,1,1,1,1,1,1,1,1,1,1,1,1,1,1,1,1,1,1,1,1,1,1,1,1,1,1,1,1,1,1,1,1,
1,1,1,1,1,1,1,6),(-1.,-0.984615384615383,-0.969230769230768,-0.953846153846152,
-0.938461538461537,-0.923076923076922,-0.907692307692306,-0.892307692307691,
-0.876923076923076,-0.86153846153846,-0.846153846153845,-0.83076923076923,
-0.815384615384614,-0.799999999999999,-0.784615384615384,-0.769230769230768,
-0.753846153846153,-0.738461538461538,-0.723076923076922,-0.707692307692307,
-0.692307692307692,-0.676923076923076,-0.661538461538461,-0.646153846153846,
-0.63076923076923,-0.615384615384615,-0.6,-0.584615384615384,-0.569230769230769,
-0.553846153846154,-0.538461538461538,-0.523076923076923,-0.507692307692308,
-0.492307692307692,-0.476923076923077,-0.461538461538462,-0.446153846153846,
-0.430769230769231,-0.415384615384615,-0.4,-0.384615384615385,-0.369230769230769,
-0.353846153846154,-0.338461538461538,-0.323076923076923,-0.307692307692308,
-0.292307692307692,-0.276923076923077,-0.261538461538462,-0.246153846153846,
-0.230769230769231,-0.215384615384615,-0.2,-0.184615384615385,-0.169230769230769,
-0.153846153846154,-0.138461538461538,-0.123076923076923,-0.107692307692308,
-0.0923076923076923,-0.0769230769230769,-0.0615384615384615,-0.0461538461538462,
-0.0307692307692308,-0.0153846153846154,0.),.UNSPECIFIED.)
CURVE()
GEOMETRIC_REPRESENTATION_ITEM()
RATIONAL_B_SPLINE_CURVE((1.,1.,1.,1.,1.,1.,1.,1.,1.,1.,1.,1.,1.,1.,1.,1.,
1.,1.,1.,1.,1.,1.,1.,1.,1.,1.,1.,1.,1.,1.,1.,1.,1.,1.,1.,1.,1.,1.,1.,1.,
1.,1.,1.,1.,1.,1.,1.,1.,1.,1.,1.,1.,1.,1.,1.,1.,1.,1.,1.,1.,1.,1.,1.,1.,
1.,1.,1.,1.,1.,1.))
REPRESENTATION_ITEM('')
);
#311=(
BOUNDED_CURVE()
B_SPLINE_CURVE(5,(#45077,#45078,#45079,#45080,#45081,#45082,#45083,#45084,
#45085,#45086,#45087,#45088,#45089,#45090,#45091,#45092,#45093,#45094,#45095,
#45096,#45097,#45098,#45099,#45100,#45101,#45102,#45103,#45104,#45105,#45106,
#45107,#45108,#45109,#45110,#45111,#45112,#45113,#45114,#45115,#45116,#45117,
#45118,#45119,#45120,#45121,#45122,#45123,#45124,#45125,#45126,#45127,#45128,
#45129,#45130,#45131,#45132,#45133,#45134,#45135,#45136,#45137,#45138,#45139,
#45140,#45141,#45142,#45143,#45144,#45145,#45146),.UNSPECIFIED.,.F.,.F.)
B_SPLINE_CURVE_WITH_KNOTS((6,1,1,1,1,1,1,1,1,1,1,1,1,1,1,1,1,1,1,1,1,1,
1,1,1,1,1,1,1,1,1,1,1,1,1,1,1,1,1,1,1,1,1,1,1,1,1,1,1,1,1,1,1,1,1,1,1,1,
1,1,1,1,1,1,1,6),(-1.,-0.984615384615383,-0.969230769230768,-0.953846153846152,
-0.938461538461537,-0.923076923076922,-0.907692307692306,-0.892307692307691,
-0.876923076923076,-0.86153846153846,-0.846153846153845,-0.83076923076923,
-0.815384615384614,-0.799999999999999,-0.784615384615384,-0.769230769230768,
-0.753846153846153,-0.738461538461538,-0.723076923076922,-0.707692307692307,
-0.692307692307692,-0.676923076923076,-0.661538461538461,-0.646153846153846,
-0.63076923076923,-0.615384615384615,-0.6,-0.584615384615384,-0.569230769230769,
-0.553846153846154,-0.538461538461538,-0.523076923076923,-0.507692307692308,
-0.492307692307692,-0.476923076923077,-0.461538461538462,-0.446153846153846,
-0.430769230769231,-0.415384615384615,-0.4,-0.384615384615385,-0.369230769230769,
-0.353846153846154,-0.338461538461538,-0.323076923076923,-0.307692307692308,
-0.292307692307692,-0.276923076923077,-0.261538461538462,-0.246153846153846,
-0.230769230769231,-0.215384615384615,-0.2,-0.184615384615385,-0.169230769230769,
-0.153846153846154,-0.138461538461538,-0.123076923076923,-0.107692307692308,
-0.0923076923076923,-0.0769230769230769,-0.0615384615384615,-0.0461538461538462,
-0.0307692307692308,-0.0153846153846154,0.),.UNSPECIFIED.)
CURVE()
GEOMETRIC_REPRESENTATION_ITEM()
RATIONAL_B_SPLINE_CURVE((1.,1.,1.,1.,1.,1.,1.,1.,1.,1.,1.,1.,1.,1.,1.,1.,
1.,1.,1.,1.,1.,1.,1.,1.,1.,1.,1.,1.,1.,1.,1.,1.,1.,1.,1.,1.,1.,1.,1.,1.,
1.,1.,1.,1.,1.,1.,1.,1.,1.,1.,1.,1.,1.,1.,1.,1.,1.,1.,1.,1.,1.,1.,1.,1.,
1.,1.,1.,1.,1.,1.))
REPRESENTATION_ITEM('')
);
#312=(
BOUNDED_CURVE()
B_SPLINE_CURVE(5,(#45293,#45294,#45295,#45296,#45297,#45298,#45299,#45300,
#45301,#45302,#45303,#45304,#45305,#45306,#45307,#45308,#45309,#45310,#45311,
#45312,#45313,#45314,#45315,#45316,#45317,#45318,#45319,#45320,#45321,#45322,
#45323,#45324,#45325,#45326,#45327,#45328,#45329,#45330,#45331,#45332,#45333,
#45334,#45335,#45336,#45337,#45338,#45339,#45340,#45341,#45342,#45343,#45344,
#45345,#45346,#45347,#45348,#45349,#45350,#45351,#45352,#45353,#45354,#45355,
#45356,#45357,#45358,#45359,#45360,#45361,#45362),.UNSPECIFIED.,.F.,.F.)
B_SPLINE_CURVE_WITH_KNOTS((6,1,1,1,1,1,1,1,1,1,1,1,1,1,1,1,1,1,1,1,1,1,
1,1,1,1,1,1,1,1,1,1,1,1,1,1,1,1,1,1,1,1,1,1,1,1,1,1,1,1,1,1,1,1,1,1,1,1,
1,1,1,1,1,1,1,6),(-1.,-0.984615384615383,-0.969230769230768,-0.953846153846152,
-0.938461538461537,-0.923076923076922,-0.907692307692306,-0.892307692307691,
-0.876923076923076,-0.86153846153846,-0.846153846153845,-0.83076923076923,
-0.815384615384614,-0.799999999999999,-0.784615384615384,-0.769230769230768,
-0.753846153846153,-0.738461538461538,-0.723076923076922,-0.707692307692307,
-0.692307692307692,-0.676923076923076,-0.661538461538461,-0.646153846153846,
-0.63076923076923,-0.615384615384615,-0.6,-0.584615384615384,-0.569230769230769,
-0.553846153846154,-0.538461538461538,-0.523076923076923,-0.507692307692308,
-0.492307692307692,-0.476923076923077,-0.461538461538462,-0.446153846153846,
-0.430769230769231,-0.415384615384615,-0.4,-0.384615384615385,-0.369230769230769,
-0.353846153846154,-0.338461538461538,-0.323076923076923,-0.307692307692308,
-0.292307692307692,-0.276923076923077,-0.261538461538462,-0.246153846153846,
-0.230769230769231,-0.215384615384615,-0.2,-0.184615384615385,-0.169230769230769,
-0.153846153846154,-0.138461538461538,-0.123076923076923,-0.107692307692308,
-0.0923076923076923,-0.0769230769230769,-0.0615384615384615,-0.0461538461538462,
-0.0307692307692308,-0.0153846153846154,0.),.UNSPECIFIED.)
CURVE()
GEOMETRIC_REPRESENTATION_ITEM()
RATIONAL_B_SPLINE_CURVE((1.,1.,1.,1.,1.,1.,1.,1.,1.,1.,1.,1.,1.,1.,1.,1.,
1.,1.,1.,1.,1.,1.,1.,1.,1.,1.,1.,1.,1.,1.,1.,1.,1.,1.,1.,1.,1.,1.,1.,1.,
1.,1.,1.,1.,1.,1.,1.,1.,1.,1.,1.,1.,1.,1.,1.,1.,1.,1.,1.,1.,1.,1.,1.,1.,
1.,1.,1.,1.,1.,1.))
REPRESENTATION_ITEM('')
);
#313=(
BOUNDED_CURVE()
B_SPLINE_CURVE(5,(#45509,#45510,#45511,#45512,#45513,#45514,#45515,#45516,
#45517,#45518,#45519,#45520,#45521,#45522,#45523,#45524,#45525,#45526,#45527,
#45528,#45529,#45530,#45531,#45532,#45533,#45534,#45535,#45536,#45537,#45538,
#45539,#45540,#45541,#45542,#45543,#45544,#45545,#45546,#45547,#45548,#45549,
#45550,#45551,#45552,#45553,#45554,#45555,#45556,#45557,#45558,#45559,#45560,
#45561,#45562,#45563,#45564,#45565,#45566,#45567,#45568,#45569,#45570,#45571,
#45572,#45573,#45574,#45575,#45576,#45577,#45578),.UNSPECIFIED.,.F.,.F.)
B_SPLINE_CURVE_WITH_KNOTS((6,1,1,1,1,1,1,1,1,1,1,1,1,1,1,1,1,1,1,1,1,1,
1,1,1,1,1,1,1,1,1,1,1,1,1,1,1,1,1,1,1,1,1,1,1,1,1,1,1,1,1,1,1,1,1,1,1,1,
1,1,1,1,1,1,1,6),(-1.,-0.984615384615383,-0.969230769230768,-0.953846153846152,
-0.938461538461537,-0.923076923076922,-0.907692307692306,-0.892307692307691,
-0.876923076923076,-0.86153846153846,-0.846153846153845,-0.83076923076923,
-0.815384615384614,-0.799999999999999,-0.784615384615384,-0.769230769230768,
-0.753846153846153,-0.738461538461538,-0.723076923076922,-0.707692307692307,
-0.692307692307692,-0.676923076923076,-0.661538461538461,-0.646153846153846,
-0.63076923076923,-0.615384615384615,-0.6,-0.584615384615384,-0.569230769230769,
-0.553846153846154,-0.538461538461538,-0.523076923076923,-0.507692307692308,
-0.492307692307692,-0.476923076923077,-0.461538461538462,-0.446153846153846,
-0.430769230769231,-0.415384615384615,-0.4,-0.384615384615385,-0.369230769230769,
-0.353846153846154,-0.338461538461538,-0.323076923076923,-0.307692307692308,
-0.292307692307692,-0.276923076923077,-0.261538461538462,-0.246153846153846,
-0.230769230769231,-0.215384615384615,-0.2,-0.184615384615385,-0.169230769230769,
-0.153846153846154,-0.138461538461538,-0.123076923076923,-0.107692307692308,
-0.0923076923076923,-0.0769230769230769,-0.0615384615384615,-0.0461538461538462,
-0.0307692307692308,-0.0153846153846154,0.),.UNSPECIFIED.)
CURVE()
GEOMETRIC_REPRESENTATION_ITEM()
RATIONAL_B_SPLINE_CURVE((1.,1.,1.,1.,1.,1.,1.,1.,1.,1.,1.,1.,1.,1.,1.,1.,
1.,1.,1.,1.,1.,1.,1.,1.,1.,1.,1.,1.,1.,1.,1.,1.,1.,1.,1.,1.,1.,1.,1.,1.,
1.,1.,1.,1.,1.,1.,1.,1.,1.,1.,1.,1.,1.,1.,1.,1.,1.,1.,1.,1.,1.,1.,1.,1.,
1.,1.,1.,1.,1.,1.))
REPRESENTATION_ITEM('')
);
#314=(
BOUNDED_CURVE()
B_SPLINE_CURVE(5,(#45725,#45726,#45727,#45728,#45729,#45730,#45731,#45732,
#45733,#45734,#45735,#45736,#45737,#45738,#45739,#45740,#45741,#45742,#45743,
#45744,#45745,#45746,#45747,#45748,#45749,#45750,#45751,#45752,#45753,#45754,
#45755,#45756,#45757,#45758,#45759,#45760,#45761,#45762,#45763,#45764,#45765,
#45766,#45767,#45768,#45769,#45770,#45771,#45772,#45773,#45774,#45775,#45776,
#45777,#45778,#45779,#45780,#45781,#45782,#45783,#45784,#45785,#45786,#45787,
#45788,#45789,#45790,#45791,#45792,#45793,#45794),.UNSPECIFIED.,.F.,.F.)
B_SPLINE_CURVE_WITH_KNOTS((6,1,1,1,1,1,1,1,1,1,1,1,1,1,1,1,1,1,1,1,1,1,
1,1,1,1,1,1,1,1,1,1,1,1,1,1,1,1,1,1,1,1,1,1,1,1,1,1,1,1,1,1,1,1,1,1,1,1,
1,1,1,1,1,1,1,6),(-1.,-0.984615384615383,-0.969230769230768,-0.953846153846152,
-0.938461538461537,-0.923076923076922,-0.907692307692306,-0.892307692307691,
-0.876923076923076,-0.86153846153846,-0.846153846153845,-0.83076923076923,
-0.815384615384614,-0.799999999999999,-0.784615384615384,-0.769230769230768,
-0.753846153846153,-0.738461538461538,-0.723076923076922,-0.707692307692307,
-0.692307692307692,-0.676923076923076,-0.661538461538461,-0.646153846153846,
-0.63076923076923,-0.615384615384615,-0.6,-0.584615384615384,-0.569230769230769,
-0.553846153846154,-0.538461538461538,-0.523076923076923,-0.507692307692308,
-0.492307692307692,-0.476923076923077,-0.461538461538462,-0.446153846153846,
-0.430769230769231,-0.415384615384615,-0.4,-0.384615384615385,-0.369230769230769,
-0.353846153846154,-0.338461538461538,-0.323076923076923,-0.307692307692308,
-0.292307692307692,-0.276923076923077,-0.261538461538462,-0.246153846153846,
-0.230769230769231,-0.215384615384615,-0.2,-0.184615384615385,-0.169230769230769,
-0.153846153846154,-0.138461538461538,-0.123076923076923,-0.107692307692308,
-0.0923076923076923,-0.0769230769230769,-0.0615384615384615,-0.0461538461538462,
-0.0307692307692308,-0.0153846153846154,0.),.UNSPECIFIED.)
CURVE()
GEOMETRIC_REPRESENTATION_ITEM()
RATIONAL_B_SPLINE_CURVE((1.,1.,1.,1.,1.,1.,1.,1.,1.,1.,1.,1.,1.,1.,1.,1.,
1.,1.,1.,1.,1.,1.,1.,1.,1.,1.,1.,1.,1.,1.,1.,1.,1.,1.,1.,1.,1.,1.,1.,1.,
1.,1.,1.,1.,1.,1.,1.,1.,1.,1.,1.,1.,1.,1.,1.,1.,1.,1.,1.,1.,1.,1.,1.,1.,
1.,1.,1.,1.,1.,1.))
REPRESENTATION_ITEM('')
);
#315=(
BOUNDED_CURVE()
B_SPLINE_CURVE(5,(#45941,#45942,#45943,#45944,#45945,#45946,#45947,#45948,
#45949,#45950,#45951,#45952,#45953,#45954,#45955,#45956,#45957,#45958,#45959,
#45960,#45961,#45962,#45963,#45964,#45965,#45966,#45967,#45968,#45969,#45970,
#45971,#45972,#45973,#45974,#45975,#45976,#45977,#45978,#45979,#45980,#45981,
#45982,#45983,#45984,#45985,#45986,#45987,#45988,#45989,#45990,#45991,#45992,
#45993,#45994,#45995,#45996,#45997,#45998,#45999,#46000,#46001,#46002,#46003,
#46004,#46005,#46006,#46007,#46008,#46009,#46010),.UNSPECIFIED.,.F.,.F.)
B_SPLINE_CURVE_WITH_KNOTS((6,1,1,1,1,1,1,1,1,1,1,1,1,1,1,1,1,1,1,1,1,1,
1,1,1,1,1,1,1,1,1,1,1,1,1,1,1,1,1,1,1,1,1,1,1,1,1,1,1,1,1,1,1,1,1,1,1,1,
1,1,1,1,1,1,1,6),(-1.,-0.984615384615383,-0.969230769230768,-0.953846153846152,
-0.938461538461537,-0.923076923076922,-0.907692307692306,-0.892307692307691,
-0.876923076923076,-0.86153846153846,-0.846153846153845,-0.83076923076923,
-0.815384615384614,-0.799999999999999,-0.784615384615384,-0.769230769230768,
-0.753846153846153,-0.738461538461538,-0.723076923076922,-0.707692307692307,
-0.692307692307692,-0.676923076923076,-0.661538461538461,-0.646153846153846,
-0.63076923076923,-0.615384615384615,-0.6,-0.584615384615384,-0.569230769230769,
-0.553846153846154,-0.538461538461538,-0.523076923076923,-0.507692307692308,
-0.492307692307692,-0.476923076923077,-0.461538461538462,-0.446153846153846,
-0.430769230769231,-0.415384615384615,-0.4,-0.384615384615385,-0.369230769230769,
-0.353846153846154,-0.338461538461538,-0.323076923076923,-0.307692307692308,
-0.292307692307692,-0.276923076923077,-0.261538461538462,-0.246153846153846,
-0.230769230769231,-0.215384615384615,-0.2,-0.184615384615385,-0.169230769230769,
-0.153846153846154,-0.138461538461538,-0.123076923076923,-0.107692307692308,
-0.0923076923076923,-0.0769230769230769,-0.0615384615384615,-0.0461538461538462,
-0.0307692307692308,-0.0153846153846154,0.),.UNSPECIFIED.)
CURVE()
GEOMETRIC_REPRESENTATION_ITEM()
RATIONAL_B_SPLINE_CURVE((1.,1.,1.,1.,1.,1.,1.,1.,1.,1.,1.,1.,1.,1.,1.,1.,
1.,1.,1.,1.,1.,1.,1.,1.,1.,1.,1.,1.,1.,1.,1.,1.,1.,1.,1.,1.,1.,1.,1.,1.,
1.,1.,1.,1.,1.,1.,1.,1.,1.,1.,1.,1.,1.,1.,1.,1.,1.,1.,1.,1.,1.,1.,1.,1.,
1.,1.,1.,1.,1.,1.))
REPRESENTATION_ITEM('')
);
#316=(
BOUNDED_CURVE()
B_SPLINE_CURVE(5,(#46157,#46158,#46159,#46160,#46161,#46162,#46163,#46164,
#46165,#46166,#46167,#46168,#46169,#46170,#46171,#46172,#46173,#46174,#46175,
#46176,#46177,#46178,#46179,#46180,#46181,#46182,#46183,#46184,#46185,#46186,
#46187,#46188,#46189,#46190,#46191,#46192,#46193,#46194,#46195,#46196,#46197,
#46198,#46199,#46200,#46201,#46202,#46203,#46204,#46205,#46206,#46207,#46208,
#46209,#46210,#46211,#46212,#46213,#46214,#46215,#46216,#46217,#46218,#46219,
#46220,#46221,#46222,#46223,#46224,#46225,#46226),.UNSPECIFIED.,.F.,.F.)
B_SPLINE_CURVE_WITH_KNOTS((6,1,1,1,1,1,1,1,1,1,1,1,1,1,1,1,1,1,1,1,1,1,
1,1,1,1,1,1,1,1,1,1,1,1,1,1,1,1,1,1,1,1,1,1,1,1,1,1,1,1,1,1,1,1,1,1,1,1,
1,1,1,1,1,1,1,6),(-1.,-0.984615384615383,-0.969230769230768,-0.953846153846152,
-0.938461538461537,-0.923076923076922,-0.907692307692306,-0.892307692307691,
-0.876923076923076,-0.86153846153846,-0.846153846153845,-0.83076923076923,
-0.815384615384614,-0.799999999999999,-0.784615384615384,-0.769230769230768,
-0.753846153846153,-0.738461538461538,-0.723076923076922,-0.707692307692307,
-0.692307692307692,-0.676923076923076,-0.661538461538461,-0.646153846153846,
-0.63076923076923,-0.615384615384615,-0.6,-0.584615384615384,-0.569230769230769,
-0.553846153846154,-0.538461538461538,-0.523076923076923,-0.507692307692308,
-0.492307692307692,-0.476923076923077,-0.461538461538462,-0.446153846153846,
-0.430769230769231,-0.415384615384615,-0.4,-0.384615384615385,-0.369230769230769,
-0.353846153846154,-0.338461538461538,-0.323076923076923,-0.307692307692308,
-0.292307692307692,-0.276923076923077,-0.261538461538462,-0.246153846153846,
-0.230769230769231,-0.215384615384615,-0.2,-0.184615384615385,-0.169230769230769,
-0.153846153846154,-0.138461538461538,-0.123076923076923,-0.107692307692308,
-0.0923076923076923,-0.0769230769230769,-0.0615384615384615,-0.0461538461538462,
-0.0307692307692308,-0.0153846153846154,0.),.UNSPECIFIED.)
CURVE()
GEOMETRIC_REPRESENTATION_ITEM()
RATIONAL_B_SPLINE_CURVE((1.,1.,1.,1.,1.,1.,1.,1.,1.,1.,1.,1.,1.,1.,1.,1.,
1.,1.,1.,1.,1.,1.,1.,1.,1.,1.,1.,1.,1.,1.,1.,1.,1.,1.,1.,1.,1.,1.,1.,1.,
1.,1.,1.,1.,1.,1.,1.,1.,1.,1.,1.,1.,1.,1.,1.,1.,1.,1.,1.,1.,1.,1.,1.,1.,
1.,1.,1.,1.,1.,1.))
REPRESENTATION_ITEM('')
);
#317=(
BOUNDED_CURVE()
B_SPLINE_CURVE(5,(#46373,#46374,#46375,#46376,#46377,#46378,#46379,#46380,
#46381,#46382,#46383,#46384,#46385,#46386,#46387,#46388,#46389,#46390,#46391,
#46392,#46393,#46394,#46395,#46396,#46397,#46398,#46399,#46400,#46401,#46402,
#46403,#46404,#46405,#46406,#46407,#46408,#46409,#46410,#46411,#46412,#46413,
#46414,#46415,#46416,#46417,#46418,#46419,#46420,#46421,#46422,#46423,#46424,
#46425,#46426,#46427,#46428,#46429,#46430,#46431,#46432,#46433,#46434,#46435,
#46436,#46437,#46438,#46439,#46440,#46441,#46442),.UNSPECIFIED.,.F.,.F.)
B_SPLINE_CURVE_WITH_KNOTS((6,1,1,1,1,1,1,1,1,1,1,1,1,1,1,1,1,1,1,1,1,1,
1,1,1,1,1,1,1,1,1,1,1,1,1,1,1,1,1,1,1,1,1,1,1,1,1,1,1,1,1,1,1,1,1,1,1,1,
1,1,1,1,1,1,1,6),(-1.,-0.984615384615383,-0.969230769230768,-0.953846153846152,
-0.938461538461537,-0.923076923076922,-0.907692307692306,-0.892307692307691,
-0.876923076923076,-0.86153846153846,-0.846153846153845,-0.83076923076923,
-0.815384615384614,-0.799999999999999,-0.784615384615384,-0.769230769230768,
-0.753846153846153,-0.738461538461538,-0.723076923076922,-0.707692307692307,
-0.692307692307692,-0.676923076923076,-0.661538461538461,-0.646153846153846,
-0.63076923076923,-0.615384615384615,-0.6,-0.584615384615384,-0.569230769230769,
-0.553846153846154,-0.538461538461538,-0.523076923076923,-0.507692307692308,
-0.492307692307692,-0.476923076923077,-0.461538461538462,-0.446153846153846,
-0.430769230769231,-0.415384615384615,-0.4,-0.384615384615385,-0.369230769230769,
-0.353846153846154,-0.338461538461538,-0.323076923076923,-0.307692307692308,
-0.292307692307692,-0.276923076923077,-0.261538461538462,-0.246153846153846,
-0.230769230769231,-0.215384615384615,-0.2,-0.184615384615385,-0.169230769230769,
-0.153846153846154,-0.138461538461538,-0.123076923076923,-0.107692307692308,
-0.0923076923076923,-0.0769230769230769,-0.0615384615384615,-0.0461538461538462,
-0.0307692307692308,-0.0153846153846154,0.),.UNSPECIFIED.)
CURVE()
GEOMETRIC_REPRESENTATION_ITEM()
RATIONAL_B_SPLINE_CURVE((1.,1.,1.,1.,1.,1.,1.,1.,1.,1.,1.,1.,1.,1.,1.,1.,
1.,1.,1.,1.,1.,1.,1.,1.,1.,1.,1.,1.,1.,1.,1.,1.,1.,1.,1.,1.,1.,1.,1.,1.,
1.,1.,1.,1.,1.,1.,1.,1.,1.,1.,1.,1.,1.,1.,1.,1.,1.,1.,1.,1.,1.,1.,1.,1.,
1.,1.,1.,1.,1.,1.))
REPRESENTATION_ITEM('')
);
#318=(
BOUNDED_CURVE()
B_SPLINE_CURVE(5,(#46589,#46590,#46591,#46592,#46593,#46594,#46595,#46596,
#46597,#46598,#46599,#46600,#46601,#46602,#46603,#46604,#46605,#46606,#46607,
#46608,#46609,#46610,#46611,#46612,#46613,#46614,#46615,#46616,#46617,#46618,
#46619,#46620,#46621,#46622,#46623,#46624,#46625,#46626,#46627,#46628,#46629,
#46630,#46631,#46632,#46633,#46634,#46635,#46636,#46637,#46638,#46639,#46640,
#46641,#46642,#46643,#46644,#46645,#46646,#46647,#46648,#46649,#46650,#46651,
#46652,#46653,#46654,#46655,#46656,#46657,#46658),.UNSPECIFIED.,.F.,.F.)
B_SPLINE_CURVE_WITH_KNOTS((6,1,1,1,1,1,1,1,1,1,1,1,1,1,1,1,1,1,1,1,1,1,
1,1,1,1,1,1,1,1,1,1,1,1,1,1,1,1,1,1,1,1,1,1,1,1,1,1,1,1,1,1,1,1,1,1,1,1,
1,1,1,1,1,1,1,6),(-1.,-0.984615384615383,-0.969230769230768,-0.953846153846152,
-0.938461538461537,-0.923076923076922,-0.907692307692306,-0.892307692307691,
-0.876923076923076,-0.86153846153846,-0.846153846153845,-0.83076923076923,
-0.815384615384614,-0.799999999999999,-0.784615384615384,-0.769230769230768,
-0.753846153846153,-0.738461538461538,-0.723076923076922,-0.707692307692307,
-0.692307692307692,-0.676923076923076,-0.661538461538461,-0.646153846153846,
-0.63076923076923,-0.615384615384615,-0.6,-0.584615384615384,-0.569230769230769,
-0.553846153846154,-0.538461538461538,-0.523076923076923,-0.507692307692308,
-0.492307692307692,-0.476923076923077,-0.461538461538462,-0.446153846153846,
-0.430769230769231,-0.415384615384615,-0.4,-0.384615384615385,-0.369230769230769,
-0.353846153846154,-0.338461538461538,-0.323076923076923,-0.307692307692308,
-0.292307692307692,-0.276923076923077,-0.261538461538462,-0.246153846153846,
-0.230769230769231,-0.215384615384615,-0.2,-0.184615384615385,-0.169230769230769,
-0.153846153846154,-0.138461538461538,-0.123076923076923,-0.107692307692308,
-0.0923076923076923,-0.0769230769230769,-0.0615384615384615,-0.0461538461538462,
-0.0307692307692308,-0.0153846153846154,0.),.UNSPECIFIED.)
CURVE()
GEOMETRIC_REPRESENTATION_ITEM()
RATIONAL_B_SPLINE_CURVE((1.,1.,1.,1.,1.,1.,1.,1.,1.,1.,1.,1.,1.,1.,1.,1.,
1.,1.,1.,1.,1.,1.,1.,1.,1.,1.,1.,1.,1.,1.,1.,1.,1.,1.,1.,1.,1.,1.,1.,1.,
1.,1.,1.,1.,1.,1.,1.,1.,1.,1.,1.,1.,1.,1.,1.,1.,1.,1.,1.,1.,1.,1.,1.,1.,
1.,1.,1.,1.,1.,1.))
REPRESENTATION_ITEM('')
);
#319=(
BOUNDED_CURVE()
B_SPLINE_CURVE(5,(#46805,#46806,#46807,#46808,#46809,#46810,#46811,#46812,
#46813,#46814,#46815,#46816,#46817,#46818,#46819,#46820,#46821,#46822,#46823,
#46824,#46825,#46826,#46827,#46828,#46829,#46830,#46831,#46832,#46833,#46834,
#46835,#46836,#46837,#46838,#46839,#46840,#46841,#46842,#46843,#46844,#46845,
#46846,#46847,#46848,#46849,#46850,#46851,#46852,#46853,#46854,#46855,#46856,
#46857,#46858,#46859,#46860,#46861,#46862,#46863,#46864,#46865,#46866,#46867,
#46868,#46869,#46870,#46871,#46872,#46873,#46874),.UNSPECIFIED.,.F.,.F.)
B_SPLINE_CURVE_WITH_KNOTS((6,1,1,1,1,1,1,1,1,1,1,1,1,1,1,1,1,1,1,1,1,1,
1,1,1,1,1,1,1,1,1,1,1,1,1,1,1,1,1,1,1,1,1,1,1,1,1,1,1,1,1,1,1,1,1,1,1,1,
1,1,1,1,1,1,1,6),(-1.,-0.984615384615383,-0.969230769230768,-0.953846153846152,
-0.938461538461537,-0.923076923076922,-0.907692307692306,-0.892307692307691,
-0.876923076923076,-0.86153846153846,-0.846153846153845,-0.83076923076923,
-0.815384615384614,-0.799999999999999,-0.784615384615384,-0.769230769230768,
-0.753846153846153,-0.738461538461538,-0.723076923076922,-0.707692307692307,
-0.692307692307692,-0.676923076923076,-0.661538461538461,-0.646153846153846,
-0.63076923076923,-0.615384615384615,-0.6,-0.584615384615384,-0.569230769230769,
-0.553846153846154,-0.538461538461538,-0.523076923076923,-0.507692307692308,
-0.492307692307692,-0.476923076923077,-0.461538461538462,-0.446153846153846,
-0.430769230769231,-0.415384615384615,-0.4,-0.384615384615385,-0.369230769230769,
-0.353846153846154,-0.338461538461538,-0.323076923076923,-0.307692307692308,
-0.292307692307692,-0.276923076923077,-0.261538461538462,-0.246153846153846,
-0.230769230769231,-0.215384615384615,-0.2,-0.184615384615385,-0.169230769230769,
-0.153846153846154,-0.138461538461538,-0.123076923076923,-0.107692307692308,
-0.0923076923076923,-0.0769230769230769,-0.0615384615384615,-0.0461538461538462,
-0.0307692307692308,-0.0153846153846154,0.),.UNSPECIFIED.)
CURVE()
GEOMETRIC_REPRESENTATION_ITEM()
RATIONAL_B_SPLINE_CURVE((1.,1.,1.,1.,1.,1.,1.,1.,1.,1.,1.,1.,1.,1.,1.,1.,
1.,1.,1.,1.,1.,1.,1.,1.,1.,1.,1.,1.,1.,1.,1.,1.,1.,1.,1.,1.,1.,1.,1.,1.,
1.,1.,1.,1.,1.,1.,1.,1.,1.,1.,1.,1.,1.,1.,1.,1.,1.,1.,1.,1.,1.,1.,1.,1.,
1.,1.,1.,1.,1.,1.))
REPRESENTATION_ITEM('')
);
#320=(
BOUNDED_CURVE()
B_SPLINE_CURVE(5,(#47021,#47022,#47023,#47024,#47025,#47026,#47027,#47028,
#47029,#47030,#47031,#47032,#47033,#47034,#47035,#47036,#47037,#47038,#47039,
#47040,#47041,#47042,#47043,#47044,#47045,#47046,#47047,#47048,#47049,#47050,
#47051,#47052,#47053,#47054,#47055,#47056,#47057,#47058,#47059,#47060,#47061,
#47062,#47063,#47064,#47065,#47066,#47067,#47068,#47069,#47070,#47071,#47072,
#47073,#47074,#47075,#47076,#47077,#47078,#47079,#47080,#47081,#47082,#47083,
#47084,#47085,#47086,#47087,#47088,#47089,#47090),.UNSPECIFIED.,.F.,.F.)
B_SPLINE_CURVE_WITH_KNOTS((6,1,1,1,1,1,1,1,1,1,1,1,1,1,1,1,1,1,1,1,1,1,
1,1,1,1,1,1,1,1,1,1,1,1,1,1,1,1,1,1,1,1,1,1,1,1,1,1,1,1,1,1,1,1,1,1,1,1,
1,1,1,1,1,1,1,6),(-1.,-0.984615384615383,-0.969230769230768,-0.953846153846152,
-0.938461538461537,-0.923076923076922,-0.907692307692306,-0.892307692307691,
-0.876923076923076,-0.86153846153846,-0.846153846153845,-0.83076923076923,
-0.815384615384614,-0.799999999999999,-0.784615384615384,-0.769230769230768,
-0.753846153846153,-0.738461538461538,-0.723076923076922,-0.707692307692307,
-0.692307692307692,-0.676923076923076,-0.661538461538461,-0.646153846153846,
-0.63076923076923,-0.615384615384615,-0.6,-0.584615384615384,-0.569230769230769,
-0.553846153846154,-0.538461538461538,-0.523076923076923,-0.507692307692308,
-0.492307692307692,-0.476923076923077,-0.461538461538462,-0.446153846153846,
-0.430769230769231,-0.415384615384615,-0.4,-0.384615384615385,-0.369230769230769,
-0.353846153846154,-0.338461538461538,-0.323076923076923,-0.307692307692308,
-0.292307692307692,-0.276923076923077,-0.261538461538462,-0.246153846153846,
-0.230769230769231,-0.215384615384615,-0.2,-0.184615384615385,-0.169230769230769,
-0.153846153846154,-0.138461538461538,-0.123076923076923,-0.107692307692308,
-0.0923076923076923,-0.0769230769230769,-0.0615384615384615,-0.0461538461538462,
-0.0307692307692308,-0.0153846153846154,0.),.UNSPECIFIED.)
CURVE()
GEOMETRIC_REPRESENTATION_ITEM()
RATIONAL_B_SPLINE_CURVE((1.,1.,1.,1.,1.,1.,1.,1.,1.,1.,1.,1.,1.,1.,1.,1.,
1.,1.,1.,1.,1.,1.,1.,1.,1.,1.,1.,1.,1.,1.,1.,1.,1.,1.,1.,1.,1.,1.,1.,1.,
1.,1.,1.,1.,1.,1.,1.,1.,1.,1.,1.,1.,1.,1.,1.,1.,1.,1.,1.,1.,1.,1.,1.,1.,
1.,1.,1.,1.,1.,1.))
REPRESENTATION_ITEM('')
);
#321=(
BOUNDED_CURVE()
B_SPLINE_CURVE(5,(#47237,#47238,#47239,#47240,#47241,#47242,#47243,#47244,
#47245,#47246,#47247,#47248,#47249,#47250,#47251,#47252,#47253,#47254,#47255,
#47256,#47257,#47258,#47259,#47260,#47261,#47262,#47263,#47264,#47265,#47266,
#47267,#47268,#47269,#47270,#47271,#47272,#47273,#47274,#47275,#47276,#47277,
#47278,#47279,#47280,#47281,#47282,#47283,#47284,#47285,#47286,#47287,#47288,
#47289,#47290,#47291,#47292,#47293,#47294,#47295,#47296,#47297,#47298,#47299,
#47300,#47301,#47302,#47303,#47304,#47305,#47306),.UNSPECIFIED.,.F.,.F.)
B_SPLINE_CURVE_WITH_KNOTS((6,1,1,1,1,1,1,1,1,1,1,1,1,1,1,1,1,1,1,1,1,1,
1,1,1,1,1,1,1,1,1,1,1,1,1,1,1,1,1,1,1,1,1,1,1,1,1,1,1,1,1,1,1,1,1,1,1,1,
1,1,1,1,1,1,1,6),(-1.,-0.984615384615383,-0.969230769230768,-0.953846153846152,
-0.938461538461537,-0.923076923076922,-0.907692307692306,-0.892307692307691,
-0.876923076923076,-0.86153846153846,-0.846153846153845,-0.83076923076923,
-0.815384615384614,-0.799999999999999,-0.784615384615384,-0.769230769230768,
-0.753846153846153,-0.738461538461538,-0.723076923076922,-0.707692307692307,
-0.692307692307692,-0.676923076923076,-0.661538461538461,-0.646153846153846,
-0.63076923076923,-0.615384615384615,-0.6,-0.584615384615384,-0.569230769230769,
-0.553846153846154,-0.538461538461538,-0.523076923076923,-0.507692307692308,
-0.492307692307692,-0.476923076923077,-0.461538461538462,-0.446153846153846,
-0.430769230769231,-0.415384615384615,-0.4,-0.384615384615385,-0.369230769230769,
-0.353846153846154,-0.338461538461538,-0.323076923076923,-0.307692307692308,
-0.292307692307692,-0.276923076923077,-0.261538461538462,-0.246153846153846,
-0.230769230769231,-0.215384615384615,-0.2,-0.184615384615385,-0.169230769230769,
-0.153846153846154,-0.138461538461538,-0.123076923076923,-0.107692307692308,
-0.0923076923076923,-0.0769230769230769,-0.0615384615384615,-0.0461538461538462,
-0.0307692307692308,-0.0153846153846154,0.),.UNSPECIFIED.)
CURVE()
GEOMETRIC_REPRESENTATION_ITEM()
RATIONAL_B_SPLINE_CURVE((1.,1.,1.,1.,1.,1.,1.,1.,1.,1.,1.,1.,1.,1.,1.,1.,
1.,1.,1.,1.,1.,1.,1.,1.,1.,1.,1.,1.,1.,1.,1.,1.,1.,1.,1.,1.,1.,1.,1.,1.,
1.,1.,1.,1.,1.,1.,1.,1.,1.,1.,1.,1.,1.,1.,1.,1.,1.,1.,1.,1.,1.,1.,1.,1.,
1.,1.,1.,1.,1.,1.))
REPRESENTATION_ITEM('')
);
#322=(
BOUNDED_CURVE()
B_SPLINE_CURVE(5,(#47453,#47454,#47455,#47456,#47457,#47458,#47459,#47460,
#47461,#47462,#47463,#47464,#47465,#47466,#47467,#47468,#47469,#47470,#47471,
#47472,#47473,#47474,#47475,#47476,#47477,#47478,#47479,#47480,#47481,#47482,
#47483,#47484,#47485,#47486,#47487,#47488,#47489,#47490,#47491,#47492,#47493,
#47494,#47495,#47496,#47497,#47498,#47499,#47500,#47501,#47502,#47503,#47504,
#47505,#47506,#47507,#47508,#47509,#47510,#47511,#47512,#47513,#47514,#47515,
#47516,#47517,#47518,#47519,#47520,#47521,#47522),.UNSPECIFIED.,.F.,.F.)
B_SPLINE_CURVE_WITH_KNOTS((6,1,1,1,1,1,1,1,1,1,1,1,1,1,1,1,1,1,1,1,1,1,
1,1,1,1,1,1,1,1,1,1,1,1,1,1,1,1,1,1,1,1,1,1,1,1,1,1,1,1,1,1,1,1,1,1,1,1,
1,1,1,1,1,1,1,6),(-1.,-0.984615384615383,-0.969230769230768,-0.953846153846152,
-0.938461538461537,-0.923076923076922,-0.907692307692306,-0.892307692307691,
-0.876923076923076,-0.86153846153846,-0.846153846153845,-0.83076923076923,
-0.815384615384614,-0.799999999999999,-0.784615384615384,-0.769230769230768,
-0.753846153846153,-0.738461538461538,-0.723076923076922,-0.707692307692307,
-0.692307692307692,-0.676923076923076,-0.661538461538461,-0.646153846153846,
-0.63076923076923,-0.615384615384615,-0.6,-0.584615384615384,-0.569230769230769,
-0.553846153846154,-0.538461538461538,-0.523076923076923,-0.507692307692308,
-0.492307692307692,-0.476923076923077,-0.461538461538462,-0.446153846153846,
-0.430769230769231,-0.415384615384615,-0.4,-0.384615384615385,-0.369230769230769,
-0.353846153846154,-0.338461538461538,-0.323076923076923,-0.307692307692308,
-0.292307692307692,-0.276923076923077,-0.261538461538462,-0.246153846153846,
-0.230769230769231,-0.215384615384615,-0.2,-0.184615384615385,-0.169230769230769,
-0.153846153846154,-0.138461538461538,-0.123076923076923,-0.107692307692308,
-0.0923076923076923,-0.0769230769230769,-0.0615384615384615,-0.0461538461538462,
-0.0307692307692308,-0.0153846153846154,0.),.UNSPECIFIED.)
CURVE()
GEOMETRIC_REPRESENTATION_ITEM()
RATIONAL_B_SPLINE_CURVE((1.,1.,1.,1.,1.,1.,1.,1.,1.,1.,1.,1.,1.,1.,1.,1.,
1.,1.,1.,1.,1.,1.,1.,1.,1.,1.,1.,1.,1.,1.,1.,1.,1.,1.,1.,1.,1.,1.,1.,1.,
1.,1.,1.,1.,1.,1.,1.,1.,1.,1.,1.,1.,1.,1.,1.,1.,1.,1.,1.,1.,1.,1.,1.,1.,
1.,1.,1.,1.,1.,1.))
REPRESENTATION_ITEM('')
);
#323=(
BOUNDED_CURVE()
B_SPLINE_CURVE(5,(#47669,#47670,#47671,#47672,#47673,#47674,#47675,#47676,
#47677,#47678,#47679,#47680,#47681,#47682,#47683,#47684,#47685,#47686,#47687,
#47688,#47689,#47690,#47691,#47692,#47693,#47694,#47695,#47696,#47697,#47698,
#47699,#47700,#47701,#47702,#47703,#47704,#47705,#47706,#47707,#47708,#47709,
#47710,#47711,#47712,#47713,#47714,#47715,#47716,#47717,#47718,#47719,#47720,
#47721,#47722,#47723,#47724,#47725,#47726,#47727,#47728,#47729,#47730,#47731,
#47732,#47733,#47734,#47735,#47736,#47737,#47738),.UNSPECIFIED.,.F.,.F.)
B_SPLINE_CURVE_WITH_KNOTS((6,1,1,1,1,1,1,1,1,1,1,1,1,1,1,1,1,1,1,1,1,1,
1,1,1,1,1,1,1,1,1,1,1,1,1,1,1,1,1,1,1,1,1,1,1,1,1,1,1,1,1,1,1,1,1,1,1,1,
1,1,1,1,1,1,1,6),(-1.,-0.984615384615383,-0.969230769230768,-0.953846153846152,
-0.938461538461537,-0.923076923076922,-0.907692307692306,-0.892307692307691,
-0.876923076923076,-0.86153846153846,-0.846153846153845,-0.83076923076923,
-0.815384615384614,-0.799999999999999,-0.784615384615384,-0.769230769230768,
-0.753846153846153,-0.738461538461538,-0.723076923076922,-0.707692307692307,
-0.692307692307692,-0.676923076923076,-0.661538461538461,-0.646153846153846,
-0.63076923076923,-0.615384615384615,-0.6,-0.584615384615384,-0.569230769230769,
-0.553846153846154,-0.538461538461538,-0.523076923076923,-0.507692307692308,
-0.492307692307692,-0.476923076923077,-0.461538461538462,-0.446153846153846,
-0.430769230769231,-0.415384615384615,-0.4,-0.384615384615385,-0.369230769230769,
-0.353846153846154,-0.338461538461538,-0.323076923076923,-0.307692307692308,
-0.292307692307692,-0.276923076923077,-0.261538461538462,-0.246153846153846,
-0.230769230769231,-0.215384615384615,-0.2,-0.184615384615385,-0.169230769230769,
-0.153846153846154,-0.138461538461538,-0.123076923076923,-0.107692307692308,
-0.0923076923076923,-0.0769230769230769,-0.0615384615384615,-0.0461538461538462,
-0.0307692307692308,-0.0153846153846154,0.),.UNSPECIFIED.)
CURVE()
GEOMETRIC_REPRESENTATION_ITEM()
RATIONAL_B_SPLINE_CURVE((1.,1.,1.,1.,1.,1.,1.,1.,1.,1.,1.,1.,1.,1.,1.,1.,
1.,1.,1.,1.,1.,1.,1.,1.,1.,1.,1.,1.,1.,1.,1.,1.,1.,1.,1.,1.,1.,1.,1.,1.,
1.,1.,1.,1.,1.,1.,1.,1.,1.,1.,1.,1.,1.,1.,1.,1.,1.,1.,1.,1.,1.,1.,1.,1.,
1.,1.,1.,1.,1.,1.))
REPRESENTATION_ITEM('')
);
#324=(
BOUNDED_CURVE()
B_SPLINE_CURVE(5,(#47885,#47886,#47887,#47888,#47889,#47890,#47891,#47892,
#47893,#47894,#47895,#47896,#47897,#47898,#47899,#47900,#47901,#47902,#47903,
#47904,#47905,#47906,#47907,#47908,#47909,#47910,#47911,#47912,#47913,#47914,
#47915,#47916,#47917,#47918,#47919,#47920,#47921,#47922,#47923,#47924,#47925,
#47926,#47927,#47928,#47929,#47930,#47931,#47932,#47933,#47934,#47935,#47936,
#47937,#47938,#47939,#47940,#47941,#47942,#47943,#47944,#47945,#47946,#47947,
#47948,#47949,#47950,#47951,#47952,#47953,#47954),.UNSPECIFIED.,.F.,.F.)
B_SPLINE_CURVE_WITH_KNOTS((6,1,1,1,1,1,1,1,1,1,1,1,1,1,1,1,1,1,1,1,1,1,
1,1,1,1,1,1,1,1,1,1,1,1,1,1,1,1,1,1,1,1,1,1,1,1,1,1,1,1,1,1,1,1,1,1,1,1,
1,1,1,1,1,1,1,6),(-1.,-0.984615384615383,-0.969230769230768,-0.953846153846152,
-0.938461538461537,-0.923076923076922,-0.907692307692306,-0.892307692307691,
-0.876923076923076,-0.86153846153846,-0.846153846153845,-0.83076923076923,
-0.815384615384614,-0.799999999999999,-0.784615384615384,-0.769230769230768,
-0.753846153846153,-0.738461538461538,-0.723076923076922,-0.707692307692307,
-0.692307692307692,-0.676923076923076,-0.661538461538461,-0.646153846153846,
-0.63076923076923,-0.615384615384615,-0.6,-0.584615384615384,-0.569230769230769,
-0.553846153846154,-0.538461538461538,-0.523076923076923,-0.507692307692308,
-0.492307692307692,-0.476923076923077,-0.461538461538462,-0.446153846153846,
-0.430769230769231,-0.415384615384615,-0.4,-0.384615384615385,-0.369230769230769,
-0.353846153846154,-0.338461538461538,-0.323076923076923,-0.307692307692308,
-0.292307692307692,-0.276923076923077,-0.261538461538462,-0.246153846153846,
-0.230769230769231,-0.215384615384615,-0.2,-0.184615384615385,-0.169230769230769,
-0.153846153846154,-0.138461538461538,-0.123076923076923,-0.107692307692308,
-0.0923076923076923,-0.0769230769230769,-0.0615384615384615,-0.0461538461538462,
-0.0307692307692308,-0.0153846153846154,0.),.UNSPECIFIED.)
CURVE()
GEOMETRIC_REPRESENTATION_ITEM()
RATIONAL_B_SPLINE_CURVE((1.,1.,1.,1.,1.,1.,1.,1.,1.,1.,1.,1.,1.,1.,1.,1.,
1.,1.,1.,1.,1.,1.,1.,1.,1.,1.,1.,1.,1.,1.,1.,1.,1.,1.,1.,1.,1.,1.,1.,1.,
1.,1.,1.,1.,1.,1.,1.,1.,1.,1.,1.,1.,1.,1.,1.,1.,1.,1.,1.,1.,1.,1.,1.,1.,
1.,1.,1.,1.,1.,1.))
REPRESENTATION_ITEM('')
);
#325=(
BOUNDED_CURVE()
B_SPLINE_CURVE(5,(#48101,#48102,#48103,#48104,#48105,#48106,#48107,#48108,
#48109,#48110,#48111,#48112,#48113,#48114,#48115,#48116,#48117,#48118,#48119,
#48120,#48121,#48122,#48123,#48124,#48125,#48126,#48127,#48128,#48129,#48130,
#48131,#48132,#48133,#48134,#48135,#48136,#48137,#48138,#48139,#48140,#48141,
#48142,#48143,#48144,#48145,#48146,#48147,#48148,#48149,#48150,#48151,#48152,
#48153,#48154,#48155,#48156,#48157,#48158,#48159,#48160,#48161,#48162,#48163,
#48164,#48165,#48166,#48167,#48168,#48169,#48170),.UNSPECIFIED.,.F.,.F.)
B_SPLINE_CURVE_WITH_KNOTS((6,1,1,1,1,1,1,1,1,1,1,1,1,1,1,1,1,1,1,1,1,1,
1,1,1,1,1,1,1,1,1,1,1,1,1,1,1,1,1,1,1,1,1,1,1,1,1,1,1,1,1,1,1,1,1,1,1,1,
1,1,1,1,1,1,1,6),(-1.,-0.984615384615383,-0.969230769230768,-0.953846153846152,
-0.938461538461537,-0.923076923076922,-0.907692307692306,-0.892307692307691,
-0.876923076923076,-0.86153846153846,-0.846153846153845,-0.83076923076923,
-0.815384615384614,-0.799999999999999,-0.784615384615384,-0.769230769230768,
-0.753846153846153,-0.738461538461538,-0.723076923076922,-0.707692307692307,
-0.692307692307692,-0.676923076923076,-0.661538461538461,-0.646153846153846,
-0.63076923076923,-0.615384615384615,-0.6,-0.584615384615384,-0.569230769230769,
-0.553846153846154,-0.538461538461538,-0.523076923076923,-0.507692307692308,
-0.492307692307692,-0.476923076923077,-0.461538461538462,-0.446153846153846,
-0.430769230769231,-0.415384615384615,-0.4,-0.384615384615385,-0.369230769230769,
-0.353846153846154,-0.338461538461538,-0.323076923076923,-0.307692307692308,
-0.292307692307692,-0.276923076923077,-0.261538461538462,-0.246153846153846,
-0.230769230769231,-0.215384615384615,-0.2,-0.184615384615385,-0.169230769230769,
-0.153846153846154,-0.138461538461538,-0.123076923076923,-0.107692307692308,
-0.0923076923076923,-0.0769230769230769,-0.0615384615384615,-0.0461538461538462,
-0.0307692307692308,-0.0153846153846154,0.),.UNSPECIFIED.)
CURVE()
GEOMETRIC_REPRESENTATION_ITEM()
RATIONAL_B_SPLINE_CURVE((1.,1.,1.,1.,1.,1.,1.,1.,1.,1.,1.,1.,1.,1.,1.,1.,
1.,1.,1.,1.,1.,1.,1.,1.,1.,1.,1.,1.,1.,1.,1.,1.,1.,1.,1.,1.,1.,1.,1.,1.,
1.,1.,1.,1.,1.,1.,1.,1.,1.,1.,1.,1.,1.,1.,1.,1.,1.,1.,1.,1.,1.,1.,1.,1.,
1.,1.,1.,1.,1.,1.))
REPRESENTATION_ITEM('')
);
#326=(
BOUNDED_CURVE()
B_SPLINE_CURVE(5,(#48317,#48318,#48319,#48320,#48321,#48322,#48323,#48324,
#48325,#48326,#48327,#48328,#48329,#48330,#48331,#48332,#48333,#48334,#48335,
#48336,#48337,#48338,#48339,#48340,#48341,#48342,#48343,#48344,#48345,#48346,
#48347,#48348,#48349,#48350,#48351,#48352,#48353,#48354,#48355,#48356,#48357,
#48358,#48359,#48360,#48361,#48362,#48363,#48364,#48365,#48366,#48367,#48368,
#48369,#48370,#48371,#48372,#48373,#48374,#48375,#48376,#48377,#48378,#48379,
#48380,#48381,#48382,#48383,#48384,#48385,#48386),.UNSPECIFIED.,.F.,.F.)
B_SPLINE_CURVE_WITH_KNOTS((6,1,1,1,1,1,1,1,1,1,1,1,1,1,1,1,1,1,1,1,1,1,
1,1,1,1,1,1,1,1,1,1,1,1,1,1,1,1,1,1,1,1,1,1,1,1,1,1,1,1,1,1,1,1,1,1,1,1,
1,1,1,1,1,1,1,6),(-1.,-0.984615384615383,-0.969230769230768,-0.953846153846152,
-0.938461538461537,-0.923076923076922,-0.907692307692306,-0.892307692307691,
-0.876923076923076,-0.86153846153846,-0.846153846153845,-0.83076923076923,
-0.815384615384614,-0.799999999999999,-0.784615384615384,-0.769230769230768,
-0.753846153846153,-0.738461538461538,-0.723076923076922,-0.707692307692307,
-0.692307692307692,-0.676923076923076,-0.661538461538461,-0.646153846153846,
-0.63076923076923,-0.615384615384615,-0.6,-0.584615384615384,-0.569230769230769,
-0.553846153846154,-0.538461538461538,-0.523076923076923,-0.507692307692308,
-0.492307692307692,-0.476923076923077,-0.461538461538462,-0.446153846153846,
-0.430769230769231,-0.415384615384615,-0.4,-0.384615384615385,-0.369230769230769,
-0.353846153846154,-0.338461538461538,-0.323076923076923,-0.307692307692308,
-0.292307692307692,-0.276923076923077,-0.261538461538462,-0.246153846153846,
-0.230769230769231,-0.215384615384615,-0.2,-0.184615384615385,-0.169230769230769,
-0.153846153846154,-0.138461538461538,-0.123076923076923,-0.107692307692308,
-0.0923076923076923,-0.0769230769230769,-0.0615384615384615,-0.0461538461538462,
-0.0307692307692308,-0.0153846153846154,0.),.UNSPECIFIED.)
CURVE()
GEOMETRIC_REPRESENTATION_ITEM()
RATIONAL_B_SPLINE_CURVE((1.,1.,1.,1.,1.,1.,1.,1.,1.,1.,1.,1.,1.,1.,1.,1.,
1.,1.,1.,1.,1.,1.,1.,1.,1.,1.,1.,1.,1.,1.,1.,1.,1.,1.,1.,1.,1.,1.,1.,1.,
1.,1.,1.,1.,1.,1.,1.,1.,1.,1.,1.,1.,1.,1.,1.,1.,1.,1.,1.,1.,1.,1.,1.,1.,
1.,1.,1.,1.,1.,1.))
REPRESENTATION_ITEM('')
);
#327=(
BOUNDED_CURVE()
B_SPLINE_CURVE(5,(#48533,#48534,#48535,#48536,#48537,#48538,#48539,#48540,
#48541,#48542,#48543,#48544,#48545,#48546,#48547,#48548,#48549,#48550,#48551,
#48552,#48553,#48554,#48555,#48556,#48557,#48558,#48559,#48560,#48561,#48562,
#48563,#48564,#48565,#48566,#48567,#48568,#48569,#48570,#48571,#48572,#48573,
#48574,#48575,#48576,#48577,#48578,#48579,#48580,#48581,#48582,#48583,#48584,
#48585,#48586,#48587,#48588,#48589,#48590,#48591,#48592,#48593,#48594,#48595,
#48596,#48597,#48598,#48599,#48600,#48601,#48602),.UNSPECIFIED.,.F.,.F.)
B_SPLINE_CURVE_WITH_KNOTS((6,1,1,1,1,1,1,1,1,1,1,1,1,1,1,1,1,1,1,1,1,1,
1,1,1,1,1,1,1,1,1,1,1,1,1,1,1,1,1,1,1,1,1,1,1,1,1,1,1,1,1,1,1,1,1,1,1,1,
1,1,1,1,1,1,1,6),(-1.,-0.984615384615383,-0.969230769230768,-0.953846153846152,
-0.938461538461537,-0.923076923076922,-0.907692307692306,-0.892307692307691,
-0.876923076923076,-0.86153846153846,-0.846153846153845,-0.83076923076923,
-0.815384615384614,-0.799999999999999,-0.784615384615384,-0.769230769230768,
-0.753846153846153,-0.738461538461538,-0.723076923076922,-0.707692307692307,
-0.692307692307692,-0.676923076923076,-0.661538461538461,-0.646153846153846,
-0.63076923076923,-0.615384615384615,-0.6,-0.584615384615384,-0.569230769230769,
-0.553846153846154,-0.538461538461538,-0.523076923076923,-0.507692307692308,
-0.492307692307692,-0.476923076923077,-0.461538461538462,-0.446153846153846,
-0.430769230769231,-0.415384615384615,-0.4,-0.384615384615385,-0.369230769230769,
-0.353846153846154,-0.338461538461538,-0.323076923076923,-0.307692307692308,
-0.292307692307692,-0.276923076923077,-0.261538461538462,-0.246153846153846,
-0.230769230769231,-0.215384615384615,-0.2,-0.184615384615385,-0.169230769230769,
-0.153846153846154,-0.138461538461538,-0.123076923076923,-0.107692307692308,
-0.0923076923076923,-0.0769230769230769,-0.0615384615384615,-0.0461538461538462,
-0.0307692307692308,-0.0153846153846154,0.),.UNSPECIFIED.)
CURVE()
GEOMETRIC_REPRESENTATION_ITEM()
RATIONAL_B_SPLINE_CURVE((1.,1.,1.,1.,1.,1.,1.,1.,1.,1.,1.,1.,1.,1.,1.,1.,
1.,1.,1.,1.,1.,1.,1.,1.,1.,1.,1.,1.,1.,1.,1.,1.,1.,1.,1.,1.,1.,1.,1.,1.,
1.,1.,1.,1.,1.,1.,1.,1.,1.,1.,1.,1.,1.,1.,1.,1.,1.,1.,1.,1.,1.,1.,1.,1.,
1.,1.,1.,1.,1.,1.))
REPRESENTATION_ITEM('')
);
#328=(
BOUNDED_CURVE()
B_SPLINE_CURVE(5,(#48749,#48750,#48751,#48752,#48753,#48754,#48755,#48756,
#48757,#48758,#48759,#48760,#48761,#48762,#48763,#48764,#48765,#48766,#48767,
#48768,#48769,#48770,#48771,#48772,#48773,#48774,#48775,#48776,#48777,#48778,
#48779,#48780,#48781,#48782,#48783,#48784,#48785,#48786,#48787,#48788,#48789,
#48790,#48791,#48792,#48793,#48794,#48795,#48796,#48797,#48798,#48799,#48800,
#48801,#48802,#48803,#48804,#48805,#48806,#48807,#48808,#48809,#48810,#48811,
#48812,#48813,#48814,#48815,#48816,#48817,#48818),.UNSPECIFIED.,.F.,.F.)
B_SPLINE_CURVE_WITH_KNOTS((6,1,1,1,1,1,1,1,1,1,1,1,1,1,1,1,1,1,1,1,1,1,
1,1,1,1,1,1,1,1,1,1,1,1,1,1,1,1,1,1,1,1,1,1,1,1,1,1,1,1,1,1,1,1,1,1,1,1,
1,1,1,1,1,1,1,6),(-1.,-0.984615384615383,-0.969230769230768,-0.953846153846152,
-0.938461538461537,-0.923076923076922,-0.907692307692306,-0.892307692307691,
-0.876923076923076,-0.86153846153846,-0.846153846153845,-0.83076923076923,
-0.815384615384614,-0.799999999999999,-0.784615384615384,-0.769230769230768,
-0.753846153846153,-0.738461538461538,-0.723076923076922,-0.707692307692307,
-0.692307692307692,-0.676923076923076,-0.661538461538461,-0.646153846153846,
-0.63076923076923,-0.615384615384615,-0.6,-0.584615384615384,-0.569230769230769,
-0.553846153846154,-0.538461538461538,-0.523076923076923,-0.507692307692308,
-0.492307692307692,-0.476923076923077,-0.461538461538462,-0.446153846153846,
-0.430769230769231,-0.415384615384615,-0.4,-0.384615384615385,-0.369230769230769,
-0.353846153846154,-0.338461538461538,-0.323076923076923,-0.307692307692308,
-0.292307692307692,-0.276923076923077,-0.261538461538462,-0.246153846153846,
-0.230769230769231,-0.215384615384615,-0.2,-0.184615384615385,-0.169230769230769,
-0.153846153846154,-0.138461538461538,-0.123076923076923,-0.107692307692308,
-0.0923076923076923,-0.0769230769230769,-0.0615384615384615,-0.0461538461538462,
-0.0307692307692308,-0.0153846153846154,0.),.UNSPECIFIED.)
CURVE()
GEOMETRIC_REPRESENTATION_ITEM()
RATIONAL_B_SPLINE_CURVE((1.,1.,1.,1.,1.,1.,1.,1.,1.,1.,1.,1.,1.,1.,1.,1.,
1.,1.,1.,1.,1.,1.,1.,1.,1.,1.,1.,1.,1.,1.,1.,1.,1.,1.,1.,1.,1.,1.,1.,1.,
1.,1.,1.,1.,1.,1.,1.,1.,1.,1.,1.,1.,1.,1.,1.,1.,1.,1.,1.,1.,1.,1.,1.,1.,
1.,1.,1.,1.,1.,1.))
REPRESENTATION_ITEM('')
);
#329=(
BOUNDED_CURVE()
B_SPLINE_CURVE(5,(#48965,#48966,#48967,#48968,#48969,#48970,#48971,#48972,
#48973,#48974,#48975,#48976,#48977,#48978,#48979,#48980,#48981,#48982,#48983,
#48984,#48985,#48986,#48987,#48988,#48989,#48990,#48991,#48992,#48993,#48994,
#48995,#48996,#48997,#48998,#48999,#49000,#49001,#49002,#49003,#49004,#49005,
#49006,#49007,#49008,#49009,#49010,#49011,#49012,#49013,#49014,#49015,#49016,
#49017,#49018,#49019,#49020,#49021,#49022,#49023,#49024,#49025,#49026,#49027,
#49028,#49029,#49030,#49031,#49032,#49033,#49034),.UNSPECIFIED.,.F.,.F.)
B_SPLINE_CURVE_WITH_KNOTS((6,1,1,1,1,1,1,1,1,1,1,1,1,1,1,1,1,1,1,1,1,1,
1,1,1,1,1,1,1,1,1,1,1,1,1,1,1,1,1,1,1,1,1,1,1,1,1,1,1,1,1,1,1,1,1,1,1,1,
1,1,1,1,1,1,1,6),(-1.,-0.984615384615383,-0.969230769230768,-0.953846153846152,
-0.938461538461537,-0.923076923076922,-0.907692307692306,-0.892307692307691,
-0.876923076923076,-0.86153846153846,-0.846153846153845,-0.83076923076923,
-0.815384615384614,-0.799999999999999,-0.784615384615384,-0.769230769230768,
-0.753846153846153,-0.738461538461538,-0.723076923076922,-0.707692307692307,
-0.692307692307692,-0.676923076923076,-0.661538461538461,-0.646153846153846,
-0.63076923076923,-0.615384615384615,-0.6,-0.584615384615384,-0.569230769230769,
-0.553846153846154,-0.538461538461538,-0.523076923076923,-0.507692307692308,
-0.492307692307692,-0.476923076923077,-0.461538461538462,-0.446153846153846,
-0.430769230769231,-0.415384615384615,-0.4,-0.384615384615385,-0.369230769230769,
-0.353846153846154,-0.338461538461538,-0.323076923076923,-0.307692307692308,
-0.292307692307692,-0.276923076923077,-0.261538461538462,-0.246153846153846,
-0.230769230769231,-0.215384615384615,-0.2,-0.184615384615385,-0.169230769230769,
-0.153846153846154,-0.138461538461538,-0.123076923076923,-0.107692307692308,
-0.0923076923076923,-0.0769230769230769,-0.0615384615384615,-0.0461538461538462,
-0.0307692307692308,-0.0153846153846154,0.),.UNSPECIFIED.)
CURVE()
GEOMETRIC_REPRESENTATION_ITEM()
RATIONAL_B_SPLINE_CURVE((1.,1.,1.,1.,1.,1.,1.,1.,1.,1.,1.,1.,1.,1.,1.,1.,
1.,1.,1.,1.,1.,1.,1.,1.,1.,1.,1.,1.,1.,1.,1.,1.,1.,1.,1.,1.,1.,1.,1.,1.,
1.,1.,1.,1.,1.,1.,1.,1.,1.,1.,1.,1.,1.,1.,1.,1.,1.,1.,1.,1.,1.,1.,1.,1.,
1.,1.,1.,1.,1.,1.))
REPRESENTATION_ITEM('')
);
#330=(
BOUNDED_CURVE()
B_SPLINE_CURVE(5,(#49181,#49182,#49183,#49184,#49185,#49186,#49187,#49188,
#49189,#49190,#49191,#49192,#49193,#49194,#49195,#49196,#49197,#49198,#49199,
#49200,#49201,#49202,#49203,#49204,#49205,#49206,#49207,#49208,#49209,#49210,
#49211,#49212,#49213,#49214,#49215,#49216,#49217,#49218,#49219,#49220,#49221,
#49222,#49223,#49224,#49225,#49226,#49227,#49228,#49229,#49230,#49231,#49232,
#49233,#49234,#49235,#49236,#49237,#49238,#49239,#49240,#49241,#49242,#49243,
#49244,#49245,#49246,#49247,#49248,#49249,#49250),.UNSPECIFIED.,.F.,.F.)
B_SPLINE_CURVE_WITH_KNOTS((6,1,1,1,1,1,1,1,1,1,1,1,1,1,1,1,1,1,1,1,1,1,
1,1,1,1,1,1,1,1,1,1,1,1,1,1,1,1,1,1,1,1,1,1,1,1,1,1,1,1,1,1,1,1,1,1,1,1,
1,1,1,1,1,1,1,6),(-1.,-0.984615384615383,-0.969230769230768,-0.953846153846152,
-0.938461538461537,-0.923076923076922,-0.907692307692306,-0.892307692307691,
-0.876923076923076,-0.86153846153846,-0.846153846153845,-0.83076923076923,
-0.815384615384614,-0.799999999999999,-0.784615384615384,-0.769230769230768,
-0.753846153846153,-0.738461538461538,-0.723076923076922,-0.707692307692307,
-0.692307692307692,-0.676923076923076,-0.661538461538461,-0.646153846153846,
-0.63076923076923,-0.615384615384615,-0.6,-0.584615384615384,-0.569230769230769,
-0.553846153846154,-0.538461538461538,-0.523076923076923,-0.507692307692308,
-0.492307692307692,-0.476923076923077,-0.461538461538462,-0.446153846153846,
-0.430769230769231,-0.415384615384615,-0.4,-0.384615384615385,-0.369230769230769,
-0.353846153846154,-0.338461538461538,-0.323076923076923,-0.307692307692308,
-0.292307692307692,-0.276923076923077,-0.261538461538462,-0.246153846153846,
-0.230769230769231,-0.215384615384615,-0.2,-0.184615384615385,-0.169230769230769,
-0.153846153846154,-0.138461538461538,-0.123076923076923,-0.107692307692308,
-0.0923076923076923,-0.0769230769230769,-0.0615384615384615,-0.0461538461538462,
-0.0307692307692308,-0.0153846153846154,0.),.UNSPECIFIED.)
CURVE()
GEOMETRIC_REPRESENTATION_ITEM()
RATIONAL_B_SPLINE_CURVE((1.,1.,1.,1.,1.,1.,1.,1.,1.,1.,1.,1.,1.,1.,1.,1.,
1.,1.,1.,1.,1.,1.,1.,1.,1.,1.,1.,1.,1.,1.,1.,1.,1.,1.,1.,1.,1.,1.,1.,1.,
1.,1.,1.,1.,1.,1.,1.,1.,1.,1.,1.,1.,1.,1.,1.,1.,1.,1.,1.,1.,1.,1.,1.,1.,
1.,1.,1.,1.,1.,1.))
REPRESENTATION_ITEM('')
);
#1167=SHAPE_REPRESENTATION_RELATIONSHIP('SRR','None',#73658,#1223);
#1223=ADVANCED_BREP_SHAPE_REPRESENTATION('',(#1363),#73354);
#1294=STYLED_ITEM('',(#73974),#1363);
#1363=MANIFOLD_SOLID_BREP('Body1',#16184);
#1578=FACE_BOUND('',#3720,.T.);
#1579=FACE_BOUND('',#3723,.T.);
#1580=FACE_BOUND('',#3805,.T.);
#1888=PLANE('',#18045);
#1889=PLANE('',#18046);
#1890=PLANE('',#18047);
#1891=PLANE('',#18048);
#1892=PLANE('',#18053);
#1893=PLANE('',#18076);
#1894=PLANE('',#18079);
#1895=PLANE('',#18082);
#1896=PLANE('',#18085);
#1897=PLANE('',#18088);
#1898=PLANE('',#18091);
#1899=PLANE('',#18094);
#1900=PLANE('',#18097);
#1901=PLANE('',#18100);
#1902=PLANE('',#18103);
#1903=PLANE('',#18106);
#1904=PLANE('',#18109);
#1905=PLANE('',#18112);
#1906=PLANE('',#18115);
#1907=PLANE('',#18118);
#1908=PLANE('',#18121);
#1909=PLANE('',#18124);
#1910=PLANE('',#18127);
#1911=PLANE('',#18130);
#1912=PLANE('',#18133);
#1913=PLANE('',#18134);
#2599=FACE_OUTER_BOUND('',#3716,.T.);
#2600=FACE_OUTER_BOUND('',#3717,.T.);
#2601=FACE_OUTER_BOUND('',#3718,.T.);
#2602=FACE_OUTER_BOUND('',#3719,.T.);
#2603=FACE_OUTER_BOUND('',#3721,.T.);
#2604=FACE_OUTER_BOUND('',#3722,.T.);
#2605=FACE_OUTER_BOUND('',#3724,.T.);
#2606=FACE_OUTER_BOUND('',#3725,.T.);
#2607=FACE_OUTER_BOUND('',#3726,.T.);
#2608=FACE_OUTER_BOUND('',#3727,.T.);
#2609=FACE_OUTER_BOUND('',#3728,.T.);
#2610=FACE_OUTER_BOUND('',#3729,.T.);
#2611=FACE_OUTER_BOUND('',#3730,.T.);
#2612=FACE_OUTER_BOUND('',#3731,.T.);
#2613=FACE_OUTER_BOUND('',#3732,.T.);
#2614=FACE_OUTER_BOUND('',#3733,.T.);
#2615=FACE_OUTER_BOUND('',#3734,.T.);
#2616=FACE_OUTER_BOUND('',#3735,.T.);
#2617=FACE_OUTER_BOUND('',#3736,.T.);
#2618=FACE_OUTER_BOUND('',#3737,.T.);
#2619=FACE_OUTER_BOUND('',#3738,.T.);
#2620=FACE_OUTER_BOUND('',#3739,.T.);
#2621=FACE_OUTER_BOUND('',#3740,.T.);
#2622=FACE_OUTER_BOUND('',#3741,.T.);
#2623=FACE_OUTER_BOUND('',#3742,.T.);
#2624=FACE_OUTER_BOUND('',#3743,.T.);
#2625=FACE_OUTER_BOUND('',#3744,.T.);
#2626=FACE_OUTER_BOUND('',#3745,.T.);
#2627=FACE_OUTER_BOUND('',#3746,.T.);
#2628=FACE_OUTER_BOUND('',#3747,.T.);
#2629=FACE_OUTER_BOUND('',#3748,.T.);
#2630=FACE_OUTER_BOUND('',#3749,.T.);
#2631=FACE_OUTER_BOUND('',#3750,.T.);
#2632=FACE_OUTER_BOUND('',#3751,.T.);
#2633=FACE_OUTER_BOUND('',#3752,.T.);
#2634=FACE_OUTER_BOUND('',#3753,.T.);
#2635=FACE_OUTER_BOUND('',#3754,.T.);
#2636=FACE_OUTER_BOUND('',#3755,.T.);
#2637=FACE_OUTER_BOUND('',#3756,.T.);
#2638=FACE_OUTER_BOUND('',#3757,.T.);
#2639=FACE_OUTER_BOUND('',#3758,.T.);
#2640=FACE_OUTER_BOUND('',#3759,.T.);
#2641=FACE_OUTER_BOUND('',#3760,.T.);
#2642=FACE_OUTER_BOUND('',#3761,.T.);
#2643=FACE_OUTER_BOUND('',#3762,.T.);
#2644=FACE_OUTER_BOUND('',#3763,.T.);
#2645=FACE_OUTER_BOUND('',#3764,.T.);
#2646=FACE_OUTER_BOUND('',#3765,.T.);
#2647=FACE_OUTER_BOUND('',#3766,.T.);
#2648=FACE_OUTER_BOUND('',#3767,.T.);
#2649=FACE_OUTER_BOUND('',#3768,.T.);
#2650=FACE_OUTER_BOUND('',#3769,.T.);
#2651=FACE_OUTER_BOUND('',#3770,.T.);
#2652=FACE_OUTER_BOUND('',#3771,.T.);
#2653=FACE_OUTER_BOUND('',#3772,.T.);
#2654=FACE_OUTER_BOUND('',#3773,.T.);
#2655=FACE_OUTER_BOUND('',#3774,.T.);
#2656=FACE_OUTER_BOUND('',#3775,.T.);
#2657=FACE_OUTER_BOUND('',#3776,.T.);
#2658=FACE_OUTER_BOUND('',#3777,.T.);
#2659=FACE_OUTER_BOUND('',#3778,.T.);
#2660=FACE_OUTER_BOUND('',#3779,.T.);
#2661=FACE_OUTER_BOUND('',#3780,.T.);
#2662=FACE_OUTER_BOUND('',#3781,.T.);
#2663=FACE_OUTER_BOUND('',#3782,.T.);
#2664=FACE_OUTER_BOUND('',#3783,.T.);
#2665=FACE_OUTER_BOUND('',#3784,.T.);
#2666=FACE_OUTER_BOUND('',#3785,.T.);
#2667=FACE_OUTER_BOUND('',#3786,.T.);
#2668=FACE_OUTER_BOUND('',#3787,.T.);
#2669=FACE_OUTER_BOUND('',#3788,.T.);
#2670=FACE_OUTER_BOUND('',#3789,.T.);
#2671=FACE_OUTER_BOUND('',#3790,.T.);
#2672=FACE_OUTER_BOUND('',#3791,.T.);
#2673=FACE_OUTER_BOUND('',#3792,.T.);
#2674=FACE_OUTER_BOUND('',#3793,.T.);
#2675=FACE_OUTER_BOUND('',#3794,.T.);
#2676=FACE_OUTER_BOUND('',#3795,.T.);
#2677=FACE_OUTER_BOUND('',#3796,.T.);
#2678=FACE_OUTER_BOUND('',#3797,.T.);
#2679=FACE_OUTER_BOUND('',#3798,.T.);
#2680=FACE_OUTER_BOUND('',#3799,.T.);
#2681=FACE_OUTER_BOUND('',#3800,.T.);
#2682=FACE_OUTER_BOUND('',#3801,.T.);
#2683=FACE_OUTER_BOUND('',#3802,.T.);
#2684=FACE_OUTER_BOUND('',#3803,.T.);
#2685=FACE_OUTER_BOUND('',#3804,.T.);
#2686=FACE_OUTER_BOUND('',#3806,.T.);
#3716=EDGE_LOOP('',(#13167,#13168,#13169,#13170));
#3717=EDGE_LOOP('',(#13171,#13172,#13173,#13174));
#3718=EDGE_LOOP('',(#13175,#13176,#13177,#13178));
#3719=EDGE_LOOP('',(#13179));
#3720=EDGE_LOOP('',(#13180,#13181,#13182,#13183));
#3721=EDGE_LOOP('',(#13184,#13185,#13186,#13187));
#3722=EDGE_LOOP('',(#13188,#13189,#13190,#13191,#13192,#13193,#13194,#13195,
#13196,#13197,#13198,#13199,#13200,#13201,#13202,#13203,#13204,#13205,#13206,
#13207,#13208,#13209,#13210,#13211,#13212,#13213,#13214,#13215,#13216,#13217,
#13218,#13219,#13220,#13221,#13222,#13223,#13224,#13225,#13226,#13227,#13228,
#13229,#13230,#13231,#13232,#13233,#13234,#13235,#13236,#13237,#13238,#13239,
#13240,#13241,#13242,#13243,#13244,#13245,#13246,#13247,#13248,#13249,#13250,
#13251,#13252,#13253,#13254,#13255,#13256,#13257,#13258,#13259,#13260,#13261,
#13262,#13263,#13264,#13265,#13266,#13267));
#3723=EDGE_LOOP('',(#13268,#13269,#13270,#13271));
#3724=EDGE_LOOP('',(#13272,#13273,#13274,#13275));
#3725=EDGE_LOOP('',(#13276,#13277,#13278,#13279));
#3726=EDGE_LOOP('',(#13280,#13281,#13282,#13283));
#3727=EDGE_LOOP('',(#13284,#13285,#13286,#13287));
#3728=EDGE_LOOP('',(#13288,#13289,#13290,#13291));
#3729=EDGE_LOOP('',(#13292,#13293,#13294,#13295));
#3730=EDGE_LOOP('',(#13296,#13297,#13298,#13299));
#3731=EDGE_LOOP('',(#13300,#13301,#13302,#13303));
#3732=EDGE_LOOP('',(#13304,#13305,#13306,#13307));
#3733=EDGE_LOOP('',(#13308,#13309,#13310,#13311));
#3734=EDGE_LOOP('',(#13312,#13313,#13314,#13315));
#3735=EDGE_LOOP('',(#13316,#13317,#13318,#13319));
#3736=EDGE_LOOP('',(#13320,#13321,#13322,#13323));
#3737=EDGE_LOOP('',(#13324,#13325,#13326,#13327));
#3738=EDGE_LOOP('',(#13328,#13329,#13330,#13331));
#3739=EDGE_LOOP('',(#13332,#13333,#13334,#13335));
#3740=EDGE_LOOP('',(#13336,#13337,#13338,#13339));
#3741=EDGE_LOOP('',(#13340,#13341,#13342,#13343));
#3742=EDGE_LOOP('',(#13344,#13345,#13346,#13347));
#3743=EDGE_LOOP('',(#13348,#13349,#13350,#13351));
#3744=EDGE_LOOP('',(#13352,#13353,#13354,#13355));
#3745=EDGE_LOOP('',(#13356,#13357,#13358,#13359));
#3746=EDGE_LOOP('',(#13360,#13361,#13362,#13363));
#3747=EDGE_LOOP('',(#13364,#13365,#13366,#13367));
#3748=EDGE_LOOP('',(#13368,#13369,#13370,#13371));
#3749=EDGE_LOOP('',(#13372,#13373,#13374,#13375));
#3750=EDGE_LOOP('',(#13376,#13377,#13378,#13379));
#3751=EDGE_LOOP('',(#13380,#13381,#13382,#13383));
#3752=EDGE_LOOP('',(#13384,#13385,#13386,#13387));
#3753=EDGE_LOOP('',(#13388,#13389,#13390,#13391));
#3754=EDGE_LOOP('',(#13392,#13393,#13394,#13395));
#3755=EDGE_LOOP('',(#13396,#13397,#13398,#13399));
#3756=EDGE_LOOP('',(#13400,#13401,#13402,#13403));
#3757=EDGE_LOOP('',(#13404,#13405,#13406,#13407));
#3758=EDGE_LOOP('',(#13408,#13409,#13410,#13411));
#3759=EDGE_LOOP('',(#13412,#13413,#13414,#13415));
#3760=EDGE_LOOP('',(#13416,#13417,#13418,#13419));
#3761=EDGE_LOOP('',(#13420,#13421,#13422,#13423));
#3762=EDGE_LOOP('',(#13424,#13425,#13426,#13427));
#3763=EDGE_LOOP('',(#13428,#13429,#13430,#13431));
#3764=EDGE_LOOP('',(#13432,#13433,#13434,#13435));
#3765=EDGE_LOOP('',(#13436,#13437,#13438,#13439));
#3766=EDGE_LOOP('',(#13440,#13441,#13442,#13443));
#3767=EDGE_LOOP('',(#13444,#13445,#13446,#13447));
#3768=EDGE_LOOP('',(#13448,#13449,#13450,#13451));
#3769=EDGE_LOOP('',(#13452,#13453,#13454,#13455));
#3770=EDGE_LOOP('',(#13456,#13457,#13458,#13459));
#3771=EDGE_LOOP('',(#13460,#13461,#13462,#13463));
#3772=EDGE_LOOP('',(#13464,#13465,#13466,#13467));
#3773=EDGE_LOOP('',(#13468,#13469,#13470,#13471));
#3774=EDGE_LOOP('',(#13472,#13473,#13474,#13475));
#3775=EDGE_LOOP('',(#13476,#13477,#13478,#13479));
#3776=EDGE_LOOP('',(#13480,#13481,#13482,#13483));
#3777=EDGE_LOOP('',(#13484,#13485,#13486,#13487));
#3778=EDGE_LOOP('',(#13488,#13489,#13490,#13491));
#3779=EDGE_LOOP('',(#13492,#13493,#13494,#13495));
#3780=EDGE_LOOP('',(#13496,#13497,#13498,#13499));
#3781=EDGE_LOOP('',(#13500,#13501,#13502,#13503));
#3782=EDGE_LOOP('',(#13504,#13505,#13506,#13507));
#3783=EDGE_LOOP('',(#13508,#13509,#13510,#13511));
#3784=EDGE_LOOP('',(#13512,#13513,#13514,#13515));
#3785=EDGE_LOOP('',(#13516,#13517,#13518,#13519));
#3786=EDGE_LOOP('',(#13520,#13521,#13522,#13523));
#3787=EDGE_LOOP('',(#13524,#13525,#13526,#13527));
#3788=EDGE_LOOP('',(#13528,#13529,#13530,#13531));
#3789=EDGE_LOOP('',(#13532,#13533,#13534,#13535));
#3790=EDGE_LOOP('',(#13536,#13537,#13538,#13539));
#3791=EDGE_LOOP('',(#13540,#13541,#13542,#13543));
#3792=EDGE_LOOP('',(#13544,#13545,#13546,#13547));
#3793=EDGE_LOOP('',(#13548,#13549,#13550,#13551));
#3794=EDGE_LOOP('',(#13552,#13553,#13554,#13555));
#3795=EDGE_LOOP('',(#13556,#13557,#13558,#13559));
#3796=EDGE_LOOP('',(#13560,#13561,#13562,#13563));
#3797=EDGE_LOOP('',(#13564,#13565,#13566,#13567));
#3798=EDGE_LOOP('',(#13568,#13569,#13570,#13571));
#3799=EDGE_LOOP('',(#13572,#13573,#13574,#13575));
#3800=EDGE_LOOP('',(#13576,#13577,#13578,#13579));
#3801=EDGE_LOOP('',(#13580,#13581,#13582,#13583));
#3802=EDGE_LOOP('',(#13584,#13585,#13586,#13587));
#3803=EDGE_LOOP('',(#13588,#13589,#13590,#13591));
#3804=EDGE_LOOP('',(#13592,#13593,#13594,#13595,#13596,#13597,#13598,#13599,
#13600,#13601,#13602,#13603,#13604,#13605,#13606,#13607,#13608,#13609,#13610,
#13611,#13612,#13613,#13614,#13615,#13616,#13617,#13618,#13619,#13620,#13621,
#13622,#13623,#13624,#13625,#13626,#13627,#13628,#13629,#13630,#13631,#13632,
#13633,#13634,#13635,#13636,#13637,#13638,#13639,#13640,#13641,#13642,#13643,
#13644,#13645,#13646,#13647,#13648,#13649,#13650,#13651,#13652,#13653,#13654,
#13655,#13656,#13657,#13658,#13659,#13660,#13661,#13662,#13663,#13664,#13665,
#13666,#13667,#13668,#13669,#13670,#13671));
#3805=EDGE_LOOP('',(#13672));
#3806=EDGE_LOOP('',(#13673,#13674,#13675,#13676));
#4704=LINE('',#37665,#5728);
#4705=LINE('',#37667,#5729);
#4706=LINE('',#37669,#5730);
#4707=LINE('',#37670,#5731);
#4708=LINE('',#37673,#5732);
#4709=LINE('',#37675,#5733);
#4710=LINE('',#37676,#5734);
#4711=LINE('',#37679,#5735);
#4712=LINE('',#37681,#5736);
#4713=LINE('',#37682,#5737);
#4714=LINE('',#37765,#5738);
#4715=LINE('',#37911,#5739);
#4716=LINE('',#38057,#5740);
#4717=LINE('',#38203,#5741);
#4718=LINE('',#38349,#5742);
#4719=LINE('',#38495,#5743);
#4720=LINE('',#38641,#5744);
#4721=LINE('',#38787,#5745);
#4722=LINE('',#38933,#5746);
#4723=LINE('',#39079,#5747);
#4724=LINE('',#39225,#5748);
#4725=LINE('',#39371,#5749);
#4726=LINE('',#39517,#5750);
#4727=LINE('',#39663,#5751);
#4728=LINE('',#39809,#5752);
#4729=LINE('',#39955,#5753);
#4730=LINE('',#40101,#5754);
#4731=LINE('',#40247,#5755);
#4732=LINE('',#40393,#5756);
#4733=LINE('',#40539,#5757);
#4734=LINE('',#40612,#5758);
#4735=LINE('',#40755,#5759);
#4736=LINE('',#40827,#5760);
#4737=LINE('',#40830,#5761);
#4738=LINE('',#40831,#5762);
#4739=LINE('',#41043,#5763);
#4740=LINE('',#41047,#5764);
#4741=LINE('',#41259,#5765);
#4742=LINE('',#41262,#5766);
#4743=LINE('',#41263,#5767);
#4744=LINE('',#41475,#5768);
#4745=LINE('',#41479,#5769);
#4746=LINE('',#41691,#5770);
#4747=LINE('',#41694,#5771);
#4748=LINE('',#41695,#5772);
#4749=LINE('',#41907,#5773);
#4750=LINE('',#41911,#5774);
#4751=LINE('',#42123,#5775);
#4752=LINE('',#42126,#5776);
#4753=LINE('',#42127,#5777);
#4754=LINE('',#42339,#5778);
#4755=LINE('',#42343,#5779);
#4756=LINE('',#42555,#5780);
#4757=LINE('',#42558,#5781);
#4758=LINE('',#42559,#5782);
#4759=LINE('',#42771,#5783);
#4760=LINE('',#42775,#5784);
#4761=LINE('',#42987,#5785);
#4762=LINE('',#42990,#5786);
#4763=LINE('',#42991,#5787);
#4764=LINE('',#43203,#5788);
#4765=LINE('',#43207,#5789);
#4766=LINE('',#43419,#5790);
#4767=LINE('',#43422,#5791);
#4768=LINE('',#43423,#5792);
#4769=LINE('',#43635,#5793);
#4770=LINE('',#43639,#5794);
#4771=LINE('',#43851,#5795);
#4772=LINE('',#43854,#5796);
#4773=LINE('',#43855,#5797);
#4774=LINE('',#44067,#5798);
#4775=LINE('',#44071,#5799);
#4776=LINE('',#44283,#5800);
#4777=LINE('',#44286,#5801);
#4778=LINE('',#44287,#5802);
#4779=LINE('',#44499,#5803);
#4780=LINE('',#44503,#5804);
#4781=LINE('',#44715,#5805);
#4782=LINE('',#44718,#5806);
#4783=LINE('',#44719,#5807);
#4784=LINE('',#44931,#5808);
#4785=LINE('',#44935,#5809);
#4786=LINE('',#45147,#5810);
#4787=LINE('',#45150,#5811);
#4788=LINE('',#45151,#5812);
#4789=LINE('',#45363,#5813);
#4790=LINE('',#45367,#5814);
#4791=LINE('',#45579,#5815);
#4792=LINE('',#45582,#5816);
#4793=LINE('',#45583,#5817);
#4794=LINE('',#45795,#5818);
#4795=LINE('',#45799,#5819);
#4796=LINE('',#46011,#5820);
#4797=LINE('',#46014,#5821);
#4798=LINE('',#46015,#5822);
#4799=LINE('',#46227,#5823);
#4800=LINE('',#46231,#5824);
#4801=LINE('',#46443,#5825);
#4802=LINE('',#46446,#5826);
#4803=LINE('',#46447,#5827);
#4804=LINE('',#46659,#5828);
#4805=LINE('',#46663,#5829);
#4806=LINE('',#46875,#5830);
#4807=LINE('',#46878,#5831);
#4808=LINE('',#46879,#5832);
#4809=LINE('',#47091,#5833);
#4810=LINE('',#47095,#5834);
#4811=LINE('',#47307,#5835);
#4812=LINE('',#47310,#5836);
#4813=LINE('',#47311,#5837);
#4814=LINE('',#47523,#5838);
#4815=LINE('',#47527,#5839);
#4816=LINE('',#47739,#5840);
#4817=LINE('',#47742,#5841);
#4818=LINE('',#47743,#5842);
#4819=LINE('',#47955,#5843);
#4820=LINE('',#47959,#5844);
#4821=LINE('',#48171,#5845);
#4822=LINE('',#48174,#5846);
#4823=LINE('',#48175,#5847);
#4824=LINE('',#48387,#5848);
#4825=LINE('',#48391,#5849);
#4826=LINE('',#48603,#5850);
#4827=LINE('',#48606,#5851);
#4828=LINE('',#48607,#5852);
#4829=LINE('',#48819,#5853);
#4830=LINE('',#48823,#5854);
#4831=LINE('',#49035,#5855);
#4832=LINE('',#49038,#5856);
#4833=LINE('',#49039,#5857);
#4834=LINE('',#49251,#5858);
#5728=VECTOR('',#21574,1.);
#5729=VECTOR('',#21575,1.);
#5730=VECTOR('',#21576,1.);
#5731=VECTOR('',#21577,1.);
#5732=VECTOR('',#21580,1.);
#5733=VECTOR('',#21581,1.);
#5734=VECTOR('',#21582,1.);
#5735=VECTOR('',#21585,1.);
#5736=VECTOR('',#21586,1.);
#5737=VECTOR('',#21587,1.);
#5738=VECTOR('',#21602,1.);
#5739=VECTOR('',#21605,1.);
#5740=VECTOR('',#21608,1.);
#5741=VECTOR('',#21611,1.);
#5742=VECTOR('',#21614,1.);
#5743=VECTOR('',#21617,1.);
#5744=VECTOR('',#21620,1.);
#5745=VECTOR('',#21623,1.);
#5746=VECTOR('',#21626,1.);
#5747=VECTOR('',#21629,1.);
#5748=VECTOR('',#21632,1.);
#5749=VECTOR('',#21635,1.);
#5750=VECTOR('',#21638,1.);
#5751=VECTOR('',#21641,1.);
#5752=VECTOR('',#21644,1.);
#5753=VECTOR('',#21647,1.);
#5754=VECTOR('',#21650,1.);
#5755=VECTOR('',#21653,1.);
#5756=VECTOR('',#21656,1.);
#5757=VECTOR('',#21659,1.);
#5758=VECTOR('',#21662,1.4);
#5759=VECTOR('',#21665,1.);
#5760=VECTOR('',#21666,1.);
#5761=VECTOR('',#21669,1.);
#5762=VECTOR('',#21670,1.);
#5763=VECTOR('',#21671,1.);
#5764=VECTOR('',#21676,1.);
#5765=VECTOR('',#21677,1.);
#5766=VECTOR('',#21680,1.);
#5767=VECTOR('',#21681,1.);
#5768=VECTOR('',#21682,1.);
#5769=VECTOR('',#21687,1.);
#5770=VECTOR('',#21688,1.);
#5771=VECTOR('',#21691,1.);
#5772=VECTOR('',#21692,1.);
#5773=VECTOR('',#21693,1.);
#5774=VECTOR('',#21698,1.);
#5775=VECTOR('',#21699,1.);
#5776=VECTOR('',#21702,1.);
#5777=VECTOR('',#21703,1.);
#5778=VECTOR('',#21704,1.);
#5779=VECTOR('',#21709,1.);
#5780=VECTOR('',#21710,1.);
#5781=VECTOR('',#21713,1.);
#5782=VECTOR('',#21714,1.);
#5783=VECTOR('',#21715,1.);
#5784=VECTOR('',#21720,1.);
#5785=VECTOR('',#21721,1.);
#5786=VECTOR('',#21724,1.);
#5787=VECTOR('',#21725,1.);
#5788=VECTOR('',#21726,1.);
#5789=VECTOR('',#21731,1.);
#5790=VECTOR('',#21732,1.);
#5791=VECTOR('',#21735,1.);
#5792=VECTOR('',#21736,1.);
#5793=VECTOR('',#21737,1.);
#5794=VECTOR('',#21742,1.);
#5795=VECTOR('',#21743,1.);
#5796=VECTOR('',#21746,1.);
#5797=VECTOR('',#21747,1.);
#5798=VECTOR('',#21748,1.);
#5799=VECTOR('',#21753,1.);
#5800=VECTOR('',#21754,1.);
#5801=VECTOR('',#21757,1.);
#5802=VECTOR('',#21758,1.);
#5803=VECTOR('',#21759,1.);
#5804=VECTOR('',#21764,1.);
#5805=VECTOR('',#21765,1.);
#5806=VECTOR('',#21768,1.);
#5807=VECTOR('',#21769,1.);
#5808=VECTOR('',#21770,1.);
#5809=VECTOR('',#21775,1.);
#5810=VECTOR('',#21776,1.);
#5811=VECTOR('',#21779,1.);
#5812=VECTOR('',#21780,1.);
#5813=VECTOR('',#21781,1.);
#5814=VECTOR('',#21786,1.);
#5815=VECTOR('',#21787,1.);
#5816=VECTOR('',#21790,1.);
#5817=VECTOR('',#21791,1.);
#5818=VECTOR('',#21792,1.);
#5819=VECTOR('',#21797,1.);
#5820=VECTOR('',#21798,1.);
#5821=VECTOR('',#21801,1.);
#5822=VECTOR('',#21802,1.);
#5823=VECTOR('',#21803,1.);
#5824=VECTOR('',#21808,1.);
#5825=VECTOR('',#21809,1.);
#5826=VECTOR('',#21812,1.);
#5827=VECTOR('',#21813,1.);
#5828=VECTOR('',#21814,1.);
#5829=VECTOR('',#21819,1.);
#5830=VECTOR('',#21820,1.);
#5831=VECTOR('',#21823,1.);
#5832=VECTOR('',#21824,1.);
#5833=VECTOR('',#21825,1.);
#5834=VECTOR('',#21830,1.);
#5835=VECTOR('',#21831,1.);
#5836=VECTOR('',#21834,1.);
#5837=VECTOR('',#21835,1.);
#5838=VECTOR('',#21836,1.);
#5839=VECTOR('',#21841,1.);
#5840=VECTOR('',#21842,1.);
#5841=VECTOR('',#21845,1.);
#5842=VECTOR('',#21846,1.);
#5843=VECTOR('',#21847,1.);
#5844=VECTOR('',#21852,1.);
#5845=VECTOR('',#21853,1.);
#5846=VECTOR('',#21856,1.);
#5847=VECTOR('',#21857,1.);
#5848=VECTOR('',#21858,1.);
#5849=VECTOR('',#21863,1.);
#5850=VECTOR('',#21864,1.);
#5851=VECTOR('',#21867,1.);
#5852=VECTOR('',#21868,1.);
#5853=VECTOR('',#21869,1.);
#5854=VECTOR('',#21874,1.);
#5855=VECTOR('',#21875,1.);
#5856=VECTOR('',#21878,1.);
#5857=VECTOR('',#21879,1.);
#5858=VECTOR('',#21880,1.);
#6658=CIRCLE('',#18049,1.4);
#6659=CIRCLE('',#18050,1.);
#6660=CIRCLE('',#18052,1.);
#6661=CIRCLE('',#18054,1.75);
#6662=CIRCLE('',#18055,1.75);
#6663=CIRCLE('',#18056,1.75);
#6664=CIRCLE('',#18057,1.75);
#6665=CIRCLE('',#18058,1.75);
#6666=CIRCLE('',#18059,1.75);
#6667=CIRCLE('',#18060,1.75);
#6668=CIRCLE('',#18061,1.75);
#6669=CIRCLE('',#18062,1.75);
#6670=CIRCLE('',#18063,1.75);
#6671=CIRCLE('',#18064,1.75);
#6672=CIRCLE('',#18065,1.75);
#6673=CIRCLE('',#18066,1.75);
#6674=CIRCLE('',#18067,1.75);
#6675=CIRCLE('',#18068,1.75);
#6676=CIRCLE('',#18069,1.75);
#6677=CIRCLE('',#18070,1.75);
#6678=CIRCLE('',#18071,1.75);
#6679=CIRCLE('',#18072,1.75);
#6680=CIRCLE('',#18073,1.75);
#6681=CIRCLE('',#18075,1.4);
#6682=CIRCLE('',#18078,1.75);
#6683=CIRCLE('',#18081,1.75);
#6684=CIRCLE('',#18084,1.75);
#6685=CIRCLE('',#18087,1.75);
#6686=CIRCLE('',#18090,1.75);
#6687=CIRCLE('',#18093,1.75);
#6688=CIRCLE('',#18096,1.75);
#6689=CIRCLE('',#18099,1.75);
#6690=CIRCLE('',#18102,1.75);
#6691=CIRCLE('',#18105,1.75);
#6692=CIRCLE('',#18108,1.75);
#6693=CIRCLE('',#18111,1.75);
#6694=CIRCLE('',#18114,1.75);
#6695=CIRCLE('',#18117,1.75);
#6696=CIRCLE('',#18120,1.75);
#6697=CIRCLE('',#18123,1.75);
#6698=CIRCLE('',#18126,1.75);
#6699=CIRCLE('',#18129,1.75);
#6700=CIRCLE('',#18132,1.75);
#6701=CIRCLE('',#18135,1.75);
#7727=VERTEX_POINT('',#37663);
#7728=VERTEX_POINT('',#37664);
#7729=VERTEX_POINT('',#37666);
#7730=VERTEX_POINT('',#37668);
#7731=VERTEX_POINT('',#37672);
#7732=VERTEX_POINT('',#37674);
#7733=VERTEX_POINT('',#37678);
#7734=VERTEX_POINT('',#37680);
#7735=VERTEX_POINT('',#37684);
#7736=VERTEX_POINT('',#37690);
#7737=VERTEX_POINT('',#37691);
#7738=VERTEX_POINT('',#37693);
#7739=VERTEX_POINT('',#37764);
#7740=VERTEX_POINT('',#37766);
#7741=VERTEX_POINT('',#37837);
#7742=VERTEX_POINT('',#37839);
#7743=VERTEX_POINT('',#37910);
#7744=VERTEX_POINT('',#37912);
#7745=VERTEX_POINT('',#37983);
#7746=VERTEX_POINT('',#37985);
#7747=VERTEX_POINT('',#38056);
#7748=VERTEX_POINT('',#38058);
#7749=VERTEX_POINT('',#38129);
#7750=VERTEX_POINT('',#38131);
#7751=VERTEX_POINT('',#38202);
#7752=VERTEX_POINT('',#38204);
#7753=VERTEX_POINT('',#38275);
#7754=VERTEX_POINT('',#38277);
#7755=VERTEX_POINT('',#38348);
#7756=VERTEX_POINT('',#38350);
#7757=VERTEX_POINT('',#38421);
#7758=VERTEX_POINT('',#38423);
#7759=VERTEX_POINT('',#38494);
#7760=VERTEX_POINT('',#38496);
#7761=VERTEX_POINT('',#38567);
#7762=VERTEX_POINT('',#38569);
#7763=VERTEX_POINT('',#38640);
#7764=VERTEX_POINT('',#38642);
#7765=VERTEX_POINT('',#38713);
#7766=VERTEX_POINT('',#38715);
#7767=VERTEX_POINT('',#38786);
#7768=VERTEX_POINT('',#38788);
#7769=VERTEX_POINT('',#38859);
#7770=VERTEX_POINT('',#38861);
#7771=VERTEX_POINT('',#38932);
#7772=VERTEX_POINT('',#38934);
#7773=VERTEX_POINT('',#39005);
#7774=VERTEX_POINT('',#39007);
#7775=VERTEX_POINT('',#39078);
#7776=VERTEX_POINT('',#39080);
#7777=VERTEX_POINT('',#39151);
#7778=VERTEX_POINT('',#39153);
#7779=VERTEX_POINT('',#39224);
#7780=VERTEX_POINT('',#39226);
#7781=VERTEX_POINT('',#39297);
#7782=VERTEX_POINT('',#39299);
#7783=VERTEX_POINT('',#39370);
#7784=VERTEX_POINT('',#39372);
#7785=VERTEX_POINT('',#39443);
#7786=VERTEX_POINT('',#39445);
#7787=VERTEX_POINT('',#39516);
#7788=VERTEX_POINT('',#39518);
#7789=VERTEX_POINT('',#39589);
#7790=VERTEX_POINT('',#39591);
#7791=VERTEX_POINT('',#39662);
#7792=VERTEX_POINT('',#39664);
#7793=VERTEX_POINT('',#39735);
#7794=VERTEX_POINT('',#39737);
#7795=VERTEX_POINT('',#39808);
#7796=VERTEX_POINT('',#39810);
#7797=VERTEX_POINT('',#39881);
#7798=VERTEX_POINT('',#39883);
#7799=VERTEX_POINT('',#39954);
#7800=VERTEX_POINT('',#39956);
#7801=VERTEX_POINT('',#40027);
#7802=VERTEX_POINT('',#40029);
#7803=VERTEX_POINT('',#40100);
#7804=VERTEX_POINT('',#40102);
#7805=VERTEX_POINT('',#40173);
#7806=VERTEX_POINT('',#40175);
#7807=VERTEX_POINT('',#40246);
#7808=VERTEX_POINT('',#40248);
#7809=VERTEX_POINT('',#40319);
#7810=VERTEX_POINT('',#40321);
#7811=VERTEX_POINT('',#40392);
#7812=VERTEX_POINT('',#40394);
#7813=VERTEX_POINT('',#40465);
#7814=VERTEX_POINT('',#40467);
#7815=VERTEX_POINT('',#40538);
#7816=VERTEX_POINT('',#40611);
#7817=VERTEX_POINT('',#40754);
#7818=VERTEX_POINT('',#40756);
#7819=VERTEX_POINT('',#40829);
#7820=VERTEX_POINT('',#40972);
#7821=VERTEX_POINT('',#41045);
#7822=VERTEX_POINT('',#41188);
#7823=VERTEX_POINT('',#41261);
#7824=VERTEX_POINT('',#41404);
#7825=VERTEX_POINT('',#41477);
#7826=VERTEX_POINT('',#41620);
#7827=VERTEX_POINT('',#41693);
#7828=VERTEX_POINT('',#41836);
#7829=VERTEX_POINT('',#41909);
#7830=VERTEX_POINT('',#42052);
#7831=VERTEX_POINT('',#42125);
#7832=VERTEX_POINT('',#42268);
#7833=VERTEX_POINT('',#42341);
#7834=VERTEX_POINT('',#42484);
#7835=VERTEX_POINT('',#42557);
#7836=VERTEX_POINT('',#42700);
#7837=VERTEX_POINT('',#42773);
#7838=VERTEX_POINT('',#42916);
#7839=VERTEX_POINT('',#42989);
#7840=VERTEX_POINT('',#43132);
#7841=VERTEX_POINT('',#43205);
#7842=VERTEX_POINT('',#43348);
#7843=VERTEX_POINT('',#43421);
#7844=VERTEX_POINT('',#43564);
#7845=VERTEX_POINT('',#43637);
#7846=VERTEX_POINT('',#43780);
#7847=VERTEX_POINT('',#43853);
#7848=VERTEX_POINT('',#43996);
#7849=VERTEX_POINT('',#44069);
#7850=VERTEX_POINT('',#44212);
#7851=VERTEX_POINT('',#44285);
#7852=VERTEX_POINT('',#44428);
#7853=VERTEX_POINT('',#44501);
#7854=VERTEX_POINT('',#44644);
#7855=VERTEX_POINT('',#44717);
#7856=VERTEX_POINT('',#44860);
#7857=VERTEX_POINT('',#44933);
#7858=VERTEX_POINT('',#45076);
#7859=VERTEX_POINT('',#45149);
#7860=VERTEX_POINT('',#45292);
#7861=VERTEX_POINT('',#45365);
#7862=VERTEX_POINT('',#45508);
#7863=VERTEX_POINT('',#45581);
#7864=VERTEX_POINT('',#45724);
#7865=VERTEX_POINT('',#45797);
#7866=VERTEX_POINT('',#45940);
#7867=VERTEX_POINT('',#46013);
#7868=VERTEX_POINT('',#46156);
#7869=VERTEX_POINT('',#46229);
#7870=VERTEX_POINT('',#46372);
#7871=VERTEX_POINT('',#46445);
#7872=VERTEX_POINT('',#46588);
#7873=VERTEX_POINT('',#46661);
#7874=VERTEX_POINT('',#46804);
#7875=VERTEX_POINT('',#46877);
#7876=VERTEX_POINT('',#47020);
#7877=VERTEX_POINT('',#47093);
#7878=VERTEX_POINT('',#47236);
#7879=VERTEX_POINT('',#47309);
#7880=VERTEX_POINT('',#47452);
#7881=VERTEX_POINT('',#47525);
#7882=VERTEX_POINT('',#47668);
#7883=VERTEX_POINT('',#47741);
#7884=VERTEX_POINT('',#47884);
#7885=VERTEX_POINT('',#47957);
#7886=VERTEX_POINT('',#48100);
#7887=VERTEX_POINT('',#48173);
#7888=VERTEX_POINT('',#48316);
#7889=VERTEX_POINT('',#48389);
#7890=VERTEX_POINT('',#48532);
#7891=VERTEX_POINT('',#48605);
#7892=VERTEX_POINT('',#48748);
#7893=VERTEX_POINT('',#48821);
#7894=VERTEX_POINT('',#48964);
#7895=VERTEX_POINT('',#49037);
#7896=VERTEX_POINT('',#49180);
#9637=EDGE_CURVE('',#7727,#7728,#4704,.T.);
#9638=EDGE_CURVE('',#7727,#7729,#4705,.T.);
#9639=EDGE_CURVE('',#7730,#7729,#4706,.T.);
#9640=EDGE_CURVE('',#7728,#7730,#4707,.T.);
#9641=EDGE_CURVE('',#7731,#7727,#4708,.T.);
#9642=EDGE_CURVE('',#7731,#7732,#4709,.T.);
#9643=EDGE_CURVE('',#7729,#7732,#4710,.T.);
#9644=EDGE_CURVE('',#7733,#7731,#4711,.T.);
#9645=EDGE_CURVE('',#7734,#7733,#4712,.T.);
#9646=EDGE_CURVE('',#7732,#7734,#4713,.T.);
#9647=EDGE_CURVE('',#7735,#7735,#6658,.T.);
#9648=EDGE_CURVE('',#7734,#7730,#6659,.T.);
#9649=EDGE_CURVE('',#7728,#7733,#6660,.T.);
#9650=EDGE_CURVE('',#7736,#7737,#6661,.T.);
#9651=EDGE_CURVE('',#7737,#7738,#251,.T.);
#9652=EDGE_CURVE('',#7738,#7739,#4714,.T.);
#9653=EDGE_CURVE('',#7739,#7740,#252,.T.);
#9654=EDGE_CURVE('',#7740,#7741,#6662,.T.);
#9655=EDGE_CURVE('',#7741,#7742,#253,.T.);
#9656=EDGE_CURVE('',#7742,#7743,#4715,.T.);
#9657=EDGE_CURVE('',#7743,#7744,#254,.T.);
#9658=EDGE_CURVE('',#7744,#7745,#6663,.T.);
#9659=EDGE_CURVE('',#7745,#7746,#255,.T.);
#9660=EDGE_CURVE('',#7746,#7747,#4716,.T.);
#9661=EDGE_CURVE('',#7747,#7748,#256,.T.);
#9662=EDGE_CURVE('',#7748,#7749,#6664,.T.);
#9663=EDGE_CURVE('',#7749,#7750,#257,.T.);
#9664=EDGE_CURVE('',#7750,#7751,#4717,.T.);
#9665=EDGE_CURVE('',#7751,#7752,#258,.T.);
#9666=EDGE_CURVE('',#7752,#7753,#6665,.T.);
#9667=EDGE_CURVE('',#7753,#7754,#259,.T.);
#9668=EDGE_CURVE('',#7754,#7755,#4718,.T.);
#9669=EDGE_CURVE('',#7755,#7756,#260,.T.);
#9670=EDGE_CURVE('',#7756,#7757,#6666,.T.);
#9671=EDGE_CURVE('',#7757,#7758,#261,.T.);
#9672=EDGE_CURVE('',#7758,#7759,#4719,.T.);
#9673=EDGE_CURVE('',#7759,#7760,#262,.T.);
#9674=EDGE_CURVE('',#7760,#7761,#6667,.T.);
#9675=EDGE_CURVE('',#7761,#7762,#263,.T.);
#9676=EDGE_CURVE('',#7762,#7763,#4720,.T.);
#9677=EDGE_CURVE('',#7763,#7764,#264,.T.);
#9678=EDGE_CURVE('',#7764,#7765,#6668,.T.);
#9679=EDGE_CURVE('',#7765,#7766,#265,.T.);
#9680=EDGE_CURVE('',#7766,#7767,#4721,.T.);
#9681=EDGE_CURVE('',#7767,#7768,#266,.T.);
#9682=EDGE_CURVE('',#7768,#7769,#6669,.T.);
#9683=EDGE_CURVE('',#7769,#7770,#267,.T.);
#9684=EDGE_CURVE('',#7770,#7771,#4722,.T.);
#9685=EDGE_CURVE('',#7771,#7772,#268,.T.);
#9686=EDGE_CURVE('',#7772,#7773,#6670,.T.);
#9687=EDGE_CURVE('',#7773,#7774,#269,.T.);
#9688=EDGE_CURVE('',#7774,#7775,#4723,.T.);
#9689=EDGE_CURVE('',#7775,#7776,#270,.T.);
#9690=EDGE_CURVE('',#7776,#7777,#6671,.T.);
#9691=EDGE_CURVE('',#7777,#7778,#271,.T.);
#9692=EDGE_CURVE('',#7778,#7779,#4724,.T.);
#9693=EDGE_CURVE('',#7779,#7780,#272,.T.);
#9694=EDGE_CURVE('',#7780,#7781,#6672,.T.);
#9695=EDGE_CURVE('',#7781,#7782,#273,.T.);
#9696=EDGE_CURVE('',#7782,#7783,#4725,.T.);
#9697=EDGE_CURVE('',#7783,#7784,#274,.T.);
#9698=EDGE_CURVE('',#7784,#7785,#6673,.T.);
#9699=EDGE_CURVE('',#7785,#7786,#275,.T.);
#9700=EDGE_CURVE('',#7786,#7787,#4726,.T.);
#9701=EDGE_CURVE('',#7787,#7788,#276,.T.);
#9702=EDGE_CURVE('',#7788,#7789,#6674,.T.);
#9703=EDGE_CURVE('',#7789,#7790,#277,.T.);
#9704=EDGE_CURVE('',#7790,#7791,#4727,.T.);
#9705=EDGE_CURVE('',#7791,#7792,#278,.T.);
#9706=EDGE_CURVE('',#7792,#7793,#6675,.T.);
#9707=EDGE_CURVE('',#7793,#7794,#279,.T.);
#9708=EDGE_CURVE('',#7794,#7795,#4728,.T.);
#9709=EDGE_CURVE('',#7795,#7796,#280,.T.);
#9710=EDGE_CURVE('',#7796,#7797,#6676,.T.);
#9711=EDGE_CURVE('',#7797,#7798,#281,.T.);
#9712=EDGE_CURVE('',#7798,#7799,#4729,.T.);
#9713=EDGE_CURVE('',#7799,#7800,#282,.T.);
#9714=EDGE_CURVE('',#7800,#7801,#6677,.T.);
#9715=EDGE_CURVE('',#7801,#7802,#283,.T.);
#9716=EDGE_CURVE('',#7802,#7803,#4730,.T.);
#9717=EDGE_CURVE('',#7803,#7804,#284,.T.);
#9718=EDGE_CURVE('',#7804,#7805,#6678,.T.);
#9719=EDGE_CURVE('',#7805,#7806,#285,.T.);
#9720=EDGE_CURVE('',#7806,#7807,#4731,.T.);
#9721=EDGE_CURVE('',#7807,#7808,#286,.T.);
#9722=EDGE_CURVE('',#7808,#7809,#6679,.T.);
#9723=EDGE_CURVE('',#7809,#7810,#287,.T.);
#9724=EDGE_CURVE('',#7810,#7811,#4732,.T.);
#9725=EDGE_CURVE('',#7811,#7812,#288,.T.);
#9726=EDGE_CURVE('',#7812,#7813,#6680,.T.);
#9727=EDGE_CURVE('',#7813,#7814,#289,.T.);
#9728=EDGE_CURVE('',#7814,#7815,#4733,.T.);
#9729=EDGE_CURVE('',#7815,#7736,#290,.T.);
#9730=EDGE_CURVE('',#7735,#7816,#4734,.T.);
#9731=EDGE_CURVE('',#7816,#7816,#6681,.T.);
#9732=EDGE_CURVE('',#7817,#7813,#4735,.T.);
#9733=EDGE_CURVE('',#7818,#7817,#291,.T.);
#9734=EDGE_CURVE('',#7814,#7818,#4736,.T.);
#9735=EDGE_CURVE('',#7819,#7818,#4737,.T.);
#9736=EDGE_CURVE('',#7815,#7819,#4738,.T.);
#9737=EDGE_CURVE('',#7820,#7819,#292,.T.);
#9738=EDGE_CURVE('',#7736,#7820,#4739,.T.);
#9739=EDGE_CURVE('',#7821,#7820,#6682,.T.);
#9740=EDGE_CURVE('',#7821,#7737,#4740,.T.);
#9741=EDGE_CURVE('',#7822,#7821,#293,.T.);
#9742=EDGE_CURVE('',#7738,#7822,#4741,.T.);
#9743=EDGE_CURVE('',#7823,#7822,#4742,.T.);
#9744=EDGE_CURVE('',#7739,#7823,#4743,.T.);
#9745=EDGE_CURVE('',#7824,#7823,#294,.T.);
#9746=EDGE_CURVE('',#7740,#7824,#4744,.T.);
#9747=EDGE_CURVE('',#7825,#7824,#6683,.T.);
#9748=EDGE_CURVE('',#7825,#7741,#4745,.T.);
#9749=EDGE_CURVE('',#7826,#7825,#295,.T.);
#9750=EDGE_CURVE('',#7742,#7826,#4746,.T.);
#9751=EDGE_CURVE('',#7827,#7826,#4747,.T.);
#9752=EDGE_CURVE('',#7743,#7827,#4748,.T.);
#9753=EDGE_CURVE('',#7828,#7827,#296,.T.);
#9754=EDGE_CURVE('',#7744,#7828,#4749,.T.);
#9755=EDGE_CURVE('',#7829,#7828,#6684,.T.);
#9756=EDGE_CURVE('',#7829,#7745,#4750,.T.);
#9757=EDGE_CURVE('',#7830,#7829,#297,.T.);
#9758=EDGE_CURVE('',#7746,#7830,#4751,.T.);
#9759=EDGE_CURVE('',#7831,#7830,#4752,.T.);
#9760=EDGE_CURVE('',#7747,#7831,#4753,.T.);
#9761=EDGE_CURVE('',#7832,#7831,#298,.T.);
#9762=EDGE_CURVE('',#7748,#7832,#4754,.T.);
#9763=EDGE_CURVE('',#7833,#7832,#6685,.T.);
#9764=EDGE_CURVE('',#7833,#7749,#4755,.T.);
#9765=EDGE_CURVE('',#7834,#7833,#299,.T.);
#9766=EDGE_CURVE('',#7750,#7834,#4756,.T.);
#9767=EDGE_CURVE('',#7835,#7834,#4757,.T.);
#9768=EDGE_CURVE('',#7751,#7835,#4758,.T.);
#9769=EDGE_CURVE('',#7836,#7835,#300,.T.);
#9770=EDGE_CURVE('',#7752,#7836,#4759,.T.);
#9771=EDGE_CURVE('',#7837,#7836,#6686,.T.);
#9772=EDGE_CURVE('',#7837,#7753,#4760,.T.);
#9773=EDGE_CURVE('',#7838,#7837,#301,.T.);
#9774=EDGE_CURVE('',#7754,#7838,#4761,.T.);
#9775=EDGE_CURVE('',#7839,#7838,#4762,.T.);
#9776=EDGE_CURVE('',#7755,#7839,#4763,.T.);
#9777=EDGE_CURVE('',#7840,#7839,#302,.T.);
#9778=EDGE_CURVE('',#7756,#7840,#4764,.T.);
#9779=EDGE_CURVE('',#7841,#7840,#6687,.T.);
#9780=EDGE_CURVE('',#7841,#7757,#4765,.T.);
#9781=EDGE_CURVE('',#7842,#7841,#303,.T.);
#9782=EDGE_CURVE('',#7758,#7842,#4766,.T.);
#9783=EDGE_CURVE('',#7843,#7842,#4767,.T.);
#9784=EDGE_CURVE('',#7759,#7843,#4768,.T.);
#9785=EDGE_CURVE('',#7844,#7843,#304,.T.);
#9786=EDGE_CURVE('',#7760,#7844,#4769,.T.);
#9787=EDGE_CURVE('',#7845,#7844,#6688,.T.);
#9788=EDGE_CURVE('',#7845,#7761,#4770,.T.);
#9789=EDGE_CURVE('',#7846,#7845,#305,.T.);
#9790=EDGE_CURVE('',#7762,#7846,#4771,.T.);
#9791=EDGE_CURVE('',#7847,#7846,#4772,.T.);
#9792=EDGE_CURVE('',#7763,#7847,#4773,.T.);
#9793=EDGE_CURVE('',#7848,#7847,#306,.T.);
#9794=EDGE_CURVE('',#7764,#7848,#4774,.T.);
#9795=EDGE_CURVE('',#7849,#7848,#6689,.T.);
#9796=EDGE_CURVE('',#7849,#7765,#4775,.T.);
#9797=EDGE_CURVE('',#7850,#7849,#307,.T.);
#9798=EDGE_CURVE('',#7766,#7850,#4776,.T.);
#9799=EDGE_CURVE('',#7851,#7850,#4777,.T.);
#9800=EDGE_CURVE('',#7767,#7851,#4778,.T.);
#9801=EDGE_CURVE('',#7852,#7851,#308,.T.);
#9802=EDGE_CURVE('',#7768,#7852,#4779,.T.);
#9803=EDGE_CURVE('',#7853,#7852,#6690,.T.);
#9804=EDGE_CURVE('',#7853,#7769,#4780,.T.);
#9805=EDGE_CURVE('',#7854,#7853,#309,.T.);
#9806=EDGE_CURVE('',#7770,#7854,#4781,.T.);
#9807=EDGE_CURVE('',#7855,#7854,#4782,.T.);
#9808=EDGE_CURVE('',#7771,#7855,#4783,.T.);
#9809=EDGE_CURVE('',#7856,#7855,#310,.T.);
#9810=EDGE_CURVE('',#7772,#7856,#4784,.T.);
#9811=EDGE_CURVE('',#7857,#7856,#6691,.T.);
#9812=EDGE_CURVE('',#7857,#7773,#4785,.T.);
#9813=EDGE_CURVE('',#7858,#7857,#311,.T.);
#9814=EDGE_CURVE('',#7774,#7858,#4786,.T.);
#9815=EDGE_CURVE('',#7859,#7858,#4787,.T.);
#9816=EDGE_CURVE('',#7775,#7859,#4788,.T.);
#9817=EDGE_CURVE('',#7860,#7859,#312,.T.);
#9818=EDGE_CURVE('',#7776,#7860,#4789,.T.);
#9819=EDGE_CURVE('',#7861,#7860,#6692,.T.);
#9820=EDGE_CURVE('',#7861,#7777,#4790,.T.);
#9821=EDGE_CURVE('',#7862,#7861,#313,.T.);
#9822=EDGE_CURVE('',#7778,#7862,#4791,.T.);
#9823=EDGE_CURVE('',#7863,#7862,#4792,.T.);
#9824=EDGE_CURVE('',#7779,#7863,#4793,.T.);
#9825=EDGE_CURVE('',#7864,#7863,#314,.T.);
#9826=EDGE_CURVE('',#7780,#7864,#4794,.T.);
#9827=EDGE_CURVE('',#7865,#7864,#6693,.T.);
#9828=EDGE_CURVE('',#7865,#7781,#4795,.T.);
#9829=EDGE_CURVE('',#7866,#7865,#315,.T.);
#9830=EDGE_CURVE('',#7782,#7866,#4796,.T.);
#9831=EDGE_CURVE('',#7867,#7866,#4797,.T.);
#9832=EDGE_CURVE('',#7783,#7867,#4798,.T.);
#9833=EDGE_CURVE('',#7868,#7867,#316,.T.);
#9834=EDGE_CURVE('',#7784,#7868,#4799,.T.);
#9835=EDGE_CURVE('',#7869,#7868,#6694,.T.);
#9836=EDGE_CURVE('',#7869,#7785,#4800,.T.);
#9837=EDGE_CURVE('',#7870,#7869,#317,.T.);
#9838=EDGE_CURVE('',#7786,#7870,#4801,.T.);
#9839=EDGE_CURVE('',#7871,#7870,#4802,.T.);
#9840=EDGE_CURVE('',#7787,#7871,#4803,.T.);
#9841=EDGE_CURVE('',#7872,#7871,#318,.T.);
#9842=EDGE_CURVE('',#7788,#7872,#4804,.T.);
#9843=EDGE_CURVE('',#7873,#7872,#6695,.T.);
#9844=EDGE_CURVE('',#7873,#7789,#4805,.T.);
#9845=EDGE_CURVE('',#7874,#7873,#319,.T.);
#9846=EDGE_CURVE('',#7790,#7874,#4806,.T.);
#9847=EDGE_CURVE('',#7875,#7874,#4807,.T.);
#9848=EDGE_CURVE('',#7791,#7875,#4808,.T.);
#9849=EDGE_CURVE('',#7876,#7875,#320,.T.);
#9850=EDGE_CURVE('',#7792,#7876,#4809,.T.);
#9851=EDGE_CURVE('',#7877,#7876,#6696,.T.);
#9852=EDGE_CURVE('',#7877,#7793,#4810,.T.);
#9853=EDGE_CURVE('',#7878,#7877,#321,.T.);
#9854=EDGE_CURVE('',#7794,#7878,#4811,.T.);
#9855=EDGE_CURVE('',#7879,#7878,#4812,.T.);
#9856=EDGE_CURVE('',#7795,#7879,#4813,.T.);
#9857=EDGE_CURVE('',#7880,#7879,#322,.T.);
#9858=EDGE_CURVE('',#7796,#7880,#4814,.T.);
#9859=EDGE_CURVE('',#7881,#7880,#6697,.T.);
#9860=EDGE_CURVE('',#7881,#7797,#4815,.T.);
#9861=EDGE_CURVE('',#7882,#7881,#323,.T.);
#9862=EDGE_CURVE('',#7798,#7882,#4816,.T.);
#9863=EDGE_CURVE('',#7883,#7882,#4817,.T.);
#9864=EDGE_CURVE('',#7799,#7883,#4818,.T.);
#9865=EDGE_CURVE('',#7884,#7883,#324,.T.);
#9866=EDGE_CURVE('',#7800,#7884,#4819,.T.);
#9867=EDGE_CURVE('',#7885,#7884,#6698,.T.);
#9868=EDGE_CURVE('',#7885,#7801,#4820,.T.);
#9869=EDGE_CURVE('',#7886,#7885,#325,.T.);
#9870=EDGE_CURVE('',#7802,#7886,#4821,.T.);
#9871=EDGE_CURVE('',#7887,#7886,#4822,.T.);
#9872=EDGE_CURVE('',#7803,#7887,#4823,.T.);
#9873=EDGE_CURVE('',#7888,#7887,#326,.T.);
#9874=EDGE_CURVE('',#7804,#7888,#4824,.T.);
#9875=EDGE_CURVE('',#7889,#7888,#6699,.T.);
#9876=EDGE_CURVE('',#7889,#7805,#4825,.T.);
#9877=EDGE_CURVE('',#7890,#7889,#327,.T.);
#9878=EDGE_CURVE('',#7806,#7890,#4826,.T.);
#9879=EDGE_CURVE('',#7891,#7890,#4827,.T.);
#9880=EDGE_CURVE('',#7807,#7891,#4828,.T.);
#9881=EDGE_CURVE('',#7892,#7891,#328,.T.);
#9882=EDGE_CURVE('',#7808,#7892,#4829,.T.);
#9883=EDGE_CURVE('',#7893,#7892,#6700,.T.);
#9884=EDGE_CURVE('',#7893,#7809,#4830,.T.);
#9885=EDGE_CURVE('',#7894,#7893,#329,.T.);
#9886=EDGE_CURVE('',#7810,#7894,#4831,.T.);
#9887=EDGE_CURVE('',#7895,#7894,#4832,.T.);
#9888=EDGE_CURVE('',#7811,#7895,#4833,.T.);
#9889=EDGE_CURVE('',#7896,#7895,#330,.T.);
#9890=EDGE_CURVE('',#7812,#7896,#4834,.T.);
#9891=EDGE_CURVE('',#7817,#7896,#6701,.T.);
#13167=ORIENTED_EDGE('',*,*,#9637,.F.);
#13168=ORIENTED_EDGE('',*,*,#9638,.T.);
#13169=ORIENTED_EDGE('',*,*,#9639,.F.);
#13170=ORIENTED_EDGE('',*,*,#9640,.F.);
#13171=ORIENTED_EDGE('',*,*,#9641,.F.);
#13172=ORIENTED_EDGE('',*,*,#9642,.T.);
#13173=ORIENTED_EDGE('',*,*,#9643,.F.);
#13174=ORIENTED_EDGE('',*,*,#9638,.F.);
#13175=ORIENTED_EDGE('',*,*,#9644,.F.);
#13176=ORIENTED_EDGE('',*,*,#9645,.F.);
#13177=ORIENTED_EDGE('',*,*,#9646,.F.);
#13178=ORIENTED_EDGE('',*,*,#9642,.F.);
#13179=ORIENTED_EDGE('',*,*,#9647,.T.);
#13180=ORIENTED_EDGE('',*,*,#9639,.T.);
#13181=ORIENTED_EDGE('',*,*,#9643,.T.);
#13182=ORIENTED_EDGE('',*,*,#9646,.T.);
#13183=ORIENTED_EDGE('',*,*,#9648,.T.);
#13184=ORIENTED_EDGE('',*,*,#9640,.T.);
#13185=ORIENTED_EDGE('',*,*,#9648,.F.);
#13186=ORIENTED_EDGE('',*,*,#9645,.T.);
#13187=ORIENTED_EDGE('',*,*,#9649,.F.);
#13188=ORIENTED_EDGE('',*,*,#9650,.T.);
#13189=ORIENTED_EDGE('',*,*,#9651,.T.);
#13190=ORIENTED_EDGE('',*,*,#9652,.T.);
#13191=ORIENTED_EDGE('',*,*,#9653,.T.);
#13192=ORIENTED_EDGE('',*,*,#9654,.T.);
#13193=ORIENTED_EDGE('',*,*,#9655,.T.);
#13194=ORIENTED_EDGE('',*,*,#9656,.T.);
#13195=ORIENTED_EDGE('',*,*,#9657,.T.);
#13196=ORIENTED_EDGE('',*,*,#9658,.T.);
#13197=ORIENTED_EDGE('',*,*,#9659,.T.);
#13198=ORIENTED_EDGE('',*,*,#9660,.T.);
#13199=ORIENTED_EDGE('',*,*,#9661,.T.);
#13200=ORIENTED_EDGE('',*,*,#9662,.T.);
#13201=ORIENTED_EDGE('',*,*,#9663,.T.);
#13202=ORIENTED_EDGE('',*,*,#9664,.T.);
#13203=ORIENTED_EDGE('',*,*,#9665,.T.);
#13204=ORIENTED_EDGE('',*,*,#9666,.T.);
#13205=ORIENTED_EDGE('',*,*,#9667,.T.);
#13206=ORIENTED_EDGE('',*,*,#9668,.T.);
#13207=ORIENTED_EDGE('',*,*,#9669,.T.);
#13208=ORIENTED_EDGE('',*,*,#9670,.T.);
#13209=ORIENTED_EDGE('',*,*,#9671,.T.);
#13210=ORIENTED_EDGE('',*,*,#9672,.T.);
#13211=ORIENTED_EDGE('',*,*,#9673,.T.);
#13212=ORIENTED_EDGE('',*,*,#9674,.T.);
#13213=ORIENTED_EDGE('',*,*,#9675,.T.);
#13214=ORIENTED_EDGE('',*,*,#9676,.T.);
#13215=ORIENTED_EDGE('',*,*,#9677,.T.);
#13216=ORIENTED_EDGE('',*,*,#9678,.T.);
#13217=ORIENTED_EDGE('',*,*,#9679,.T.);
#13218=ORIENTED_EDGE('',*,*,#9680,.T.);
#13219=ORIENTED_EDGE('',*,*,#9681,.T.);
#13220=ORIENTED_EDGE('',*,*,#9682,.T.);
#13221=ORIENTED_EDGE('',*,*,#9683,.T.);
#13222=ORIENTED_EDGE('',*,*,#9684,.T.);
#13223=ORIENTED_EDGE('',*,*,#9685,.T.);
#13224=ORIENTED_EDGE('',*,*,#9686,.T.);
#13225=ORIENTED_EDGE('',*,*,#9687,.T.);
#13226=ORIENTED_EDGE('',*,*,#9688,.T.);
#13227=ORIENTED_EDGE('',*,*,#9689,.T.);
#13228=ORIENTED_EDGE('',*,*,#9690,.T.);
#13229=ORIENTED_EDGE('',*,*,#9691,.T.);
#13230=ORIENTED_EDGE('',*,*,#9692,.T.);
#13231=ORIENTED_EDGE('',*,*,#9693,.T.);
#13232=ORIENTED_EDGE('',*,*,#9694,.T.);
#13233=ORIENTED_EDGE('',*,*,#9695,.T.);
#13234=ORIENTED_EDGE('',*,*,#9696,.T.);
#13235=ORIENTED_EDGE('',*,*,#9697,.T.);
#13236=ORIENTED_EDGE('',*,*,#9698,.T.);
#13237=ORIENTED_EDGE('',*,*,#9699,.T.);
#13238=ORIENTED_EDGE('',*,*,#9700,.T.);
#13239=ORIENTED_EDGE('',*,*,#9701,.T.);
#13240=ORIENTED_EDGE('',*,*,#9702,.T.);
#13241=ORIENTED_EDGE('',*,*,#9703,.T.);
#13242=ORIENTED_EDGE('',*,*,#9704,.T.);
#13243=ORIENTED_EDGE('',*,*,#9705,.T.);
#13244=ORIENTED_EDGE('',*,*,#9706,.T.);
#13245=ORIENTED_EDGE('',*,*,#9707,.T.);
#13246=ORIENTED_EDGE('',*,*,#9708,.T.);
#13247=ORIENTED_EDGE('',*,*,#9709,.T.);
#13248=ORIENTED_EDGE('',*,*,#9710,.T.);
#13249=ORIENTED_EDGE('',*,*,#9711,.T.);
#13250=ORIENTED_EDGE('',*,*,#9712,.T.);
#13251=ORIENTED_EDGE('',*,*,#9713,.T.);
#13252=ORIENTED_EDGE('',*,*,#9714,.T.);
#13253=ORIENTED_EDGE('',*,*,#9715,.T.);
#13254=ORIENTED_EDGE('',*,*,#9716,.T.);
#13255=ORIENTED_EDGE('',*,*,#9717,.T.);
#13256=ORIENTED_EDGE('',*,*,#9718,.T.);
#13257=ORIENTED_EDGE('',*,*,#9719,.T.);
#13258=ORIENTED_EDGE('',*,*,#9720,.T.);
#13259=ORIENTED_EDGE('',*,*,#9721,.T.);
#13260=ORIENTED_EDGE('',*,*,#9722,.T.);
#13261=ORIENTED_EDGE('',*,*,#9723,.T.);
#13262=ORIENTED_EDGE('',*,*,#9724,.T.);
#13263=ORIENTED_EDGE('',*,*,#9725,.T.);
#13264=ORIENTED_EDGE('',*,*,#9726,.T.);
#13265=ORIENTED_EDGE('',*,*,#9727,.T.);
#13266=ORIENTED_EDGE('',*,*,#9728,.T.);
#13267=ORIENTED_EDGE('',*,*,#9729,.T.);
#13268=ORIENTED_EDGE('',*,*,#9637,.T.);
#13269=ORIENTED_EDGE('',*,*,#9649,.T.);
#13270=ORIENTED_EDGE('',*,*,#9644,.T.);
#13271=ORIENTED_EDGE('',*,*,#9641,.T.);
#13272=ORIENTED_EDGE('',*,*,#9647,.F.);
#13273=ORIENTED_EDGE('',*,*,#9730,.T.);
#13274=ORIENTED_EDGE('',*,*,#9731,.F.);
#13275=ORIENTED_EDGE('',*,*,#9730,.F.);
#13276=ORIENTED_EDGE('',*,*,#9732,.F.);
#13277=ORIENTED_EDGE('',*,*,#9733,.F.);
#13278=ORIENTED_EDGE('',*,*,#9734,.F.);
#13279=ORIENTED_EDGE('',*,*,#9727,.F.);
#13280=ORIENTED_EDGE('',*,*,#9734,.T.);
#13281=ORIENTED_EDGE('',*,*,#9735,.F.);
#13282=ORIENTED_EDGE('',*,*,#9736,.F.);
#13283=ORIENTED_EDGE('',*,*,#9728,.F.);
#13284=ORIENTED_EDGE('',*,*,#9736,.T.);
#13285=ORIENTED_EDGE('',*,*,#9737,.F.);
#13286=ORIENTED_EDGE('',*,*,#9738,.F.);
#13287=ORIENTED_EDGE('',*,*,#9729,.F.);
#13288=ORIENTED_EDGE('',*,*,#9738,.T.);
#13289=ORIENTED_EDGE('',*,*,#9739,.F.);
#13290=ORIENTED_EDGE('',*,*,#9740,.T.);
#13291=ORIENTED_EDGE('',*,*,#9650,.F.);
#13292=ORIENTED_EDGE('',*,*,#9740,.F.);
#13293=ORIENTED_EDGE('',*,*,#9741,.F.);
#13294=ORIENTED_EDGE('',*,*,#9742,.F.);
#13295=ORIENTED_EDGE('',*,*,#9651,.F.);
#13296=ORIENTED_EDGE('',*,*,#9742,.T.);
#13297=ORIENTED_EDGE('',*,*,#9743,.F.);
#13298=ORIENTED_EDGE('',*,*,#9744,.F.);
#13299=ORIENTED_EDGE('',*,*,#9652,.F.);
#13300=ORIENTED_EDGE('',*,*,#9744,.T.);
#13301=ORIENTED_EDGE('',*,*,#9745,.F.);
#13302=ORIENTED_EDGE('',*,*,#9746,.F.);
#13303=ORIENTED_EDGE('',*,*,#9653,.F.);
#13304=ORIENTED_EDGE('',*,*,#9746,.T.);
#13305=ORIENTED_EDGE('',*,*,#9747,.F.);
#13306=ORIENTED_EDGE('',*,*,#9748,.T.);
#13307=ORIENTED_EDGE('',*,*,#9654,.F.);
#13308=ORIENTED_EDGE('',*,*,#9748,.F.);
#13309=ORIENTED_EDGE('',*,*,#9749,.F.);
#13310=ORIENTED_EDGE('',*,*,#9750,.F.);
#13311=ORIENTED_EDGE('',*,*,#9655,.F.);
#13312=ORIENTED_EDGE('',*,*,#9750,.T.);
#13313=ORIENTED_EDGE('',*,*,#9751,.F.);
#13314=ORIENTED_EDGE('',*,*,#9752,.F.);
#13315=ORIENTED_EDGE('',*,*,#9656,.F.);
#13316=ORIENTED_EDGE('',*,*,#9752,.T.);
#13317=ORIENTED_EDGE('',*,*,#9753,.F.);
#13318=ORIENTED_EDGE('',*,*,#9754,.F.);
#13319=ORIENTED_EDGE('',*,*,#9657,.F.);
#13320=ORIENTED_EDGE('',*,*,#9754,.T.);
#13321=ORIENTED_EDGE('',*,*,#9755,.F.);
#13322=ORIENTED_EDGE('',*,*,#9756,.T.);
#13323=ORIENTED_EDGE('',*,*,#9658,.F.);
#13324=ORIENTED_EDGE('',*,*,#9756,.F.);
#13325=ORIENTED_EDGE('',*,*,#9757,.F.);
#13326=ORIENTED_EDGE('',*,*,#9758,.F.);
#13327=ORIENTED_EDGE('',*,*,#9659,.F.);
#13328=ORIENTED_EDGE('',*,*,#9758,.T.);
#13329=ORIENTED_EDGE('',*,*,#9759,.F.);
#13330=ORIENTED_EDGE('',*,*,#9760,.F.);
#13331=ORIENTED_EDGE('',*,*,#9660,.F.);
#13332=ORIENTED_EDGE('',*,*,#9760,.T.);
#13333=ORIENTED_EDGE('',*,*,#9761,.F.);
#13334=ORIENTED_EDGE('',*,*,#9762,.F.);
#13335=ORIENTED_EDGE('',*,*,#9661,.F.);
#13336=ORIENTED_EDGE('',*,*,#9762,.T.);
#13337=ORIENTED_EDGE('',*,*,#9763,.F.);
#13338=ORIENTED_EDGE('',*,*,#9764,.T.);
#13339=ORIENTED_EDGE('',*,*,#9662,.F.);
#13340=ORIENTED_EDGE('',*,*,#9764,.F.);
#13341=ORIENTED_EDGE('',*,*,#9765,.F.);
#13342=ORIENTED_EDGE('',*,*,#9766,.F.);
#13343=ORIENTED_EDGE('',*,*,#9663,.F.);
#13344=ORIENTED_EDGE('',*,*,#9766,.T.);
#13345=ORIENTED_EDGE('',*,*,#9767,.F.);
#13346=ORIENTED_EDGE('',*,*,#9768,.F.);
#13347=ORIENTED_EDGE('',*,*,#9664,.F.);
#13348=ORIENTED_EDGE('',*,*,#9768,.T.);
#13349=ORIENTED_EDGE('',*,*,#9769,.F.);
#13350=ORIENTED_EDGE('',*,*,#9770,.F.);
#13351=ORIENTED_EDGE('',*,*,#9665,.F.);
#13352=ORIENTED_EDGE('',*,*,#9770,.T.);
#13353=ORIENTED_EDGE('',*,*,#9771,.F.);
#13354=ORIENTED_EDGE('',*,*,#9772,.T.);
#13355=ORIENTED_EDGE('',*,*,#9666,.F.);
#13356=ORIENTED_EDGE('',*,*,#9772,.F.);
#13357=ORIENTED_EDGE('',*,*,#9773,.F.);
#13358=ORIENTED_EDGE('',*,*,#9774,.F.);
#13359=ORIENTED_EDGE('',*,*,#9667,.F.);
#13360=ORIENTED_EDGE('',*,*,#9774,.T.);
#13361=ORIENTED_EDGE('',*,*,#9775,.F.);
#13362=ORIENTED_EDGE('',*,*,#9776,.F.);
#13363=ORIENTED_EDGE('',*,*,#9668,.F.);
#13364=ORIENTED_EDGE('',*,*,#9776,.T.);
#13365=ORIENTED_EDGE('',*,*,#9777,.F.);
#13366=ORIENTED_EDGE('',*,*,#9778,.F.);
#13367=ORIENTED_EDGE('',*,*,#9669,.F.);
#13368=ORIENTED_EDGE('',*,*,#9778,.T.);
#13369=ORIENTED_EDGE('',*,*,#9779,.F.);
#13370=ORIENTED_EDGE('',*,*,#9780,.T.);
#13371=ORIENTED_EDGE('',*,*,#9670,.F.);
#13372=ORIENTED_EDGE('',*,*,#9780,.F.);
#13373=ORIENTED_EDGE('',*,*,#9781,.F.);
#13374=ORIENTED_EDGE('',*,*,#9782,.F.);
#13375=ORIENTED_EDGE('',*,*,#9671,.F.);
#13376=ORIENTED_EDGE('',*,*,#9782,.T.);
#13377=ORIENTED_EDGE('',*,*,#9783,.F.);
#13378=ORIENTED_EDGE('',*,*,#9784,.F.);
#13379=ORIENTED_EDGE('',*,*,#9672,.F.);
#13380=ORIENTED_EDGE('',*,*,#9784,.T.);
#13381=ORIENTED_EDGE('',*,*,#9785,.F.);
#13382=ORIENTED_EDGE('',*,*,#9786,.F.);
#13383=ORIENTED_EDGE('',*,*,#9673,.F.);
#13384=ORIENTED_EDGE('',*,*,#9786,.T.);
#13385=ORIENTED_EDGE('',*,*,#9787,.F.);
#13386=ORIENTED_EDGE('',*,*,#9788,.T.);
#13387=ORIENTED_EDGE('',*,*,#9674,.F.);
#13388=ORIENTED_EDGE('',*,*,#9788,.F.);
#13389=ORIENTED_EDGE('',*,*,#9789,.F.);
#13390=ORIENTED_EDGE('',*,*,#9790,.F.);
#13391=ORIENTED_EDGE('',*,*,#9675,.F.);
#13392=ORIENTED_EDGE('',*,*,#9790,.T.);
#13393=ORIENTED_EDGE('',*,*,#9791,.F.);
#13394=ORIENTED_EDGE('',*,*,#9792,.F.);
#13395=ORIENTED_EDGE('',*,*,#9676,.F.);
#13396=ORIENTED_EDGE('',*,*,#9792,.T.);
#13397=ORIENTED_EDGE('',*,*,#9793,.F.);
#13398=ORIENTED_EDGE('',*,*,#9794,.F.);
#13399=ORIENTED_EDGE('',*,*,#9677,.F.);
#13400=ORIENTED_EDGE('',*,*,#9794,.T.);
#13401=ORIENTED_EDGE('',*,*,#9795,.F.);
#13402=ORIENTED_EDGE('',*,*,#9796,.T.);
#13403=ORIENTED_EDGE('',*,*,#9678,.F.);
#13404=ORIENTED_EDGE('',*,*,#9796,.F.);
#13405=ORIENTED_EDGE('',*,*,#9797,.F.);
#13406=ORIENTED_EDGE('',*,*,#9798,.F.);
#13407=ORIENTED_EDGE('',*,*,#9679,.F.);
#13408=ORIENTED_EDGE('',*,*,#9798,.T.);
#13409=ORIENTED_EDGE('',*,*,#9799,.F.);
#13410=ORIENTED_EDGE('',*,*,#9800,.F.);
#13411=ORIENTED_EDGE('',*,*,#9680,.F.);
#13412=ORIENTED_EDGE('',*,*,#9800,.T.);
#13413=ORIENTED_EDGE('',*,*,#9801,.F.);
#13414=ORIENTED_EDGE('',*,*,#9802,.F.);
#13415=ORIENTED_EDGE('',*,*,#9681,.F.);
#13416=ORIENTED_EDGE('',*,*,#9802,.T.);
#13417=ORIENTED_EDGE('',*,*,#9803,.F.);
#13418=ORIENTED_EDGE('',*,*,#9804,.T.);
#13419=ORIENTED_EDGE('',*,*,#9682,.F.);
#13420=ORIENTED_EDGE('',*,*,#9804,.F.);
#13421=ORIENTED_EDGE('',*,*,#9805,.F.);
#13422=ORIENTED_EDGE('',*,*,#9806,.F.);
#13423=ORIENTED_EDGE('',*,*,#9683,.F.);
#13424=ORIENTED_EDGE('',*,*,#9806,.T.);
#13425=ORIENTED_EDGE('',*,*,#9807,.F.);
#13426=ORIENTED_EDGE('',*,*,#9808,.F.);
#13427=ORIENTED_EDGE('',*,*,#9684,.F.);
#13428=ORIENTED_EDGE('',*,*,#9808,.T.);
#13429=ORIENTED_EDGE('',*,*,#9809,.F.);
#13430=ORIENTED_EDGE('',*,*,#9810,.F.);
#13431=ORIENTED_EDGE('',*,*,#9685,.F.);
#13432=ORIENTED_EDGE('',*,*,#9810,.T.);
#13433=ORIENTED_EDGE('',*,*,#9811,.F.);
#13434=ORIENTED_EDGE('',*,*,#9812,.T.);
#13435=ORIENTED_EDGE('',*,*,#9686,.F.);
#13436=ORIENTED_EDGE('',*,*,#9812,.F.);
#13437=ORIENTED_EDGE('',*,*,#9813,.F.);
#13438=ORIENTED_EDGE('',*,*,#9814,.F.);
#13439=ORIENTED_EDGE('',*,*,#9687,.F.);
#13440=ORIENTED_EDGE('',*,*,#9814,.T.);
#13441=ORIENTED_EDGE('',*,*,#9815,.F.);
#13442=ORIENTED_EDGE('',*,*,#9816,.F.);
#13443=ORIENTED_EDGE('',*,*,#9688,.F.);
#13444=ORIENTED_EDGE('',*,*,#9816,.T.);
#13445=ORIENTED_EDGE('',*,*,#9817,.F.);
#13446=ORIENTED_EDGE('',*,*,#9818,.F.);
#13447=ORIENTED_EDGE('',*,*,#9689,.F.);
#13448=ORIENTED_EDGE('',*,*,#9818,.T.);
#13449=ORIENTED_EDGE('',*,*,#9819,.F.);
#13450=ORIENTED_EDGE('',*,*,#9820,.T.);
#13451=ORIENTED_EDGE('',*,*,#9690,.F.);
#13452=ORIENTED_EDGE('',*,*,#9820,.F.);
#13453=ORIENTED_EDGE('',*,*,#9821,.F.);
#13454=ORIENTED_EDGE('',*,*,#9822,.F.);
#13455=ORIENTED_EDGE('',*,*,#9691,.F.);
#13456=ORIENTED_EDGE('',*,*,#9822,.T.);
#13457=ORIENTED_EDGE('',*,*,#9823,.F.);
#13458=ORIENTED_EDGE('',*,*,#9824,.F.);
#13459=ORIENTED_EDGE('',*,*,#9692,.F.);
#13460=ORIENTED_EDGE('',*,*,#9824,.T.);
#13461=ORIENTED_EDGE('',*,*,#9825,.F.);
#13462=ORIENTED_EDGE('',*,*,#9826,.F.);
#13463=ORIENTED_EDGE('',*,*,#9693,.F.);
#13464=ORIENTED_EDGE('',*,*,#9826,.T.);
#13465=ORIENTED_EDGE('',*,*,#9827,.F.);
#13466=ORIENTED_EDGE('',*,*,#9828,.T.);
#13467=ORIENTED_EDGE('',*,*,#9694,.F.);
#13468=ORIENTED_EDGE('',*,*,#9828,.F.);
#13469=ORIENTED_EDGE('',*,*,#9829,.F.);
#13470=ORIENTED_EDGE('',*,*,#9830,.F.);
#13471=ORIENTED_EDGE('',*,*,#9695,.F.);
#13472=ORIENTED_EDGE('',*,*,#9830,.T.);
#13473=ORIENTED_EDGE('',*,*,#9831,.F.);
#13474=ORIENTED_EDGE('',*,*,#9832,.F.);
#13475=ORIENTED_EDGE('',*,*,#9696,.F.);
#13476=ORIENTED_EDGE('',*,*,#9832,.T.);
#13477=ORIENTED_EDGE('',*,*,#9833,.F.);
#13478=ORIENTED_EDGE('',*,*,#9834,.F.);
#13479=ORIENTED_EDGE('',*,*,#9697,.F.);
#13480=ORIENTED_EDGE('',*,*,#9834,.T.);
#13481=ORIENTED_EDGE('',*,*,#9835,.F.);
#13482=ORIENTED_EDGE('',*,*,#9836,.T.);
#13483=ORIENTED_EDGE('',*,*,#9698,.F.);
#13484=ORIENTED_EDGE('',*,*,#9836,.F.);
#13485=ORIENTED_EDGE('',*,*,#9837,.F.);
#13486=ORIENTED_EDGE('',*,*,#9838,.F.);
#13487=ORIENTED_EDGE('',*,*,#9699,.F.);
#13488=ORIENTED_EDGE('',*,*,#9838,.T.);
#13489=ORIENTED_EDGE('',*,*,#9839,.F.);
#13490=ORIENTED_EDGE('',*,*,#9840,.F.);
#13491=ORIENTED_EDGE('',*,*,#9700,.F.);
#13492=ORIENTED_EDGE('',*,*,#9840,.T.);
#13493=ORIENTED_EDGE('',*,*,#9841,.F.);
#13494=ORIENTED_EDGE('',*,*,#9842,.F.);
#13495=ORIENTED_EDGE('',*,*,#9701,.F.);
#13496=ORIENTED_EDGE('',*,*,#9842,.T.);
#13497=ORIENTED_EDGE('',*,*,#9843,.F.);
#13498=ORIENTED_EDGE('',*,*,#9844,.T.);
#13499=ORIENTED_EDGE('',*,*,#9702,.F.);
#13500=ORIENTED_EDGE('',*,*,#9844,.F.);
#13501=ORIENTED_EDGE('',*,*,#9845,.F.);
#13502=ORIENTED_EDGE('',*,*,#9846,.F.);
#13503=ORIENTED_EDGE('',*,*,#9703,.F.);
#13504=ORIENTED_EDGE('',*,*,#9846,.T.);
#13505=ORIENTED_EDGE('',*,*,#9847,.F.);
#13506=ORIENTED_EDGE('',*,*,#9848,.F.);
#13507=ORIENTED_EDGE('',*,*,#9704,.F.);
#13508=ORIENTED_EDGE('',*,*,#9848,.T.);
#13509=ORIENTED_EDGE('',*,*,#9849,.F.);
#13510=ORIENTED_EDGE('',*,*,#9850,.F.);
#13511=ORIENTED_EDGE('',*,*,#9705,.F.);
#13512=ORIENTED_EDGE('',*,*,#9850,.T.);
#13513=ORIENTED_EDGE('',*,*,#9851,.F.);
#13514=ORIENTED_EDGE('',*,*,#9852,.T.);
#13515=ORIENTED_EDGE('',*,*,#9706,.F.);
#13516=ORIENTED_EDGE('',*,*,#9852,.F.);
#13517=ORIENTED_EDGE('',*,*,#9853,.F.);
#13518=ORIENTED_EDGE('',*,*,#9854,.F.);
#13519=ORIENTED_EDGE('',*,*,#9707,.F.);
#13520=ORIENTED_EDGE('',*,*,#9854,.T.);
#13521=ORIENTED_EDGE('',*,*,#9855,.F.);
#13522=ORIENTED_EDGE('',*,*,#9856,.F.);
#13523=ORIENTED_EDGE('',*,*,#9708,.F.);
#13524=ORIENTED_EDGE('',*,*,#9856,.T.);
#13525=ORIENTED_EDGE('',*,*,#9857,.F.);
#13526=ORIENTED_EDGE('',*,*,#9858,.F.);
#13527=ORIENTED_EDGE('',*,*,#9709,.F.);
#13528=ORIENTED_EDGE('',*,*,#9858,.T.);
#13529=ORIENTED_EDGE('',*,*,#9859,.F.);
#13530=ORIENTED_EDGE('',*,*,#9860,.T.);
#13531=ORIENTED_EDGE('',*,*,#9710,.F.);
#13532=ORIENTED_EDGE('',*,*,#9860,.F.);
#13533=ORIENTED_EDGE('',*,*,#9861,.F.);
#13534=ORIENTED_EDGE('',*,*,#9862,.F.);
#13535=ORIENTED_EDGE('',*,*,#9711,.F.);
#13536=ORIENTED_EDGE('',*,*,#9862,.T.);
#13537=ORIENTED_EDGE('',*,*,#9863,.F.);
#13538=ORIENTED_EDGE('',*,*,#9864,.F.);
#13539=ORIENTED_EDGE('',*,*,#9712,.F.);
#13540=ORIENTED_EDGE('',*,*,#9864,.T.);
#13541=ORIENTED_EDGE('',*,*,#9865,.F.);
#13542=ORIENTED_EDGE('',*,*,#9866,.F.);
#13543=ORIENTED_EDGE('',*,*,#9713,.F.);
#13544=ORIENTED_EDGE('',*,*,#9866,.T.);
#13545=ORIENTED_EDGE('',*,*,#9867,.F.);
#13546=ORIENTED_EDGE('',*,*,#9868,.T.);
#13547=ORIENTED_EDGE('',*,*,#9714,.F.);
#13548=ORIENTED_EDGE('',*,*,#9868,.F.);
#13549=ORIENTED_EDGE('',*,*,#9869,.F.);
#13550=ORIENTED_EDGE('',*,*,#9870,.F.);
#13551=ORIENTED_EDGE('',*,*,#9715,.F.);
#13552=ORIENTED_EDGE('',*,*,#9870,.T.);
#13553=ORIENTED_EDGE('',*,*,#9871,.F.);
#13554=ORIENTED_EDGE('',*,*,#9872,.F.);
#13555=ORIENTED_EDGE('',*,*,#9716,.F.);
#13556=ORIENTED_EDGE('',*,*,#9872,.T.);
#13557=ORIENTED_EDGE('',*,*,#9873,.F.);
#13558=ORIENTED_EDGE('',*,*,#9874,.F.);
#13559=ORIENTED_EDGE('',*,*,#9717,.F.);
#13560=ORIENTED_EDGE('',*,*,#9874,.T.);
#13561=ORIENTED_EDGE('',*,*,#9875,.F.);
#13562=ORIENTED_EDGE('',*,*,#9876,.T.);
#13563=ORIENTED_EDGE('',*,*,#9718,.F.);
#13564=ORIENTED_EDGE('',*,*,#9876,.F.);
#13565=ORIENTED_EDGE('',*,*,#9877,.F.);
#13566=ORIENTED_EDGE('',*,*,#9878,.F.);
#13567=ORIENTED_EDGE('',*,*,#9719,.F.);
#13568=ORIENTED_EDGE('',*,*,#9878,.T.);
#13569=ORIENTED_EDGE('',*,*,#9879,.F.);
#13570=ORIENTED_EDGE('',*,*,#9880,.F.);
#13571=ORIENTED_EDGE('',*,*,#9720,.F.);
#13572=ORIENTED_EDGE('',*,*,#9880,.T.);
#13573=ORIENTED_EDGE('',*,*,#9881,.F.);
#13574=ORIENTED_EDGE('',*,*,#9882,.F.);
#13575=ORIENTED_EDGE('',*,*,#9721,.F.);
#13576=ORIENTED_EDGE('',*,*,#9882,.T.);
#13577=ORIENTED_EDGE('',*,*,#9883,.F.);
#13578=ORIENTED_EDGE('',*,*,#9884,.T.);
#13579=ORIENTED_EDGE('',*,*,#9722,.F.);
#13580=ORIENTED_EDGE('',*,*,#9884,.F.);
#13581=ORIENTED_EDGE('',*,*,#9885,.F.);
#13582=ORIENTED_EDGE('',*,*,#9886,.F.);
#13583=ORIENTED_EDGE('',*,*,#9723,.F.);
#13584=ORIENTED_EDGE('',*,*,#9886,.T.);
#13585=ORIENTED_EDGE('',*,*,#9887,.F.);
#13586=ORIENTED_EDGE('',*,*,#9888,.F.);
#13587=ORIENTED_EDGE('',*,*,#9724,.F.);
#13588=ORIENTED_EDGE('',*,*,#9888,.T.);
#13589=ORIENTED_EDGE('',*,*,#9889,.F.);
#13590=ORIENTED_EDGE('',*,*,#9890,.F.);
#13591=ORIENTED_EDGE('',*,*,#9725,.F.);
#13592=ORIENTED_EDGE('',*,*,#9891,.T.);
#13593=ORIENTED_EDGE('',*,*,#9889,.T.);
#13594=ORIENTED_EDGE('',*,*,#9887,.T.);
#13595=ORIENTED_EDGE('',*,*,#9885,.T.);
#13596=ORIENTED_EDGE('',*,*,#9883,.T.);
#13597=ORIENTED_EDGE('',*,*,#9881,.T.);
#13598=ORIENTED_EDGE('',*,*,#9879,.T.);
#13599=ORIENTED_EDGE('',*,*,#9877,.T.);
#13600=ORIENTED_EDGE('',*,*,#9875,.T.);
#13601=ORIENTED_EDGE('',*,*,#9873,.T.);
#13602=ORIENTED_EDGE('',*,*,#9871,.T.);
#13603=ORIENTED_EDGE('',*,*,#9869,.T.);
#13604=ORIENTED_EDGE('',*,*,#9867,.T.);
#13605=ORIENTED_EDGE('',*,*,#9865,.T.);
#13606=ORIENTED_EDGE('',*,*,#9863,.T.);
#13607=ORIENTED_EDGE('',*,*,#9861,.T.);
#13608=ORIENTED_EDGE('',*,*,#9859,.T.);
#13609=ORIENTED_EDGE('',*,*,#9857,.T.);
#13610=ORIENTED_EDGE('',*,*,#9855,.T.);
#13611=ORIENTED_EDGE('',*,*,#9853,.T.);
#13612=ORIENTED_EDGE('',*,*,#9851,.T.);
#13613=ORIENTED_EDGE('',*,*,#9849,.T.);
#13614=ORIENTED_EDGE('',*,*,#9847,.T.);
#13615=ORIENTED_EDGE('',*,*,#9845,.T.);
#13616=ORIENTED_EDGE('',*,*,#9843,.T.);
#13617=ORIENTED_EDGE('',*,*,#9841,.T.);
#13618=ORIENTED_EDGE('',*,*,#9839,.T.);
#13619=ORIENTED_EDGE('',*,*,#9837,.T.);
#13620=ORIENTED_EDGE('',*,*,#9835,.T.);
#13621=ORIENTED_EDGE('',*,*,#9833,.T.);
#13622=ORIENTED_EDGE('',*,*,#9831,.T.);
#13623=ORIENTED_EDGE('',*,*,#9829,.T.);
#13624=ORIENTED_EDGE('',*,*,#9827,.T.);
#13625=ORIENTED_EDGE('',*,*,#9825,.T.);
#13626=ORIENTED_EDGE('',*,*,#9823,.T.);
#13627=ORIENTED_EDGE('',*,*,#9821,.T.);
#13628=ORIENTED_EDGE('',*,*,#9819,.T.);
#13629=ORIENTED_EDGE('',*,*,#9817,.T.);
#13630=ORIENTED_EDGE('',*,*,#9815,.T.);
#13631=ORIENTED_EDGE('',*,*,#9813,.T.);
#13632=ORIENTED_EDGE('',*,*,#9811,.T.);
#13633=ORIENTED_EDGE('',*,*,#9809,.T.);
#13634=ORIENTED_EDGE('',*,*,#9807,.T.);
#13635=ORIENTED_EDGE('',*,*,#9805,.T.);
#13636=ORIENTED_EDGE('',*,*,#9803,.T.);
#13637=ORIENTED_EDGE('',*,*,#9801,.T.);
#13638=ORIENTED_EDGE('',*,*,#9799,.T.);
#13639=ORIENTED_EDGE('',*,*,#9797,.T.);
#13640=ORIENTED_EDGE('',*,*,#9795,.T.);
#13641=ORIENTED_EDGE('',*,*,#9793,.T.);
#13642=ORIENTED_EDGE('',*,*,#9791,.T.);
#13643=ORIENTED_EDGE('',*,*,#9789,.T.);
#13644=ORIENTED_EDGE('',*,*,#9787,.T.);
#13645=ORIENTED_EDGE('',*,*,#9785,.T.);
#13646=ORIENTED_EDGE('',*,*,#9783,.T.);
#13647=ORIENTED_EDGE('',*,*,#9781,.T.);
#13648=ORIENTED_EDGE('',*,*,#9779,.T.);
#13649=ORIENTED_EDGE('',*,*,#9777,.T.);
#13650=ORIENTED_EDGE('',*,*,#9775,.T.);
#13651=ORIENTED_EDGE('',*,*,#9773,.T.);
#13652=ORIENTED_EDGE('',*,*,#9771,.T.);
#13653=ORIENTED_EDGE('',*,*,#9769,.T.);
#13654=ORIENTED_EDGE('',*,*,#9767,.T.);
#13655=ORIENTED_EDGE('',*,*,#9765,.T.);
#13656=ORIENTED_EDGE('',*,*,#9763,.T.);
#13657=ORIENTED_EDGE('',*,*,#9761,.T.);
#13658=ORIENTED_EDGE('',*,*,#9759,.T.);
#13659=ORIENTED_EDGE('',*,*,#9757,.T.);
#13660=ORIENTED_EDGE('',*,*,#9755,.T.);
#13661=ORIENTED_EDGE('',*,*,#9753,.T.);
#13662=ORIENTED_EDGE('',*,*,#9751,.T.);
#13663=ORIENTED_EDGE('',*,*,#9749,.T.);
#13664=ORIENTED_EDGE('',*,*,#9747,.T.);
#13665=ORIENTED_EDGE('',*,*,#9745,.T.);
#13666=ORIENTED_EDGE('',*,*,#9743,.T.);
#13667=ORIENTED_EDGE('',*,*,#9741,.T.);
#13668=ORIENTED_EDGE('',*,*,#9739,.T.);
#13669=ORIENTED_EDGE('',*,*,#9737,.T.);
#13670=ORIENTED_EDGE('',*,*,#9735,.T.);
#13671=ORIENTED_EDGE('',*,*,#9733,.T.);
#13672=ORIENTED_EDGE('',*,*,#9731,.T.);
#13673=ORIENTED_EDGE('',*,*,#9732,.T.);
#13674=ORIENTED_EDGE('',*,*,#9726,.F.);
#13675=ORIENTED_EDGE('',*,*,#9890,.T.);
#13676=ORIENTED_EDGE('',*,*,#9891,.F.);
#15129=CYLINDRICAL_SURFACE('',#18051,1.);
#15130=CYLINDRICAL_SURFACE('',#18074,1.4);
#15131=CYLINDRICAL_SURFACE('',#18077,1.75);
#15132=CYLINDRICAL_SURFACE('',#18080,1.75);
#15133=CYLINDRICAL_SURFACE('',#18083,1.75);
#15134=CYLINDRICAL_SURFACE('',#18086,1.75);
#15135=CYLINDRICAL_SURFACE('',#18089,1.75);
#15136=CYLINDRICAL_SURFACE('',#18092,1.75);
#15137=CYLINDRICAL_SURFACE('',#18095,1.75);
#15138=CYLINDRICAL_SURFACE('',#18098,1.75);
#15139=CYLINDRICAL_SURFACE('',#18101,1.75);
#15140=CYLINDRICAL_SURFACE('',#18104,1.75);
#15141=CYLINDRICAL_SURFACE('',#18107,1.75);
#15142=CYLINDRICAL_SURFACE('',#18110,1.75);
#15143=CYLINDRICAL_SURFACE('',#18113,1.75);
#15144=CYLINDRICAL_SURFACE('',#18116,1.75);
#15145=CYLINDRICAL_SURFACE('',#18119,1.75);
#15146=CYLINDRICAL_SURFACE('',#18122,1.75);
#15147=CYLINDRICAL_SURFACE('',#18125,1.75);
#15148=CYLINDRICAL_SURFACE('',#18128,1.75);
#15149=CYLINDRICAL_SURFACE('',#18131,1.75);
#15150=CYLINDRICAL_SURFACE('',#18136,1.75);
#15806=ADVANCED_FACE('',(#2599),#1888,.F.);
#15807=ADVANCED_FACE('',(#2600),#1889,.F.);
#15808=ADVANCED_FACE('',(#2601),#1890,.F.);
#15809=ADVANCED_FACE('',(#2602,#1578),#1891,.T.);
#15810=ADVANCED_FACE('',(#2603),#15129,.F.);
#15811=ADVANCED_FACE('',(#2604,#1579),#1892,.F.);
#15812=ADVANCED_FACE('',(#2605),#15130,.T.);
#15813=ADVANCED_FACE('',(#2606),#51,.T.);
#15814=ADVANCED_FACE('',(#2607),#1893,.T.);
#15815=ADVANCED_FACE('',(#2608),#52,.T.);
#15816=ADVANCED_FACE('',(#2609),#15131,.T.);
#15817=ADVANCED_FACE('',(#2610),#53,.T.);
#15818=ADVANCED_FACE('',(#2611),#1894,.T.);
#15819=ADVANCED_FACE('',(#2612),#54,.T.);
#15820=ADVANCED_FACE('',(#2613),#15132,.T.);
#15821=ADVANCED_FACE('',(#2614),#55,.T.);
#15822=ADVANCED_FACE('',(#2615),#1895,.T.);
#15823=ADVANCED_FACE('',(#2616),#56,.T.);
#15824=ADVANCED_FACE('',(#2617),#15133,.T.);
#15825=ADVANCED_FACE('',(#2618),#57,.T.);
#15826=ADVANCED_FACE('',(#2619),#1896,.T.);
#15827=ADVANCED_FACE('',(#2620),#58,.T.);
#15828=ADVANCED_FACE('',(#2621),#15134,.T.);
#15829=ADVANCED_FACE('',(#2622),#59,.T.);
#15830=ADVANCED_FACE('',(#2623),#1897,.T.);
#15831=ADVANCED_FACE('',(#2624),#60,.T.);
#15832=ADVANCED_FACE('',(#2625),#15135,.T.);
#15833=ADVANCED_FACE('',(#2626),#61,.T.);
#15834=ADVANCED_FACE('',(#2627),#1898,.T.);
#15835=ADVANCED_FACE('',(#2628),#62,.T.);
#15836=ADVANCED_FACE('',(#2629),#15136,.T.);
#15837=ADVANCED_FACE('',(#2630),#63,.T.);
#15838=ADVANCED_FACE('',(#2631),#1899,.T.);
#15839=ADVANCED_FACE('',(#2632),#64,.T.);
#15840=ADVANCED_FACE('',(#2633),#15137,.T.);
#15841=ADVANCED_FACE('',(#2634),#65,.T.);
#15842=ADVANCED_FACE('',(#2635),#1900,.T.);
#15843=ADVANCED_FACE('',(#2636),#66,.T.);
#15844=ADVANCED_FACE('',(#2637),#15138,.T.);
#15845=ADVANCED_FACE('',(#2638),#67,.T.);
#15846=ADVANCED_FACE('',(#2639),#1901,.T.);
#15847=ADVANCED_FACE('',(#2640),#68,.T.);
#15848=ADVANCED_FACE('',(#2641),#15139,.T.);
#15849=ADVANCED_FACE('',(#2642),#69,.T.);
#15850=ADVANCED_FACE('',(#2643),#1902,.T.);
#15851=ADVANCED_FACE('',(#2644),#70,.T.);
#15852=ADVANCED_FACE('',(#2645),#15140,.T.);
#15853=ADVANCED_FACE('',(#2646),#71,.T.);
#15854=ADVANCED_FACE('',(#2647),#1903,.T.);
#15855=ADVANCED_FACE('',(#2648),#72,.T.);
#15856=ADVANCED_FACE('',(#2649),#15141,.T.);
#15857=ADVANCED_FACE('',(#2650),#73,.T.);
#15858=ADVANCED_FACE('',(#2651),#1904,.T.);
#15859=ADVANCED_FACE('',(#2652),#74,.T.);
#15860=ADVANCED_FACE('',(#2653),#15142,.T.);
#15861=ADVANCED_FACE('',(#2654),#75,.T.);
#15862=ADVANCED_FACE('',(#2655),#1905,.T.);
#15863=ADVANCED_FACE('',(#2656),#76,.T.);
#15864=ADVANCED_FACE('',(#2657),#15143,.T.);
#15865=ADVANCED_FACE('',(#2658),#77,.T.);
#15866=ADVANCED_FACE('',(#2659),#1906,.T.);
#15867=ADVANCED_FACE('',(#2660),#78,.T.);
#15868=ADVANCED_FACE('',(#2661),#15144,.T.);
#15869=ADVANCED_FACE('',(#2662),#79,.T.);
#15870=ADVANCED_FACE('',(#2663),#1907,.T.);
#15871=ADVANCED_FACE('',(#2664),#80,.T.);
#15872=ADVANCED_FACE('',(#2665),#15145,.T.);
#15873=ADVANCED_FACE('',(#2666),#81,.T.);
#15874=ADVANCED_FACE('',(#2667),#1908,.T.);
#15875=ADVANCED_FACE('',(#2668),#82,.T.);
#15876=ADVANCED_FACE('',(#2669),#15146,.T.);
#15877=ADVANCED_FACE('',(#2670),#83,.T.);
#15878=ADVANCED_FACE('',(#2671),#1909,.T.);
#15879=ADVANCED_FACE('',(#2672),#84,.T.);
#15880=ADVANCED_FACE('',(#2673),#15147,.T.);
#15881=ADVANCED_FACE('',(#2674),#85,.T.);
#15882=ADVANCED_FACE('',(#2675),#1910,.T.);
#15883=ADVANCED_FACE('',(#2676),#86,.T.);
#15884=ADVANCED_FACE('',(#2677),#15148,.T.);
#15885=ADVANCED_FACE('',(#2678),#87,.T.);
#15886=ADVANCED_FACE('',(#2679),#1911,.T.);
#15887=ADVANCED_FACE('',(#2680),#88,.T.);
#15888=ADVANCED_FACE('',(#2681),#15149,.T.);
#15889=ADVANCED_FACE('',(#2682),#89,.T.);
#15890=ADVANCED_FACE('',(#2683),#1912,.T.);
#15891=ADVANCED_FACE('',(#2684),#90,.T.);
#15892=ADVANCED_FACE('',(#2685,#1580),#1913,.T.);
#15893=ADVANCED_FACE('',(#2686),#15150,.T.);
#16184=CLOSED_SHELL('',(#15806,#15807,#15808,#15809,#15810,#15811,#15812,
#15813,#15814,#15815,#15816,#15817,#15818,#15819,#15820,#15821,#15822,#15823,
#15824,#15825,#15826,#15827,#15828,#15829,#15830,#15831,#15832,#15833,#15834,
#15835,#15836,#15837,#15838,#15839,#15840,#15841,#15842,#15843,#15844,#15845,
#15846,#15847,#15848,#15849,#15850,#15851,#15852,#15853,#15854,#15855,#15856,
#15857,#15858,#15859,#15860,#15861,#15862,#15863,#15864,#15865,#15866,#15867,
#15868,#15869,#15870,#15871,#15872,#15873,#15874,#15875,#15876,#15877,#15878,
#15879,#15880,#15881,#15882,#15883,#15884,#15885,#15886,#15887,#15888,#15889,
#15890,#15891,#15892,#15893));
#18044=AXIS2_PLACEMENT_3D('',#37661,#21570,#21571);
#18045=AXIS2_PLACEMENT_3D('',#37662,#21572,#21573);
#18046=AXIS2_PLACEMENT_3D('',#37671,#21578,#21579);
#18047=AXIS2_PLACEMENT_3D('',#37677,#21583,#21584);
#18048=AXIS2_PLACEMENT_3D('',#37683,#21588,#21589);
#18049=AXIS2_PLACEMENT_3D('',#37685,#21590,#21591);
#18050=AXIS2_PLACEMENT_3D('',#37686,#21592,#21593);
#18051=AXIS2_PLACEMENT_3D('',#37687,#21594,#21595);
#18052=AXIS2_PLACEMENT_3D('',#37688,#21596,#21597);
#18053=AXIS2_PLACEMENT_3D('',#37689,#21598,#21599);
#18054=AXIS2_PLACEMENT_3D('',#37692,#21600,#21601);
#18055=AXIS2_PLACEMENT_3D('',#37838,#21603,#21604);
#18056=AXIS2_PLACEMENT_3D('',#37984,#21606,#21607);
#18057=AXIS2_PLACEMENT_3D('',#38130,#21609,#21610);
#18058=AXIS2_PLACEMENT_3D('',#38276,#21612,#21613);
#18059=AXIS2_PLACEMENT_3D('',#38422,#21615,#21616);
#18060=AXIS2_PLACEMENT_3D('',#38568,#21618,#21619);
#18061=AXIS2_PLACEMENT_3D('',#38714,#21621,#21622);
#18062=AXIS2_PLACEMENT_3D('',#38860,#21624,#21625);
#18063=AXIS2_PLACEMENT_3D('',#39006,#21627,#21628);
#18064=AXIS2_PLACEMENT_3D('',#39152,#21630,#21631);
#18065=AXIS2_PLACEMENT_3D('',#39298,#21633,#21634);
#18066=AXIS2_PLACEMENT_3D('',#39444,#21636,#21637);
#18067=AXIS2_PLACEMENT_3D('',#39590,#21639,#21640);
#18068=AXIS2_PLACEMENT_3D('',#39736,#21642,#21643);
#18069=AXIS2_PLACEMENT_3D('',#39882,#21645,#21646);
#18070=AXIS2_PLACEMENT_3D('',#40028,#21648,#21649);
#18071=AXIS2_PLACEMENT_3D('',#40174,#21651,#21652);
#18072=AXIS2_PLACEMENT_3D('',#40320,#21654,#21655);
#18073=AXIS2_PLACEMENT_3D('',#40466,#21657,#21658);
#18074=AXIS2_PLACEMENT_3D('',#40610,#21660,#21661);
#18075=AXIS2_PLACEMENT_3D('',#40613,#21663,#21664);
#18076=AXIS2_PLACEMENT_3D('',#40828,#21667,#21668);
#18077=AXIS2_PLACEMENT_3D('',#41044,#21672,#21673);
#18078=AXIS2_PLACEMENT_3D('',#41046,#21674,#21675);
#18079=AXIS2_PLACEMENT_3D('',#41260,#21678,#21679);
#18080=AXIS2_PLACEMENT_3D('',#41476,#21683,#21684);
#18081=AXIS2_PLACEMENT_3D('',#41478,#21685,#21686);
#18082=AXIS2_PLACEMENT_3D('',#41692,#21689,#21690);
#18083=AXIS2_PLACEMENT_3D('',#41908,#21694,#21695);
#18084=AXIS2_PLACEMENT_3D('',#41910,#21696,#21697);
#18085=AXIS2_PLACEMENT_3D('',#42124,#21700,#21701);
#18086=AXIS2_PLACEMENT_3D('',#42340,#21705,#21706);
#18087=AXIS2_PLACEMENT_3D('',#42342,#21707,#21708);
#18088=AXIS2_PLACEMENT_3D('',#42556,#21711,#21712);
#18089=AXIS2_PLACEMENT_3D('',#42772,#21716,#21717);
#18090=AXIS2_PLACEMENT_3D('',#42774,#21718,#21719);
#18091=AXIS2_PLACEMENT_3D('',#42988,#21722,#21723);
#18092=AXIS2_PLACEMENT_3D('',#43204,#21727,#21728);
#18093=AXIS2_PLACEMENT_3D('',#43206,#21729,#21730);
#18094=AXIS2_PLACEMENT_3D('',#43420,#21733,#21734);
#18095=AXIS2_PLACEMENT_3D('',#43636,#21738,#21739);
#18096=AXIS2_PLACEMENT_3D('',#43638,#21740,#21741);
#18097=AXIS2_PLACEMENT_3D('',#43852,#21744,#21745);
#18098=AXIS2_PLACEMENT_3D('',#44068,#21749,#21750);
#18099=AXIS2_PLACEMENT_3D('',#44070,#21751,#21752);
#18100=AXIS2_PLACEMENT_3D('',#44284,#21755,#21756);
#18101=AXIS2_PLACEMENT_3D('',#44500,#21760,#21761);
#18102=AXIS2_PLACEMENT_3D('',#44502,#21762,#21763);
#18103=AXIS2_PLACEMENT_3D('',#44716,#21766,#21767);
#18104=AXIS2_PLACEMENT_3D('',#44932,#21771,#21772);
#18105=AXIS2_PLACEMENT_3D('',#44934,#21773,#21774);
#18106=AXIS2_PLACEMENT_3D('',#45148,#21777,#21778);
#18107=AXIS2_PLACEMENT_3D('',#45364,#21782,#21783);
#18108=AXIS2_PLACEMENT_3D('',#45366,#21784,#21785);
#18109=AXIS2_PLACEMENT_3D('',#45580,#21788,#21789);
#18110=AXIS2_PLACEMENT_3D('',#45796,#21793,#21794);
#18111=AXIS2_PLACEMENT_3D('',#45798,#21795,#21796);
#18112=AXIS2_PLACEMENT_3D('',#46012,#21799,#21800);
#18113=AXIS2_PLACEMENT_3D('',#46228,#21804,#21805);
#18114=AXIS2_PLACEMENT_3D('',#46230,#21806,#21807);
#18115=AXIS2_PLACEMENT_3D('',#46444,#21810,#21811);
#18116=AXIS2_PLACEMENT_3D('',#46660,#21815,#21816);
#18117=AXIS2_PLACEMENT_3D('',#46662,#21817,#21818);
#18118=AXIS2_PLACEMENT_3D('',#46876,#21821,#21822);
#18119=AXIS2_PLACEMENT_3D('',#47092,#21826,#21827);
#18120=AXIS2_PLACEMENT_3D('',#47094,#21828,#21829);
#18121=AXIS2_PLACEMENT_3D('',#47308,#21832,#21833);
#18122=AXIS2_PLACEMENT_3D('',#47524,#21837,#21838);
#18123=AXIS2_PLACEMENT_3D('',#47526,#21839,#21840);
#18124=AXIS2_PLACEMENT_3D('',#47740,#21843,#21844);
#18125=AXIS2_PLACEMENT_3D('',#47956,#21848,#21849);
#18126=AXIS2_PLACEMENT_3D('',#47958,#21850,#21851);
#18127=AXIS2_PLACEMENT_3D('',#48172,#21854,#21855);
#18128=AXIS2_PLACEMENT_3D('',#48388,#21859,#21860);
#18129=AXIS2_PLACEMENT_3D('',#48390,#21861,#21862);
#18130=AXIS2_PLACEMENT_3D('',#48604,#21865,#21866);
#18131=AXIS2_PLACEMENT_3D('',#48820,#21870,#21871);
#18132=AXIS2_PLACEMENT_3D('',#48822,#21872,#21873);
#18133=AXIS2_PLACEMENT_3D('',#49036,#21876,#21877);
#18134=AXIS2_PLACEMENT_3D('',#49252,#21881,#21882);
#18135=AXIS2_PLACEMENT_3D('',#49253,#21883,#21884);
#18136=AXIS2_PLACEMENT_3D('',#49254,#21885,#21886);
#21570=DIRECTION('axis',(0.,0.,1.));
#21571=DIRECTION('refdir',(1.,0.,0.));
#21572=DIRECTION('center_axis',(-1.,0.,0.));
#21573=DIRECTION('ref_axis',(0.,0.,1.));
#21574=DIRECTION('',(0.,0.,1.));
#21575=DIRECTION('',(0.,1.,0.));
#21576=DIRECTION('',(0.,0.,-1.));
#21577=DIRECTION('',(0.,1.,0.));
#21578=DIRECTION('center_axis',(0.,0.,-1.));
#21579=DIRECTION('ref_axis',(-1.,0.,0.));
#21580=DIRECTION('',(-1.,0.,0.));
#21581=DIRECTION('',(0.,1.,0.));
#21582=DIRECTION('',(1.,0.,0.));
#21583=DIRECTION('center_axis',(1.,0.,0.));
#21584=DIRECTION('ref_axis',(0.,0.,-1.));
#21585=DIRECTION('',(0.,0.,-1.));
#21586=DIRECTION('',(0.,-1.,0.));
#21587=DIRECTION('',(0.,0.,1.));
#21588=DIRECTION('center_axis',(0.,1.,0.));
#21589=DIRECTION('ref_axis',(1.,0.,0.));
#21590=DIRECTION('center_axis',(0.,1.,0.));
#21591=DIRECTION('ref_axis',(1.,0.,0.));
#21592=DIRECTION('center_axis',(0.,-1.,0.));
#21593=DIRECTION('ref_axis',(1.,0.,0.));
#21594=DIRECTION('center_axis',(0.,1.,0.));
#21595=DIRECTION('ref_axis',(-1.83697019872103E-16,0.,1.));
#21596=DIRECTION('center_axis',(0.,1.,0.));
#21597=DIRECTION('ref_axis',(1.,0.,0.));
#21598=DIRECTION('center_axis',(0.,1.,0.));
#21599=DIRECTION('ref_axis',(1.,0.,0.));
#21600=DIRECTION('center_axis',(0.,-1.,0.));
#21601=DIRECTION('ref_axis',(1.,0.,0.));
#21602=DIRECTION('',(-0.587785252292473,0.,0.809016994374947));
#21603=DIRECTION('center_axis',(0.,-1.,0.));
#21604=DIRECTION('ref_axis',(1.,0.,0.));
#21605=DIRECTION('',(-0.809016994374948,0.,0.587785252292473));
#21606=DIRECTION('center_axis',(0.,-1.,0.));
#21607=DIRECTION('ref_axis',(1.,0.,0.));
#21608=DIRECTION('',(-0.951056516295154,0.,0.309016994374947));
#21609=DIRECTION('center_axis',(0.,-1.,0.));
#21610=DIRECTION('ref_axis',(1.,0.,0.));
#21611=DIRECTION('',(-1.,0.,-1.83697019872103E-16));
#21612=DIRECTION('center_axis',(0.,-1.,0.));
#21613=DIRECTION('ref_axis',(1.,0.,0.));
#21614=DIRECTION('',(-0.951056516295154,0.,-0.309016994374948));
#21615=DIRECTION('center_axis',(0.,-1.,0.));
#21616=DIRECTION('ref_axis',(1.,0.,0.));
#21617=DIRECTION('',(-0.809016994374947,0.,-0.587785252292473));
#21618=DIRECTION('center_axis',(0.,-1.,0.));
#21619=DIRECTION('ref_axis',(1.,0.,0.));
#21620=DIRECTION('',(-0.587785252292473,0.,-0.809016994374948));
#21621=DIRECTION('center_axis',(0.,-1.,0.));
#21622=DIRECTION('ref_axis',(1.,0.,0.));
#21623=DIRECTION('',(-0.309016994374947,0.,-0.951056516295154));
#21624=DIRECTION('center_axis',(0.,-1.,0.));
#21625=DIRECTION('ref_axis',(1.,0.,0.));
#21626=DIRECTION('',(1.22464679914735E-16,0.,-1.));
#21627=DIRECTION('center_axis',(0.,-1.,0.));
#21628=DIRECTION('ref_axis',(1.,0.,0.));
#21629=DIRECTION('',(0.309016994374948,0.,-0.951056516295154));
#21630=DIRECTION('center_axis',(0.,-1.,0.));
#21631=DIRECTION('ref_axis',(1.,0.,0.));
#21632=DIRECTION('',(0.587785252292473,0.,-0.809016994374947));
#21633=DIRECTION('center_axis',(0.,-1.,0.));
#21634=DIRECTION('ref_axis',(1.,0.,0.));
#21635=DIRECTION('',(0.809016994374948,0.,-0.587785252292473));
#21636=DIRECTION('center_axis',(0.,-1.,0.));
#21637=DIRECTION('ref_axis',(1.,0.,0.));
#21638=DIRECTION('',(0.951056516295154,0.,-0.309016994374947));
#21639=DIRECTION('center_axis',(0.,-1.,0.));
#21640=DIRECTION('ref_axis',(1.,0.,0.));
#21641=DIRECTION('',(1.,0.,6.12323399573677E-17));
#21642=DIRECTION('center_axis',(0.,-1.,0.));
#21643=DIRECTION('ref_axis',(1.,0.,0.));
#21644=DIRECTION('',(0.951056516295154,0.,0.309016994374948));
#21645=DIRECTION('center_axis',(0.,-1.,0.));
#21646=DIRECTION('ref_axis',(1.,0.,0.));
#21647=DIRECTION('',(0.809016994374947,0.,0.587785252292473));
#21648=DIRECTION('center_axis',(0.,-1.,0.));
#21649=DIRECTION('ref_axis',(1.,0.,0.));
#21650=DIRECTION('',(0.587785252292473,0.,0.809016994374947));
#21651=DIRECTION('center_axis',(0.,-1.,0.));
#21652=DIRECTION('ref_axis',(1.,0.,0.));
#21653=DIRECTION('',(0.309016994374947,0.,0.951056516295154));
#21654=DIRECTION('center_axis',(0.,-1.,0.));
#21655=DIRECTION('ref_axis',(1.,0.,0.));
#21656=DIRECTION('',(0.,0.,1.));
#21657=DIRECTION('center_axis',(0.,-1.,0.));
#21658=DIRECTION('ref_axis',(1.,0.,0.));
#21659=DIRECTION('',(-0.309016994374948,0.,0.951056516295154));
#21660=DIRECTION('center_axis',(0.,1.,0.));
#21661=DIRECTION('ref_axis',(1.,0.,0.));
#21662=DIRECTION('',(0.,-1.,0.));
#21663=DIRECTION('center_axis',(0.,-1.,0.));
#21664=DIRECTION('ref_axis',(1.,0.,0.));
#21665=DIRECTION('',(0.,-1.,0.));
#21666=DIRECTION('',(0.,1.,0.));
#21667=DIRECTION('center_axis',(0.951056516295154,0.,0.309016994374948));
#21668=DIRECTION('ref_axis',(0.309016994374948,0.,-0.951056516295154));
#21669=DIRECTION('',(0.309016994374948,0.,-0.951056516295154));
#21670=DIRECTION('',(0.,1.,0.));
#21671=DIRECTION('',(0.,1.,0.));
#21672=DIRECTION('center_axis',(0.,1.,0.));
#21673=DIRECTION('ref_axis',(1.,0.,0.));
#21674=DIRECTION('center_axis',(0.,1.,0.));
#21675=DIRECTION('ref_axis',(1.,0.,0.));
#21676=DIRECTION('',(0.,-1.,0.));
#21677=DIRECTION('',(0.,1.,0.));
#21678=DIRECTION('center_axis',(0.809016994374947,0.,0.587785252292473));
#21679=DIRECTION('ref_axis',(0.587785252292473,0.,-0.809016994374947));
#21680=DIRECTION('',(0.587785252292473,0.,-0.809016994374947));
#21681=DIRECTION('',(0.,1.,0.));
#21682=DIRECTION('',(0.,1.,0.));
#21683=DIRECTION('center_axis',(0.,1.,0.));
#21684=DIRECTION('ref_axis',(1.,0.,0.));
#21685=DIRECTION('center_axis',(0.,1.,0.));
#21686=DIRECTION('ref_axis',(1.,0.,0.));
#21687=DIRECTION('',(0.,-1.,0.));
#21688=DIRECTION('',(0.,1.,0.));
#21689=DIRECTION('center_axis',(0.587785252292473,0.,0.809016994374948));
#21690=DIRECTION('ref_axis',(0.809016994374948,0.,-0.587785252292473));
#21691=DIRECTION('',(0.809016994374948,0.,-0.587785252292473));
#21692=DIRECTION('',(0.,1.,0.));
#21693=DIRECTION('',(0.,1.,0.));
#21694=DIRECTION('center_axis',(0.,1.,0.));
#21695=DIRECTION('ref_axis',(1.,0.,0.));
#21696=DIRECTION('center_axis',(0.,1.,0.));
#21697=DIRECTION('ref_axis',(1.,0.,0.));
#21698=DIRECTION('',(0.,-1.,0.));
#21699=DIRECTION('',(0.,1.,0.));
#21700=DIRECTION('center_axis',(0.309016994374947,0.,0.951056516295154));
#21701=DIRECTION('ref_axis',(0.951056516295154,0.,-0.309016994374947));
#21702=DIRECTION('',(0.951056516295154,0.,-0.309016994374947));
#21703=DIRECTION('',(0.,1.,0.));
#21704=DIRECTION('',(0.,1.,0.));
#21705=DIRECTION('center_axis',(0.,1.,0.));
#21706=DIRECTION('ref_axis',(1.,0.,0.));
#21707=DIRECTION('center_axis',(0.,1.,0.));
#21708=DIRECTION('ref_axis',(1.,0.,0.));
#21709=DIRECTION('',(0.,-1.,0.));
#21710=DIRECTION('',(0.,1.,0.));
#21711=DIRECTION('center_axis',(-1.83697019872103E-16,0.,1.));
#21712=DIRECTION('ref_axis',(1.,0.,1.83697019872103E-16));
#21713=DIRECTION('',(1.,0.,1.83697019872103E-16));
#21714=DIRECTION('',(0.,1.,0.));
#21715=DIRECTION('',(0.,1.,0.));
#21716=DIRECTION('center_axis',(0.,1.,0.));
#21717=DIRECTION('ref_axis',(1.,0.,0.));
#21718=DIRECTION('center_axis',(0.,1.,0.));
#21719=DIRECTION('ref_axis',(1.,0.,0.));
#21720=DIRECTION('',(0.,-1.,0.));
#21721=DIRECTION('',(0.,1.,0.));
#21722=DIRECTION('center_axis',(-0.309016994374948,0.,0.951056516295154));
#21723=DIRECTION('ref_axis',(0.951056516295154,0.,0.309016994374948));
#21724=DIRECTION('',(0.951056516295154,0.,0.309016994374948));
#21725=DIRECTION('',(0.,1.,0.));
#21726=DIRECTION('',(0.,1.,0.));
#21727=DIRECTION('center_axis',(0.,1.,0.));
#21728=DIRECTION('ref_axis',(1.,0.,0.));
#21729=DIRECTION('center_axis',(0.,1.,0.));
#21730=DIRECTION('ref_axis',(1.,0.,0.));
#21731=DIRECTION('',(0.,-1.,0.));
#21732=DIRECTION('',(0.,1.,0.));
#21733=DIRECTION('center_axis',(-0.587785252292473,0.,0.809016994374947));
#21734=DIRECTION('ref_axis',(0.809016994374947,0.,0.587785252292473));
#21735=DIRECTION('',(0.809016994374947,0.,0.587785252292473));
#21736=DIRECTION('',(0.,1.,0.));
#21737=DIRECTION('',(0.,1.,0.));
#21738=DIRECTION('center_axis',(0.,1.,0.));
#21739=DIRECTION('ref_axis',(1.,0.,0.));
#21740=DIRECTION('center_axis',(0.,1.,0.));
#21741=DIRECTION('ref_axis',(1.,0.,0.));
#21742=DIRECTION('',(0.,-1.,0.));
#21743=DIRECTION('',(0.,1.,0.));
#21744=DIRECTION('center_axis',(-0.809016994374948,0.,0.587785252292473));
#21745=DIRECTION('ref_axis',(0.587785252292473,0.,0.809016994374948));
#21746=DIRECTION('',(0.587785252292473,0.,0.809016994374948));
#21747=DIRECTION('',(0.,1.,0.));
#21748=DIRECTION('',(0.,1.,0.));
#21749=DIRECTION('center_axis',(0.,1.,0.));
#21750=DIRECTION('ref_axis',(1.,0.,0.));
#21751=DIRECTION('center_axis',(0.,1.,0.));
#21752=DIRECTION('ref_axis',(1.,0.,0.));
#21753=DIRECTION('',(0.,-1.,0.));
#21754=DIRECTION('',(0.,1.,0.));
#21755=DIRECTION('center_axis',(-0.951056516295154,0.,0.309016994374947));
#21756=DIRECTION('ref_axis',(0.309016994374947,0.,0.951056516295154));
#21757=DIRECTION('',(0.309016994374947,0.,0.951056516295154));
#21758=DIRECTION('',(0.,1.,0.));
#21759=DIRECTION('',(0.,1.,0.));
#21760=DIRECTION('center_axis',(0.,1.,0.));
#21761=DIRECTION('ref_axis',(1.,0.,0.));
#21762=DIRECTION('center_axis',(0.,1.,0.));
#21763=DIRECTION('ref_axis',(1.,0.,0.));
#21764=DIRECTION('',(0.,-1.,0.));
#21765=DIRECTION('',(0.,1.,0.));
#21766=DIRECTION('center_axis',(-1.,0.,-1.22464679914735E-16));
#21767=DIRECTION('ref_axis',(-1.22464679914735E-16,0.,1.));
#21768=DIRECTION('',(-1.22464679914735E-16,0.,1.));
#21769=DIRECTION('',(0.,1.,0.));
#21770=DIRECTION('',(0.,1.,0.));
#21771=DIRECTION('center_axis',(0.,1.,0.));
#21772=DIRECTION('ref_axis',(1.,0.,0.));
#21773=DIRECTION('center_axis',(0.,1.,0.));
#21774=DIRECTION('ref_axis',(1.,0.,0.));
#21775=DIRECTION('',(0.,-1.,0.));
#21776=DIRECTION('',(0.,1.,0.));
#21777=DIRECTION('center_axis',(-0.951056516295154,0.,-0.309016994374948));
#21778=DIRECTION('ref_axis',(-0.309016994374948,0.,0.951056516295154));
#21779=DIRECTION('',(-0.309016994374948,0.,0.951056516295154));
#21780=DIRECTION('',(0.,1.,0.));
#21781=DIRECTION('',(0.,1.,0.));
#21782=DIRECTION('center_axis',(0.,1.,0.));
#21783=DIRECTION('ref_axis',(1.,0.,0.));
#21784=DIRECTION('center_axis',(0.,1.,0.));
#21785=DIRECTION('ref_axis',(1.,0.,0.));
#21786=DIRECTION('',(0.,-1.,0.));
#21787=DIRECTION('',(0.,1.,0.));
#21788=DIRECTION('center_axis',(-0.809016994374947,0.,-0.587785252292473));
#21789=DIRECTION('ref_axis',(-0.587785252292473,0.,0.809016994374947));
#21790=DIRECTION('',(-0.587785252292473,0.,0.809016994374947));
#21791=DIRECTION('',(0.,1.,0.));
#21792=DIRECTION('',(0.,1.,0.));
#21793=DIRECTION('center_axis',(0.,1.,0.));
#21794=DIRECTION('ref_axis',(1.,0.,0.));
#21795=DIRECTION('center_axis',(0.,1.,0.));
#21796=DIRECTION('ref_axis',(1.,0.,0.));
#21797=DIRECTION('',(0.,-1.,0.));
#21798=DIRECTION('',(0.,1.,0.));
#21799=DIRECTION('center_axis',(-0.587785252292473,0.,-0.809016994374948));
#21800=DIRECTION('ref_axis',(-0.809016994374948,0.,0.587785252292473));
#21801=DIRECTION('',(-0.809016994374948,0.,0.587785252292473));
#21802=DIRECTION('',(0.,1.,0.));
#21803=DIRECTION('',(0.,1.,0.));
#21804=DIRECTION('center_axis',(0.,1.,0.));
#21805=DIRECTION('ref_axis',(1.,0.,0.));
#21806=DIRECTION('center_axis',(0.,1.,0.));
#21807=DIRECTION('ref_axis',(1.,0.,0.));
#21808=DIRECTION('',(0.,-1.,0.));
#21809=DIRECTION('',(0.,1.,0.));
#21810=DIRECTION('center_axis',(-0.309016994374947,0.,-0.951056516295154));
#21811=DIRECTION('ref_axis',(-0.951056516295154,0.,0.309016994374947));
#21812=DIRECTION('',(-0.951056516295154,0.,0.309016994374947));
#21813=DIRECTION('',(0.,1.,0.));
#21814=DIRECTION('',(0.,1.,0.));
#21815=DIRECTION('center_axis',(0.,1.,0.));
#21816=DIRECTION('ref_axis',(1.,0.,0.));
#21817=DIRECTION('center_axis',(0.,1.,0.));
#21818=DIRECTION('ref_axis',(1.,0.,0.));
#21819=DIRECTION('',(0.,-1.,0.));
#21820=DIRECTION('',(0.,1.,0.));
#21821=DIRECTION('center_axis',(6.12323399573677E-17,0.,-1.));
#21822=DIRECTION('ref_axis',(-1.,0.,-6.12323399573677E-17));
#21823=DIRECTION('',(-1.,0.,-6.12323399573677E-17));
#21824=DIRECTION('',(0.,1.,0.));
#21825=DIRECTION('',(0.,1.,0.));
#21826=DIRECTION('center_axis',(0.,1.,0.));
#21827=DIRECTION('ref_axis',(1.,0.,0.));
#21828=DIRECTION('center_axis',(0.,1.,0.));
#21829=DIRECTION('ref_axis',(1.,0.,0.));
#21830=DIRECTION('',(0.,-1.,0.));
#21831=DIRECTION('',(0.,1.,0.));
#21832=DIRECTION('center_axis',(0.309016994374948,0.,-0.951056516295154));
#21833=DIRECTION('ref_axis',(-0.951056516295154,0.,-0.309016994374948));
#21834=DIRECTION('',(-0.951056516295154,0.,-0.309016994374948));
#21835=DIRECTION('',(0.,1.,0.));
#21836=DIRECTION('',(0.,1.,0.));
#21837=DIRECTION('center_axis',(0.,1.,0.));
#21838=DIRECTION('ref_axis',(1.,0.,0.));
#21839=DIRECTION('center_axis',(0.,1.,0.));
#21840=DIRECTION('ref_axis',(1.,0.,0.));
#21841=DIRECTION('',(0.,-1.,0.));
#21842=DIRECTION('',(0.,1.,0.));
#21843=DIRECTION('center_axis',(0.587785252292473,0.,-0.809016994374947));
#21844=DIRECTION('ref_axis',(-0.809016994374947,0.,-0.587785252292473));
#21845=DIRECTION('',(-0.809016994374947,0.,-0.587785252292473));
#21846=DIRECTION('',(0.,1.,0.));
#21847=DIRECTION('',(0.,1.,0.));
#21848=DIRECTION('center_axis',(0.,1.,0.));
#21849=DIRECTION('ref_axis',(1.,0.,0.));
#21850=DIRECTION('center_axis',(0.,1.,0.));
#21851=DIRECTION('ref_axis',(1.,0.,0.));
#21852=DIRECTION('',(0.,-1.,0.));
#21853=DIRECTION('',(0.,1.,0.));
#21854=DIRECTION('center_axis',(0.809016994374947,0.,-0.587785252292473));
#21855=DIRECTION('ref_axis',(-0.587785252292473,0.,-0.809016994374947));
#21856=DIRECTION('',(-0.587785252292473,0.,-0.809016994374947));
#21857=DIRECTION('',(0.,1.,0.));
#21858=DIRECTION('',(0.,1.,0.));
#21859=DIRECTION('center_axis',(0.,1.,0.));
#21860=DIRECTION('ref_axis',(1.,0.,0.));
#21861=DIRECTION('center_axis',(0.,1.,0.));
#21862=DIRECTION('ref_axis',(1.,0.,0.));
#21863=DIRECTION('',(0.,-1.,0.));
#21864=DIRECTION('',(0.,1.,0.));
#21865=DIRECTION('center_axis',(0.951056516295154,0.,-0.309016994374947));
#21866=DIRECTION('ref_axis',(-0.309016994374947,0.,-0.951056516295154));
#21867=DIRECTION('',(-0.309016994374947,0.,-0.951056516295154));
#21868=DIRECTION('',(0.,1.,0.));
#21869=DIRECTION('',(0.,1.,0.));
#21870=DIRECTION('center_axis',(0.,1.,0.));
#21871=DIRECTION('ref_axis',(1.,0.,0.));
#21872=DIRECTION('center_axis',(0.,1.,0.));
#21873=DIRECTION('ref_axis',(1.,0.,0.));
#21874=DIRECTION('',(0.,-1.,0.));
#21875=DIRECTION('',(0.,1.,0.));
#21876=DIRECTION('center_axis',(1.,0.,0.));
#21877=DIRECTION('ref_axis',(0.,0.,-1.));
#21878=DIRECTION('',(0.,0.,-1.));
#21879=DIRECTION('',(0.,1.,0.));
#21880=DIRECTION('',(0.,1.,0.));
#21881=DIRECTION('center_axis',(0.,1.,0.));
#21882=DIRECTION('ref_axis',(1.,0.,0.));
#21883=DIRECTION('center_axis',(0.,1.,0.));
#21884=DIRECTION('ref_axis',(1.,0.,0.));
#21885=DIRECTION('center_axis',(0.,1.,0.));
#21886=DIRECTION('ref_axis',(1.,0.,0.));
#37661=CARTESIAN_POINT('',(0.,0.,0.));
#37662=CARTESIAN_POINT('Origin',(-0.3,-1.1,-1.28));
#37663=CARTESIAN_POINT('',(-0.3,-1.,-1.28));
#37664=CARTESIAN_POINT('',(-0.3,-1.,-0.953939201416946));
#37665=CARTESIAN_POINT('',(-0.3,-1.,-0.64));
#37666=CARTESIAN_POINT('',(-0.3,2.2,-1.28));
#37667=CARTESIAN_POINT('',(-0.3,-1.1,-1.28));
#37668=CARTESIAN_POINT('',(-0.3,2.2,-0.953939201416946));
#37669=CARTESIAN_POINT('',(-0.3,2.2,-0.64));
#37670=CARTESIAN_POINT('',(-0.3,-1.1,-0.953939201416946));
#37671=CARTESIAN_POINT('Origin',(0.3,-1.1,-1.28));
#37672=CARTESIAN_POINT('',(0.3,-1.,-1.28));
#37673=CARTESIAN_POINT('',(0.15,-1.,-1.28));
#37674=CARTESIAN_POINT('',(0.3,2.2,-1.28));
#37675=CARTESIAN_POINT('',(0.3,-1.1,-1.28));
#37676=CARTESIAN_POINT('',(0.15,2.2,-1.28));
#37677=CARTESIAN_POINT('Origin',(0.3,-1.1,0.));
#37678=CARTESIAN_POINT('',(0.3,-1.,-0.953939201416946));
#37679=CARTESIAN_POINT('',(0.3,-1.,0.));
#37680=CARTESIAN_POINT('',(0.3,2.2,-0.953939201416946));
#37681=CARTESIAN_POINT('',(0.3,-1.1,-0.953939201416946));
#37682=CARTESIAN_POINT('',(0.3,2.2,0.));
#37683=CARTESIAN_POINT('Origin',(0.,2.2,0.));
#37684=CARTESIAN_POINT('',(-1.4,2.2,1.71450551880629E-16));
#37685=CARTESIAN_POINT('Origin',(0.,2.2,0.));
#37686=CARTESIAN_POINT('Origin',(0.,2.2,0.));
#37687=CARTESIAN_POINT('Origin',(0.,-1.1,0.));
#37688=CARTESIAN_POINT('Origin',(0.,-1.,0.));
#37689=CARTESIAN_POINT('Origin',(0.,-1.,0.));
#37690=CARTESIAN_POINT('',(1.60662857109684,-1.,0.693717979106306));
#37691=CARTESIAN_POINT('',(1.5055822144029,-1.,0.892032620296856));
#37692=CARTESIAN_POINT('Origin',(0.,-1.,0.));
#37693=CARTESIAN_POINT('',(1.81978687191668,-1.,1.23627494547115));
#37694=CARTESIAN_POINT('Ctrl Pts',(1.5055822144029,-1.,0.892032620296856));
#37695=CARTESIAN_POINT('Ctrl Pts',(1.50980486806688,-1.,0.894452006964544));
#37696=CARTESIAN_POINT('Ctrl Pts',(1.51805569590094,-1.,0.899185047483511));
#37697=CARTESIAN_POINT('Ctrl Pts',(1.52984849887993,-1.,0.905967409625651));
#37698=CARTESIAN_POINT('Ctrl Pts',(1.54440491149498,-1.,0.914375919026456));
#37699=CARTESIAN_POINT('Ctrl Pts',(1.56065988578893,-1.,0.923832188944341));
#37700=CARTESIAN_POINT('Ctrl Pts',(1.57499388382243,-1.,0.932246680108685));
#37701=CARTESIAN_POINT('Ctrl Pts',(1.58744937487176,-1.,0.939646377893399));
#37702=CARTESIAN_POINT('Ctrl Pts',(1.59810042043673,-1.,0.946078063315257));
#37703=CARTESIAN_POINT('Ctrl Pts',(1.60706069896936,-1.,0.951613284356035));
#37704=CARTESIAN_POINT('Ctrl Pts',(1.61449324337085,-1.,0.956354422920671));
#37705=CARTESIAN_POINT('Ctrl Pts',(1.62061638140221,-1.,0.960438326101729));
#37706=CARTESIAN_POINT('Ctrl Pts',(1.62571930670187,-1.,0.964046107040536));
#37707=CARTESIAN_POINT('Ctrl Pts',(1.63013849959461,-1.,0.967387853230345));
#37708=CARTESIAN_POINT('Ctrl Pts',(1.63420665729798,-1.,0.970669715997509));
#37709=CARTESIAN_POINT('Ctrl Pts',(1.63820952658144,-1.,0.974066058287419));
#37710=CARTESIAN_POINT('Ctrl Pts',(1.64233990826687,-1.,0.977689794119417));
#37711=CARTESIAN_POINT('Ctrl Pts',(1.64665139190656,-1.,0.981562530939489));
#37712=CARTESIAN_POINT('Ctrl Pts',(1.65110016612638,-1.,0.985642622920821));
#37713=CARTESIAN_POINT('Ctrl Pts',(1.65559044289699,-1.,0.989855627854165));
#37714=CARTESIAN_POINT('Ctrl Pts',(1.66001553809947,-1.,0.994121836661306));
#37715=CARTESIAN_POINT('Ctrl Pts',(1.66430758030376,-1.,0.998389654952758));
#37716=CARTESIAN_POINT('Ctrl Pts',(1.66846059277303,-1.,1.00265091003727));
#37717=CARTESIAN_POINT('Ctrl Pts',(1.67250335383293,-1.,1.00692206696414));
#37718=CARTESIAN_POINT('Ctrl Pts',(1.67648246776464,-1.,1.01123236493511));
#37719=CARTESIAN_POINT('Ctrl Pts',(1.68044289894798,-1.,1.01561026162773));
#37720=CARTESIAN_POINT('Ctrl Pts',(1.68440578021706,-1.,1.02006795074201));
#37721=CARTESIAN_POINT('Ctrl Pts',(1.68836910178447,-1.,1.02460180535255));
#37722=CARTESIAN_POINT('Ctrl Pts',(1.69231840863458,-1.,1.02919977579147));
#37723=CARTESIAN_POINT('Ctrl Pts',(1.69623414782771,-1.,1.03384646003588));
#37724=CARTESIAN_POINT('Ctrl Pts',(1.70010052930962,-1.,1.03852922490789));
#37725=CARTESIAN_POINT('Ctrl Pts',(1.70391338707982,-1.,1.04324363334554));
#37726=CARTESIAN_POINT('Ctrl Pts',(1.70767646263649,-1.,1.04799085404995));
#37727=CARTESIAN_POINT('Ctrl Pts',(1.71139783543989,-1.,1.05277517202855));
#37728=CARTESIAN_POINT('Ctrl Pts',(1.7150865442702,-1.,1.05760163192479));
#37729=CARTESIAN_POINT('Ctrl Pts',(1.71874858456904,-1.,1.06247324680647));
#37730=CARTESIAN_POINT('Ctrl Pts',(1.72238500928453,-1.,1.06738966975462));
#37731=CARTESIAN_POINT('Ctrl Pts',(1.72599406198488,-1.,1.07234866990252));
#37732=CARTESIAN_POINT('Ctrl Pts',(1.72957248977424,-1.,1.0773470373727));
#37733=CARTESIAN_POINT('Ctrl Pts',(1.73311705663407,-1.,1.08238162784749));
#37734=CARTESIAN_POINT('Ctrl Pts',(1.73662628326091,-1.,1.08745056285427));
#37735=CARTESIAN_POINT('Ctrl Pts',(1.74010053962247,-1.,1.09255329056493));
#37736=CARTESIAN_POINT('Ctrl Pts',(1.74354119236208,-1.,1.09768999241226));
#37737=CARTESIAN_POINT('Ctrl Pts',(1.74695004214923,-1.,1.10286118991143));
#37738=CARTESIAN_POINT('Ctrl Pts',(1.7503286607592,-1.,1.10806728183007));
#37739=CARTESIAN_POINT('Ctrl Pts',(1.7536777209463,-1.,1.11330807582551));
#37740=CARTESIAN_POINT('Ctrl Pts',(1.75699720772105,-1.,1.11858293216763));
#37741=CARTESIAN_POINT('Ctrl Pts',(1.76028671825096,-1.,1.12389096855086));
#37742=CARTESIAN_POINT('Ctrl Pts',(1.7635457196617,-1.,1.12923123555075));
#37743=CARTESIAN_POINT('Ctrl Pts',(1.76677384551862,-1.,1.1346029180462));
#37744=CARTESIAN_POINT('Ctrl Pts',(1.76997111386769,-1.,1.14000548336975));
#37745=CARTESIAN_POINT('Ctrl Pts',(1.77313777896194,-1.,1.1454385822692));
#37746=CARTESIAN_POINT('Ctrl Pts',(1.7762742255701,-1.,1.15090197841515));
#37747=CARTESIAN_POINT('Ctrl Pts',(1.77938085564275,-1.,1.15639547194698));
#37748=CARTESIAN_POINT('Ctrl Pts',(1.78245795881009,-1.,1.16191881298499));
#37749=CARTESIAN_POINT('Ctrl Pts',(1.78550566040443,-1.,1.16747166312303));
#37750=CARTESIAN_POINT('Ctrl Pts',(1.78852398877616,-1.,1.17305363177328));
#37751=CARTESIAN_POINT('Ctrl Pts',(1.79151291552689,-1.,1.17866429440809));
#37752=CARTESIAN_POINT('Ctrl Pts',(1.79447240321515,-1.,1.18430321697432));
#37753=CARTESIAN_POINT('Ctrl Pts',(1.79740245923478,-1.,1.18996997934445));
#37754=CARTESIAN_POINT('Ctrl Pts',(1.80030314369879,-1.,1.19566418930242));
#37755=CARTESIAN_POINT('Ctrl Pts',(1.80317454838603,-1.,1.20138548938974));
#37756=CARTESIAN_POINT('Ctrl Pts',(1.80601678480707,-1.,1.20713356605475));
#37757=CARTESIAN_POINT('Ctrl Pts',(1.80882996917129,-1.,1.21290815708314));
#37758=CARTESIAN_POINT('Ctrl Pts',(1.81161420806656,-1.,1.21870906103557));
#37759=CARTESIAN_POINT('Ctrl Pts',(1.81436959210434,-1.,1.2245361330495));
#37760=CARTESIAN_POINT('Ctrl Pts',(1.8165508718364,-1.,1.2292186489137));
#37761=CARTESIAN_POINT('Ctrl Pts',(1.81817389921279,-1.,1.2327422452705));
#37762=CARTESIAN_POINT('Ctrl Pts',(1.81925017193666,-1.,1.23509651170476));
#37763=CARTESIAN_POINT('Ctrl Pts',(1.81978687191668,-1.,1.23627494547115));
#37764=CARTESIAN_POINT('',(1.73811241238545,-1.,1.34869019493419));
#37765=CARTESIAN_POINT('',(1.81978687191668,-1.,1.23627494547115));
#37766=CARTESIAN_POINT('',(1.31362392696032,-1.,1.15624053661742));
#37767=CARTESIAN_POINT('Ctrl Pts',(1.73811241238545,-1.,1.34869019493419));
#37768=CARTESIAN_POINT('Ctrl Pts',(1.73682580585691,-1.,1.34854391898045));
#37769=CARTESIAN_POINT('Ctrl Pts',(1.73425417885907,-1.,1.34824783112887));
#37770=CARTESIAN_POINT('Ctrl Pts',(1.7304014965394,-1.,1.34779309152035));
#37771=CARTESIAN_POINT('Ctrl Pts',(1.72527410680674,-1.,1.34716554819527));
#37772=CARTESIAN_POINT('Ctrl Pts',(1.7188807715049,-1.,1.34634568653227));
#37773=CARTESIAN_POINT('Ctrl Pts',(1.71250340686822,-1.,1.34549029589416));
#37774=CARTESIAN_POINT('Ctrl Pts',(1.70614212266738,-1.,1.34459924533831));
#37775=CARTESIAN_POINT('Ctrl Pts',(1.69979707754427,-1.,1.34367237124483));
#37776=CARTESIAN_POINT('Ctrl Pts',(1.6934684849687,-1.,1.34270948206319));
#37777=CARTESIAN_POINT('Ctrl Pts',(1.68715660868764,-1.,1.341710374848));
#37778=CARTESIAN_POINT('Ctrl Pts',(1.68086176030362,-1.,1.34067485185203));
#37779=CARTESIAN_POINT('Ctrl Pts',(1.67458429426086,-1.,1.3396027347034));
#37780=CARTESIAN_POINT('Ctrl Pts',(1.66832460783989,-1.,1.33849388654388));
#37781=CARTESIAN_POINT('Ctrl Pts',(1.66208312541983,-1.,1.33734820885262));
#37782=CARTESIAN_POINT('Ctrl Pts',(1.65586025952593,-1.,1.33616559745172));
#37783=CARTESIAN_POINT('Ctrl Pts',(1.6496563728683,-1.,1.33494590467993));
#37784=CARTESIAN_POINT('Ctrl Pts',(1.6434717485603,-1.,1.33368890676572));
#37785=CARTESIAN_POINT('Ctrl Pts',(1.63730653475089,-1.,1.33239425103724));
#37786=CARTESIAN_POINT('Ctrl Pts',(1.63116079730923,-1.,1.33106149345645));
#37787=CARTESIAN_POINT('Ctrl Pts',(1.62503464209797,-1.,1.3296901950568));
#37788=CARTESIAN_POINT('Ctrl Pts',(1.61892832270724,-1.,1.32828000610449));
#37789=CARTESIAN_POINT('Ctrl Pts',(1.6128423401575,-1.,1.32683074483356));
#37790=CARTESIAN_POINT('Ctrl Pts',(1.60677758290954,-1.,1.32534250785782));
#37791=CARTESIAN_POINT('Ctrl Pts',(1.60073511858687,-1.,1.32381550858256));
#37792=CARTESIAN_POINT('Ctrl Pts',(1.59471591079403,-1.,1.32224985747682));
#37793=CARTESIAN_POINT('Ctrl Pts',(1.58872057258245,-1.,1.32064537110892));
#37794=CARTESIAN_POINT('Ctrl Pts',(1.58274907898834,-1.,1.31900135021432));
#37795=CARTESIAN_POINT('Ctrl Pts',(1.5768005650559,-1.,1.31731642317187));
#37796=CARTESIAN_POINT('Ctrl Pts',(1.57087397835723,-1.,1.31558903860016));
#37797=CARTESIAN_POINT('Ctrl Pts',(1.56496872402353,-1.,1.31381795281002));
#37798=CARTESIAN_POINT('Ctrl Pts',(1.55908521254821,-1.,1.31200264341696));
#37799=CARTESIAN_POINT('Ctrl Pts',(1.55322568759481,-1.,1.31014393684222));
#37800=CARTESIAN_POINT('Ctrl Pts',(1.54739413957185,-1.,1.30824393907473));
#37801=CARTESIAN_POINT('Ctrl Pts',(1.54159462645432,-1.,1.30630475189556));
#37802=CARTESIAN_POINT('Ctrl Pts',(1.53582981268977,-1.,1.30432735639489));
#37803=CARTESIAN_POINT('Ctrl Pts',(1.53009970283891,-1.,1.30231064395568));
#37804=CARTESIAN_POINT('Ctrl Pts',(1.52439957861062,-1.,1.30024984366328));
#37805=CARTESIAN_POINT('Ctrl Pts',(1.51872184912724,-1.,1.29813791800747));
#37806=CARTESIAN_POINT('Ctrl Pts',(1.51305994241402,-1.,1.29596850710509));
#37807=CARTESIAN_POINT('Ctrl Pts',(1.50741159078365,-1.,1.29373841372842));
#37808=CARTESIAN_POINT('Ctrl Pts',(1.50178230149776,-1.,1.29145022885181));
#37809=CARTESIAN_POINT('Ctrl Pts',(1.49618896881754,-1.,1.28911506584254));
#37810=CARTESIAN_POINT('Ctrl Pts',(1.4906522831278,-1.,1.2867467611644));
#37811=CARTESIAN_POINT('Ctrl Pts',(1.4851881711891,-1.,1.28435533880201));
#37812=CARTESIAN_POINT('Ctrl Pts',(1.47980070347095,-1.,1.28194158939517));
#37813=CARTESIAN_POINT('Ctrl Pts',(1.4744717526707,-1.,1.2794891824849));
#37814=CARTESIAN_POINT('Ctrl Pts',(1.46916035917133,-1.,1.2769641483109));
#37815=CARTESIAN_POINT('Ctrl Pts',(1.46382431332476,-1.,1.27433119897822));
#37816=CARTESIAN_POINT('Ctrl Pts',(1.45843906294697,-1.,1.27156805265289));
#37817=CARTESIAN_POINT('Ctrl Pts',(1.45301422764247,-1.,1.2686778680489));
#37818=CARTESIAN_POINT('Ctrl Pts',(1.44761985001662,-1.,1.26570925118868));
#37819=CARTESIAN_POINT('Ctrl Pts',(1.44236470511303,-1.,1.26273903323859));
#37820=CARTESIAN_POINT('Ctrl Pts',(1.43734919180847,-1.,1.25983531012005));
#37821=CARTESIAN_POINT('Ctrl Pts',(1.43262645609691,-1.,1.25702687965755));
#37822=CARTESIAN_POINT('Ctrl Pts',(1.42815938799387,-1.,1.25426945222639));
#37823=CARTESIAN_POINT('Ctrl Pts',(1.42378102115575,-1.,1.2514145557001));
#37824=CARTESIAN_POINT('Ctrl Pts',(1.41923722596025,-1.,1.24824430986571));
#37825=CARTESIAN_POINT('Ctrl Pts',(1.41422913175179,-1.,1.24450600513056));
#37826=CARTESIAN_POINT('Ctrl Pts',(1.40845295531283,-1.,1.23994455029534));
#37827=CARTESIAN_POINT('Ctrl Pts',(1.40164708206106,-1.,1.23434087290423));
#37828=CARTESIAN_POINT('Ctrl Pts',(1.39361389568796,-1.,1.22752961899387));
#37829=CARTESIAN_POINT('Ctrl Pts',(1.38420564527715,-1.,1.21938737280852));
#37830=CARTESIAN_POINT('Ctrl Pts',(1.37331915607905,-1.,1.20982812925645));
#37831=CARTESIAN_POINT('Ctrl Pts',(1.36088705043885,-1.,1.1987959077932));
#37832=CARTESIAN_POINT('Ctrl Pts',(1.34687054001093,-1.,1.18625865667441));
#37833=CARTESIAN_POINT('Ctrl Pts',(1.33437539347008,-1.,1.17501305789857));
#37834=CARTESIAN_POINT('Ctrl Pts',(1.32428080721772,-1.,1.16589330093588));
#37835=CARTESIAN_POINT('Ctrl Pts',(1.31722977216397,-1.,1.15950888730809));
#37836=CARTESIAN_POINT('Ctrl Pts',(1.31362392696032,-1.,1.15624053661742));
#37837=CARTESIAN_POINT('',(1.15624053661742,-1.,1.31362392696033));
#37838=CARTESIAN_POINT('Origin',(0.,-1.,0.));
#37839=CARTESIAN_POINT('',(1.34869019493419,-1.,1.73811241238545));
#37840=CARTESIAN_POINT('Ctrl Pts',(1.15624053661742,-1.,1.31362392696033));
#37841=CARTESIAN_POINT('Ctrl Pts',(1.15950888730433,-1.,1.3172297721596));
#37842=CARTESIAN_POINT('Ctrl Pts',(1.16589330092532,-1.,1.32428080720544));
#37843=CARTESIAN_POINT('Ctrl Pts',(1.17501305787994,-1.,1.33437539344842));
#37844=CARTESIAN_POINT('Ctrl Pts',(1.18625865664915,-1.,1.34687053998157));
#37845=CARTESIAN_POINT('Ctrl Pts',(1.1987959077656,-1.,1.36088705040677));
#37846=CARTESIAN_POINT('Ctrl Pts',(1.20982812923113,-1.,1.37331915604962));
#37847=CARTESIAN_POINT('Ctrl Pts',(1.21938737278853,-1.,1.38420564525391));
#37848=CARTESIAN_POINT('Ctrl Pts',(1.22752961898063,-1.,1.39361389567257));
#37849=CARTESIAN_POINT('Ctrl Pts',(1.23434087289768,-1.,1.40164708205345));
#37850=CARTESIAN_POINT('Ctrl Pts',(1.23994455029421,-1.,1.40845295531151));
#37851=CARTESIAN_POINT('Ctrl Pts',(1.24450600513278,-1.,1.41422913175437));
#37852=CARTESIAN_POINT('Ctrl Pts',(1.24824430986911,-1.,1.41923722596421));
#37853=CARTESIAN_POINT('Ctrl Pts',(1.25141455570299,-1.,1.42378102115911));
#37854=CARTESIAN_POINT('Ctrl Pts',(1.25426945222783,-1.,1.42815938799555));
#37855=CARTESIAN_POINT('Ctrl Pts',(1.25702687965744,-1.,1.43262645609679));
#37856=CARTESIAN_POINT('Ctrl Pts',(1.25983531011894,-1.,1.43734919180719));
#37857=CARTESIAN_POINT('Ctrl Pts',(1.26273903323723,-1.,1.44236470511145));
#37858=CARTESIAN_POINT('Ctrl Pts',(1.26570925118767,-1.,1.44761985001544));
#37859=CARTESIAN_POINT('Ctrl Pts',(1.26867786804854,-1.,1.45301422764205));
#37860=CARTESIAN_POINT('Ctrl Pts',(1.27156805265312,-1.,1.45843906294725));
#37861=CARTESIAN_POINT('Ctrl Pts',(1.27433119897877,-1.,1.4638243133254));
#37862=CARTESIAN_POINT('Ctrl Pts',(1.27696414831144,-1.,1.46916035917197));
#37863=CARTESIAN_POINT('Ctrl Pts',(1.27948918248524,-1.,1.4744717526711));
#37864=CARTESIAN_POINT('Ctrl Pts',(1.28194158939522,-1.,1.47980070347102));
#37865=CARTESIAN_POINT('Ctrl Pts',(1.28435533880184,-1.,1.48518817118891));
#37866=CARTESIAN_POINT('Ctrl Pts',(1.28674676116415,-1.,1.4906522831275));
#37867=CARTESIAN_POINT('Ctrl Pts',(1.28911506584232,-1.,1.49618896881729));
#37868=CARTESIAN_POINT('Ctrl Pts',(1.29145022885171,-1.,1.50178230149764));
#37869=CARTESIAN_POINT('Ctrl Pts',(1.29373841372843,-1.,1.50741159078367));
#37870=CARTESIAN_POINT('Ctrl Pts',(1.29596850710518,-1.,1.51305994241412));
#37871=CARTESIAN_POINT('Ctrl Pts',(1.29813791800757,-1.,1.51872184912735));
#37872=CARTESIAN_POINT('Ctrl Pts',(1.30024984366334,-1.,1.5243995786107));
#37873=CARTESIAN_POINT('Ctrl Pts',(1.3023106439557,-1.,1.53009970283893));
#37874=CARTESIAN_POINT('Ctrl Pts',(1.30432735639487,-1.,1.53582981268976));
#37875=CARTESIAN_POINT('Ctrl Pts',(1.30630475189553,-1.,1.54159462645428));
#37876=CARTESIAN_POINT('Ctrl Pts',(1.30824393907471,-1.,1.54739413957183));
#37877=CARTESIAN_POINT('Ctrl Pts',(1.31014393684221,-1.,1.55322568759481));
#37878=CARTESIAN_POINT('Ctrl Pts',(1.31200264341696,-1.,1.55908521254822));
#37879=CARTESIAN_POINT('Ctrl Pts',(1.31381795281002,-1.,1.56496872402352));
#37880=CARTESIAN_POINT('Ctrl Pts',(1.31558903860015,-1.,1.57087397835721));
#37881=CARTESIAN_POINT('Ctrl Pts',(1.31731642317183,-1.,1.57680056505585));
#37882=CARTESIAN_POINT('Ctrl Pts',(1.31900135021428,-1.,1.58274907898829));
#37883=CARTESIAN_POINT('Ctrl Pts',(1.32064537110891,-1.,1.58872057258244));
#37884=CARTESIAN_POINT('Ctrl Pts',(1.32224985747686,-1.,1.59471591079408));
#37885=CARTESIAN_POINT('Ctrl Pts',(1.32381550858266,-1.,1.600735118587));
#37886=CARTESIAN_POINT('Ctrl Pts',(1.32534250785794,-1.,1.6067775829097));
#37887=CARTESIAN_POINT('Ctrl Pts',(1.32683074483365,-1.,1.61284234015762));
#37888=CARTESIAN_POINT('Ctrl Pts',(1.32828000610448,-1.,1.61892832270723));
#37889=CARTESIAN_POINT('Ctrl Pts',(1.32969019505665,-1.,1.62503464209777));
#37890=CARTESIAN_POINT('Ctrl Pts',(1.33106149345618,-1.,1.63116079730887));
#37891=CARTESIAN_POINT('Ctrl Pts',(1.33239425103694,-1.,1.6373065347505));
#37892=CARTESIAN_POINT('Ctrl Pts',(1.33368890676554,-1.,1.64347174856007));
#37893=CARTESIAN_POINT('Ctrl Pts',(1.33494590468003,-1.,1.64965637286843));
#37894=CARTESIAN_POINT('Ctrl Pts',(1.33616559745217,-1.,1.65586025952651));
#37895=CARTESIAN_POINT('Ctrl Pts',(1.33734820885331,-1.,1.66208312542073));
#37896=CARTESIAN_POINT('Ctrl Pts',(1.33849388654458,-1.,1.66832460784078));
#37897=CARTESIAN_POINT('Ctrl Pts',(1.33960273470372,-1.,1.67458429426126));
#37898=CARTESIAN_POINT('Ctrl Pts',(1.3406748518516,-1.,1.68086176030308));
#37899=CARTESIAN_POINT('Ctrl Pts',(1.34171037484673,-1.,1.68715660868602));
#37900=CARTESIAN_POINT('Ctrl Pts',(1.34270948206139,-1.,1.6934684849664));
#37901=CARTESIAN_POINT('Ctrl Pts',(1.34367237124322,-1.,1.69979707754221));
#37902=CARTESIAN_POINT('Ctrl Pts',(1.34459924533783,-1.,1.70614212266676));
#37903=CARTESIAN_POINT('Ctrl Pts',(1.34549029589563,-1.,1.71250340687011));
#37904=CARTESIAN_POINT('Ctrl Pts',(1.34634568653586,-1.,1.7188807715095));
#37905=CARTESIAN_POINT('Ctrl Pts',(1.34716554820013,-1.,1.72527410681298));
#37906=CARTESIAN_POINT('Ctrl Pts',(1.3477930915247,-1.,1.73040149654497));
#37907=CARTESIAN_POINT('Ctrl Pts',(1.34824783113158,-1.,1.73425417886255));
#37908=CARTESIAN_POINT('Ctrl Pts',(1.34854391898145,-1.,1.73682580585819));
#37909=CARTESIAN_POINT('Ctrl Pts',(1.34869019493419,-1.,1.73811241238545));
#37910=CARTESIAN_POINT('',(1.23627494547115,-1.,1.81978687191668));
#37911=CARTESIAN_POINT('',(1.34869019493419,-1.,1.73811241238545));
#37912=CARTESIAN_POINT('',(0.892032620296855,-1.,1.5055822144029));
#37913=CARTESIAN_POINT('Ctrl Pts',(1.23627494547115,-1.,1.81978687191668));
#37914=CARTESIAN_POINT('Ctrl Pts',(1.23509651170384,-1.,1.81925017193531));
#37915=CARTESIAN_POINT('Ctrl Pts',(1.23274224526804,-1.,1.81817389920914));
#37916=CARTESIAN_POINT('Ctrl Pts',(1.22921864890975,-1.,1.81655087183054));
#37917=CARTESIAN_POINT('Ctrl Pts',(1.22453613304507,-1.,1.81436959209778));
#37918=CARTESIAN_POINT('Ctrl Pts',(1.2187090610323,-1.,1.81161420806172));
#37919=CARTESIAN_POINT('Ctrl Pts',(1.2129081570818,-1.,1.80882996916931));
#37920=CARTESIAN_POINT('Ctrl Pts',(1.20713356605519,-1.,1.80601678480772));
#37921=CARTESIAN_POINT('Ctrl Pts',(1.2013854893912,-1.,1.8031745483882));
#37922=CARTESIAN_POINT('Ctrl Pts',(1.19566418930405,-1.,1.80030314370121));
#37923=CARTESIAN_POINT('Ctrl Pts',(1.1899699793456,-1.,1.79740245923649));
#37924=CARTESIAN_POINT('Ctrl Pts',(1.18430321697471,-1.,1.79447240321572));
#37925=CARTESIAN_POINT('Ctrl Pts',(1.17866429440781,-1.,1.79151291552646));
#37926=CARTESIAN_POINT('Ctrl Pts',(1.17305363177265,-1.,1.78852398877523));
#37927=CARTESIAN_POINT('Ctrl Pts',(1.16747166312239,-1.,1.78550566040349));
#37928=CARTESIAN_POINT('Ctrl Pts',(1.16191881298458,-1.,1.78245795880949));
#37929=CARTESIAN_POINT('Ctrl Pts',(1.15639547194689,-1.,1.77938085564261));
#37930=CARTESIAN_POINT('Ctrl Pts',(1.15090197841531,-1.,1.77627422557034));
#37931=CARTESIAN_POINT('Ctrl Pts',(1.14543858226948,-1.,1.77313777896234));
#37932=CARTESIAN_POINT('Ctrl Pts',(1.14000548337,-1.,1.76997111386806));
#37933=CARTESIAN_POINT('Ctrl Pts',(1.13460291804634,-1.,1.76677384551883));
#37934=CARTESIAN_POINT('Ctrl Pts',(1.12923123555076,-1.,1.76354571966171));
#37935=CARTESIAN_POINT('Ctrl Pts',(1.12389096855078,-1.,1.76028671825084));
#37936=CARTESIAN_POINT('Ctrl Pts',(1.11858293216752,-1.,1.75699720772089));
#37937=CARTESIAN_POINT('Ctrl Pts',(1.11330807582542,-1.,1.75367772094617));
#37938=CARTESIAN_POINT('Ctrl Pts',(1.10806728183003,-1.,1.75032866075914));
#37939=CARTESIAN_POINT('Ctrl Pts',(1.10286118991144,-1.,1.74695004214924));
#37940=CARTESIAN_POINT('Ctrl Pts',(1.09768999241229,-1.,1.74354119236212));
#37941=CARTESIAN_POINT('Ctrl Pts',(1.09255329056496,-1.,1.74010053962252));
#37942=CARTESIAN_POINT('Ctrl Pts',(1.08745056285429,-1.,1.73662628326093));
#37943=CARTESIAN_POINT('Ctrl Pts',(1.08238162784749,-1.,1.73311705663407));
#37944=CARTESIAN_POINT('Ctrl Pts',(1.0773470373727,-1.,1.72957248977424));
#37945=CARTESIAN_POINT('Ctrl Pts',(1.07234866990252,-1.,1.72599406198489));
#37946=CARTESIAN_POINT('Ctrl Pts',(1.06738966975463,-1.,1.72238500928456));
#37947=CARTESIAN_POINT('Ctrl Pts',(1.06247324680649,-1.,1.71874858456908));
#37948=CARTESIAN_POINT('Ctrl Pts',(1.05760163192481,-1.,1.71508654427022));
#37949=CARTESIAN_POINT('Ctrl Pts',(1.05277517202853,-1.,1.71139783543986));
#37950=CARTESIAN_POINT('Ctrl Pts',(1.0479908540499,-1.,1.70767646263641));
#37951=CARTESIAN_POINT('Ctrl Pts',(1.04324363334546,-1.,1.70391338707969));
#37952=CARTESIAN_POINT('Ctrl Pts',(1.03852922490782,-1.,1.70010052930951));
#37953=CARTESIAN_POINT('Ctrl Pts',(1.03384646003587,-1.,1.69623414782769));
#37954=CARTESIAN_POINT('Ctrl Pts',(1.02919977579155,-1.,1.69231840863471));
#37955=CARTESIAN_POINT('Ctrl Pts',(1.02460180535272,-1.,1.68836910178475));
#37956=CARTESIAN_POINT('Ctrl Pts',(1.02006795074222,-1.,1.68440578021739));
#37957=CARTESIAN_POINT('Ctrl Pts',(1.01561026162786,-1.,1.6804428989482));
#37958=CARTESIAN_POINT('Ctrl Pts',(1.01123236493507,-1.,1.67648246776457));
#37959=CARTESIAN_POINT('Ctrl Pts',(1.00692206696387,-1.,1.67250335383248));
#37960=CARTESIAN_POINT('Ctrl Pts',(1.00265091003682,-1.,1.66846059277231));
#37961=CARTESIAN_POINT('Ctrl Pts',(0.998389654952317,-1.,1.66430758030304));
#37962=CARTESIAN_POINT('Ctrl Pts',(0.994121836661115,-1.,1.66001553809916));
#37963=CARTESIAN_POINT('Ctrl Pts',(0.98985562785445,-1.,1.65559044289746));
#37964=CARTESIAN_POINT('Ctrl Pts',(0.985642622921626,-1.,1.6511001661277));
#37965=CARTESIAN_POINT('Ctrl Pts',(0.981562530940574,-1.,1.64665139190834));
#37966=CARTESIAN_POINT('Ctrl Pts',(0.977689794120296,-1.,1.64233990826831));
#37967=CARTESIAN_POINT('Ctrl Pts',(0.974066058287501,-1.,1.63820952658157));
#37968=CARTESIAN_POINT('Ctrl Pts',(0.970669715996356,-1.,1.63420665729609));
#37969=CARTESIAN_POINT('Ctrl Pts',(0.967387853228041,-1.,1.63013849959083));
#37970=CARTESIAN_POINT('Ctrl Pts',(0.964046107037821,-1.,1.6257193066974));
#37971=CARTESIAN_POINT('Ctrl Pts',(0.960438326099958,-1.,1.62061638139929));
#37972=CARTESIAN_POINT('Ctrl Pts',(0.956354422921572,-1.,1.61449324337233));
#37973=CARTESIAN_POINT('Ctrl Pts',(0.951613284361247,-1.,1.60706069897794));
#37974=CARTESIAN_POINT('Ctrl Pts',(0.946078063325795,-1.,1.59810042045408));
#37975=CARTESIAN_POINT('Ctrl Pts',(0.939646377909319,-1.,1.58744937489796));
#37976=CARTESIAN_POINT('Ctrl Pts',(0.932246680128848,-1.,1.57499388385561));
#37977=CARTESIAN_POINT('Ctrl Pts',(0.923832188966322,-1.,1.56065988582509));
#37978=CARTESIAN_POINT('Ctrl Pts',(0.914375919046579,-1.,1.54440491152808));
#37979=CARTESIAN_POINT('Ctrl Pts',(0.905967409640498,-1.,1.52984849890434));
#37980=CARTESIAN_POINT('Ctrl Pts',(0.89918504749193,-1.,1.51805569591479));
#37981=CARTESIAN_POINT('Ctrl Pts',(0.894452006967538,-1.,1.50980486807181));
#37982=CARTESIAN_POINT('Ctrl Pts',(0.892032620296855,-1.,1.5055822144029));
#37983=CARTESIAN_POINT('',(0.693717979106305,-1.,1.60662857109684));
#37984=CARTESIAN_POINT('Origin',(0.,-1.,0.));
#37985=CARTESIAN_POINT('',(0.7455743247944,-1.,2.0698113262342));
#37986=CARTESIAN_POINT('Ctrl Pts',(0.693717979106305,-1.,1.60662857109684));
#37987=CARTESIAN_POINT('Ctrl Pts',(0.69571209787897,-1.,1.61106790957619));
#37988=CARTESIAN_POINT('Ctrl Pts',(0.699605146398836,-1.,1.61974673471117));
#37989=CARTESIAN_POINT('Ctrl Pts',(0.705159151977294,-1.,1.6321654166204));
#37990=CARTESIAN_POINT('Ctrl Pts',(0.711993139340447,-1.,1.64752408828442));
#37991=CARTESIAN_POINT('Ctrl Pts',(0.719585433787949,-1.,1.66472880551777));
#37992=CARTESIAN_POINT('Ctrl Pts',(0.726235967982445,-1.,1.67996158451922));
#37993=CARTESIAN_POINT('Ctrl Pts',(0.731963238685357,-1.,1.69326921972915));
#37994=CARTESIAN_POINT('Ctrl Pts',(0.736799665716932,-1.,1.70473309004249));
#37995=CARTESIAN_POINT('Ctrl Pts',(0.74079516202821,-1.,1.71447789751001));
#37996=CARTESIAN_POINT('Ctrl Pts',(0.744021445433093,-1.,1.72268229916769));
#37997=CARTESIAN_POINT('Ctrl Pts',(0.746574710097752,-1.,1.72958533647714));
#37998=CARTESIAN_POINT('Ctrl Pts',(0.74858246295687,-1.,1.7355035168033));
#37999=CARTESIAN_POINT('Ctrl Pts',(0.750193435981249,-1.,1.74080458267114));
#38000=CARTESIAN_POINT('Ctrl Pts',(0.751555614164482,-1.,1.74585086852502));
#38001=CARTESIAN_POINT('Ctrl Pts',(0.752797683531314,-1.,1.75095139468794));
#38002=CARTESIAN_POINT('Ctrl Pts',(0.754009254027828,-1.,1.75631083600019));
#38003=CARTESIAN_POINT('Ctrl Pts',(0.755220979974461,-1.,1.76197817240128));
#38004=CARTESIAN_POINT('Ctrl Pts',(0.75642189602781,-1.,1.76789396002998));
#38005=CARTESIAN_POINT('Ctrl Pts',(0.757578264077028,-1.,1.77394167108292));
#38006=CARTESIAN_POINT('Ctrl Pts',(0.758650626677518,-1.,1.77999411220945));
#38007=CARTESIAN_POINT('Ctrl Pts',(0.759614401110189,-1.,1.78596964884604));
#38008=CARTESIAN_POINT('Ctrl Pts',(0.760469555880749,-1.,1.7918581561088));
#38009=CARTESIAN_POINT('Ctrl Pts',(0.761229695230558,-1.,1.79768986997783));
#38010=CARTESIAN_POINT('Ctrl Pts',(0.761915336443547,-1.,1.80351583877342));
#38011=CARTESIAN_POINT('Ctrl Pts',(0.762546129463938,-1.,1.80938551463965));
#38012=CARTESIAN_POINT('Ctrl Pts',(0.763132003836634,-1.,1.8153211840553));
#38013=CARTESIAN_POINT('Ctrl Pts',(0.763673465462726,-1.,1.82131873145266));
#38014=CARTESIAN_POINT('Ctrl Pts',(0.764165902605995,-1.,1.82735991200065));
#38015=CARTESIAN_POINT('Ctrl Pts',(0.764602549687853,-1.,1.83342077227142));
#38016=CARTESIAN_POINT('Ctrl Pts',(0.764978057881737,-1.,1.83948181064835));
#38017=CARTESIAN_POINT('Ctrl Pts',(0.765291664862029,-1.,1.84553698875924));
#38018=CARTESIAN_POINT('Ctrl Pts',(0.765545710619062,-1.,1.85158945130063));
#38019=CARTESIAN_POINT('Ctrl Pts',(0.765744212909318,-1.,1.85764741390394));
#38020=CARTESIAN_POINT('Ctrl Pts',(0.765891519092547,-1.,1.86372027063312));
#38021=CARTESIAN_POINT('Ctrl Pts',(0.765990708546091,-1.,1.86981398314341));
#38022=CARTESIAN_POINT('Ctrl Pts',(0.766042837036744,-1.,1.87592888967883));
#38023=CARTESIAN_POINT('Ctrl Pts',(0.766047794851864,-1.,1.88206215302561));
#38024=CARTESIAN_POINT('Ctrl Pts',(0.766004837062091,-1.,1.88820926433409));
#38025=CARTESIAN_POINT('Ctrl Pts',(0.765913193856978,-1.,1.89436577771388));
#38026=CARTESIAN_POINT('Ctrl Pts',(0.765772772593386,-1.,1.90052930393596));
#38027=CARTESIAN_POINT('Ctrl Pts',(0.765584196937919,-1.,1.90669961402356));
#38028=CARTESIAN_POINT('Ctrl Pts',(0.765348465884722,-1.,1.91287765805169));
#38029=CARTESIAN_POINT('Ctrl Pts',(0.765066729667088,-1.,1.91906491634196));
#38030=CARTESIAN_POINT('Ctrl Pts',(0.764740025488211,-1.,1.92526263537048));
#38031=CARTESIAN_POINT('Ctrl Pts',(0.76436901067394,-1.,1.93147105496382));
#38032=CARTESIAN_POINT('Ctrl Pts',(0.763954049121458,-1.,1.93768964875886));
#38033=CARTESIAN_POINT('Ctrl Pts',(0.763495333538629,-1.,1.9439174661764));
#38034=CARTESIAN_POINT('Ctrl Pts',(0.762992990878769,-1.,1.95015342590024));
#38035=CARTESIAN_POINT('Ctrl Pts',(0.762447203806178,-1.,1.95639665309869));
#38036=CARTESIAN_POINT('Ctrl Pts',(0.761858300014423,-1.,1.96264672744186));
#38037=CARTESIAN_POINT('Ctrl Pts',(0.76122669048382,-1.,1.96890351582499));
#38038=CARTESIAN_POINT('Ctrl Pts',(0.760552825409757,-1.,1.97516705321494));
#38039=CARTESIAN_POINT('Ctrl Pts',(0.75983714745219,-1.,1.98143741418172));
#38040=CARTESIAN_POINT('Ctrl Pts',(0.759080037802488,-1.,1.98771456680874));
#38041=CARTESIAN_POINT('Ctrl Pts',(0.758281796766761,-1.,1.99399831098817));
#38042=CARTESIAN_POINT('Ctrl Pts',(0.757442676862724,-1.,2.00028834739178));
#38043=CARTESIAN_POINT('Ctrl Pts',(0.75656290464667,-1.,2.0065843158773));
#38044=CARTESIAN_POINT('Ctrl Pts',(0.755642704957865,-1.,2.01288584328084));
#38045=CARTESIAN_POINT('Ctrl Pts',(0.754682330722816,-1.,2.01919259405809));
#38046=CARTESIAN_POINT('Ctrl Pts',(0.753682061112768,-1.,2.02550428623313));
#38047=CARTESIAN_POINT('Ctrl Pts',(0.75264218048721,-1.,2.03182068456221));
#38048=CARTESIAN_POINT('Ctrl Pts',(0.751562963361115,-1.,2.03814160092099));
#38049=CARTESIAN_POINT('Ctrl Pts',(0.750444657875575,-1.,2.04446689147979));
#38050=CARTESIAN_POINT('Ctrl Pts',(0.749287468665046,-1.,2.05079645592154));
#38051=CARTESIAN_POINT('Ctrl Pts',(0.748091554183802,-1.,2.05713023031007));
#38052=CARTESIAN_POINT('Ctrl Pts',(0.747103932787919,-1.,2.06220058927826));
#38053=CARTESIAN_POINT('Ctrl Pts',(0.7463458715442,-1.,2.06600523016815));
#38054=CARTESIAN_POINT('Ctrl Pts',(0.745832791378367,-1.,2.06854248895728));
#38055=CARTESIAN_POINT('Ctrl Pts',(0.7455743247944,-1.,2.0698113262342));
#38056=CARTESIAN_POINT('',(0.61342227326009,-1.,2.11275013067528));
#38057=CARTESIAN_POINT('',(0.7455743247944,-1.,2.0698113262342));
#38058=CARTESIAN_POINT('',(0.383122945602004,-1.,1.7075470150345));
#38059=CARTESIAN_POINT('Ctrl Pts',(0.61342227326009,-1.,2.11275013067528));
#38060=CARTESIAN_POINT('Ctrl Pts',(0.6124673655618,-1.,2.11187554259986));
#38061=CARTESIAN_POINT('Ctrl Pts',(0.610560911689898,-1.,2.11012443807238));
#38062=CARTESIAN_POINT('Ctrl Pts',(0.607711315454876,-1.,2.1074919961518));
#38063=CARTESIAN_POINT('Ctrl Pts',(0.60393203073603,-1.,2.10397049886949));
#38064=CARTESIAN_POINT('Ctrl Pts',(0.599241616420533,-1.,2.0995493086477));
#38065=CARTESIAN_POINT('Ctrl Pts',(0.594585006052162,-1.,2.0951087622027));
#38066=CARTESIAN_POINT('Ctrl Pts',(0.589962365403406,-1.,2.09064881812129));
#38067=CARTESIAN_POINT('Ctrl Pts',(0.585373918991617,-1.,2.08616943727951));
#38068=CARTESIAN_POINT('Ctrl Pts',(0.580819952108063,-1.,2.08167059018418));
#38069=CARTESIAN_POINT('Ctrl Pts',(0.576300797416844,-1.,2.07715226767559));
#38070=CARTESIAN_POINT('Ctrl Pts',(0.571816823242602,-1.,2.07261449292824));
#38071=CARTESIAN_POINT('Ctrl Pts',(0.567368421181087,-1.,2.06805732997334));
#38072=CARTESIAN_POINT('Ctrl Pts',(0.562955993082261,-1.,2.06348090160589));
#38073=CARTESIAN_POINT('Ctrl Pts',(0.558579940185151,-1.,2.05888537756462));
#38074=CARTESIAN_POINT('Ctrl Pts',(0.554240657463906,-1.,2.05427091604413));
#38075=CARTESIAN_POINT('Ctrl Pts',(0.549938525150295,-1.,2.04963761077958));
#38076=CARTESIAN_POINT('Ctrl Pts',(0.54567390381743,-1.,2.04498544714588));
#38077=CARTESIAN_POINT('Ctrl Pts',(0.541447120615659,-1.,2.04031422690527));
#38078=CARTESIAN_POINT('Ctrl Pts',(0.537258489833262,-1.,2.03562362954037));
#38079=CARTESIAN_POINT('Ctrl Pts',(0.533108355132976,-1.,2.03091336214426));
#38080=CARTESIAN_POINT('Ctrl Pts',(0.528997127241914,-1.,2.0261832908329));
#38081=CARTESIAN_POINT('Ctrl Pts',(0.524925318333476,-1.,2.02143356304698));
#38082=CARTESIAN_POINT('Ctrl Pts',(0.52089359039937,-1.,2.01666477917286));
#38083=CARTESIAN_POINT('Ctrl Pts',(0.516902681728687,-1.,2.01187773939242));
#38084=CARTESIAN_POINT('Ctrl Pts',(0.512953306961792,-1.,2.00707309946949));
#38085=CARTESIAN_POINT('Ctrl Pts',(0.509046069886157,-1.,2.00225107134734));
#38086=CARTESIAN_POINT('Ctrl Pts',(0.505181361323026,-1.,1.99741107463572));
#38087=CARTESIAN_POINT('Ctrl Pts',(0.501359287727146,-1.,1.99255149126155));
#38088=CARTESIAN_POINT('Ctrl Pts',(0.497579909545574,-1.,1.98767044752932));
#38089=CARTESIAN_POINT('Ctrl Pts',(0.493843476541494,-1.,1.98276658761821));
#38090=CARTESIAN_POINT('Ctrl Pts',(0.490150627860952,-1.,1.97783973019229));
#38091=CARTESIAN_POINT('Ctrl Pts',(0.486502692907658,-1.,1.97289186263272));
#38092=CARTESIAN_POINT('Ctrl Pts',(0.48290166212069,-1.,1.96792703422362));
#38093=CARTESIAN_POINT('Ctrl Pts',(0.479349583074855,-1.,1.96294933055943));
#38094=CARTESIAN_POINT('Ctrl Pts',(0.475848034683176,-1.,1.95796111148177));
#38095=CARTESIAN_POINT('Ctrl Pts',(0.472397672264072,-1.,1.95296148278133));
#38096=CARTESIAN_POINT('Ctrl Pts',(0.468997482913135,-1.,1.94794381136514));
#38097=CARTESIAN_POINT('Ctrl Pts',(0.46564546202603,-1.,1.9428979419619));
#38098=CARTESIAN_POINT('Ctrl Pts',(0.462340031009056,-1.,1.93781486640821));
#38099=CARTESIAN_POINT('Ctrl Pts',(0.459081234547926,-1.,1.93269066517934));
#38100=CARTESIAN_POINT('Ctrl Pts',(0.45587200517437,-1.,1.92753067150476));
#38101=CARTESIAN_POINT('Ctrl Pts',(0.452719478359432,-1.,1.92235380648502));
#38102=CARTESIAN_POINT('Ctrl Pts',(0.449632260106662,-1.,1.91718342555755));
#38103=CARTESIAN_POINT('Ctrl Pts',(0.446617343485711,-1.,1.9120369998112));
#38104=CARTESIAN_POINT('Ctrl Pts',(0.44367755684915,-1.,1.90691756144898));
#38105=CARTESIAN_POINT('Ctrl Pts',(0.440807833704038,-1.,1.90180124389086));
#38106=CARTESIAN_POINT('Ctrl Pts',(0.437995003948244,-1.,1.89663648956466));
#38107=CARTESIAN_POINT('Ctrl Pts',(0.435225660963383,-1.,1.89136993975504));
#38108=CARTESIAN_POINT('Ctrl Pts',(0.432493038548748,-1.,1.88596913666793));
#38109=CARTESIAN_POINT('Ctrl Pts',(0.429803062482344,-1.,1.88044229001832));
#38110=CARTESIAN_POINT('Ctrl Pts',(0.427183828519102,-1.,1.87486989291484));
#38111=CARTESIAN_POINT('Ctrl Pts',(0.424678177291358,-1.,1.86937803944323));
#38112=CARTESIAN_POINT('Ctrl Pts',(0.422327307418275,-1.,1.86408083334028));
#38113=CARTESIAN_POINT('Ctrl Pts',(0.420157287975619,-1.,1.85903281096686));
#38114=CARTESIAN_POINT('Ctrl Pts',(0.418164129143534,-1.,1.85417632856234));
#38115=CARTESIAN_POINT('Ctrl Pts',(0.416300022038864,-1.,1.84929312929882));
#38116=CARTESIAN_POINT('Ctrl Pts',(0.41448743825434,-1.,1.8440575707371));
#38117=CARTESIAN_POINT('Ctrl Pts',(0.412633125322161,-1.,1.83808953475839));
#38118=CARTESIAN_POINT('Ctrl Pts',(0.410641256301674,-1.,1.83100408895216));
#38119=CARTESIAN_POINT('Ctrl Pts',(0.408428948108533,-1.,1.8224702267854));
#38120=CARTESIAN_POINT('Ctrl Pts',(0.405933518411838,-1.,1.81223801813988));
#38121=CARTESIAN_POINT('Ctrl Pts',(0.403107976170441,-1.,1.80012077176221));
#38122=CARTESIAN_POINT('Ctrl Pts',(0.39991940378308,-1.,1.78598826347533));
#38123=CARTESIAN_POINT('Ctrl Pts',(0.39634619612042,-1.,1.7697556004756));
#38124=CARTESIAN_POINT('Ctrl Pts',(0.392375812294307,-1.,1.75137405313962));
#38125=CARTESIAN_POINT('Ctrl Pts',(0.388877023509191,-1.,1.7349317097561));
#38126=CARTESIAN_POINT('Ctrl Pts',(0.38607079032701,-1.,1.72162022246158));
#38127=CARTESIAN_POINT('Ctrl Pts',(0.384119047315541,-1.,1.71231062891958));
#38128=CARTESIAN_POINT('Ctrl Pts',(0.383122945602004,-1.,1.7075470150345));
#38129=CARTESIAN_POINT('',(0.163289472382896,-1.,1.74236521665491));
#38130=CARTESIAN_POINT('Origin',(0.,-1.,0.));
#38131=CARTESIAN_POINT('',(0.0694764450219578,-1.,2.19890268624765));
#38132=CARTESIAN_POINT('Ctrl Pts',(0.163289472382896,-1.,1.74236521665491));
#38133=CARTESIAN_POINT('Ctrl Pts',(0.163814161002002,-1.,1.7472034950333));
#38134=CARTESIAN_POINT('Ctrl Pts',(0.164834765707158,-1.,1.75666056638427));
#38135=CARTESIAN_POINT('Ctrl Pts',(0.1662793551464,-1.,1.77018771684844));
#38136=CARTESIAN_POINT('Ctrl Pts',(0.168032772805197,-1.,1.7869064998507));
#38137=CARTESIAN_POINT('Ctrl Pts',(0.169936923904608,-1.,1.80561530629706));
#38138=CARTESIAN_POINT('Ctrl Pts',(0.171554770204119,-1.,1.82215766811545));
#38139=CARTESIAN_POINT('Ctrl Pts',(0.1728894428919,-1.,1.83658380527692));
#38140=CARTESIAN_POINT('Ctrl Pts',(0.173946627587731,-1.,1.8489811319852));
#38141=CARTESIAN_POINT('Ctrl Pts',(0.17473525927603,-1.,1.85948367088837));
#38142=CARTESIAN_POINT('Ctrl Pts',(0.175268337590757,-1.,1.86828349694799));
#38143=CARTESIAN_POINT('Ctrl Pts',(0.175563480746485,-1.,1.87563767773588));
#38144=CARTESIAN_POINT('Ctrl Pts',(0.175644148889698,-1.,1.88188663145367));
#38145=CARTESIAN_POINT('Ctrl Pts',(0.175538155840648,-1.,1.88742606273259));
#38146=CARTESIAN_POINT('Ctrl Pts',(0.175274276190844,-1.,1.892646301985));
#38147=CARTESIAN_POINT('Ctrl Pts',(0.174879405091263,-1.,1.89788101117132));
#38148=CARTESIAN_POINT('Ctrl Pts',(0.174375518661085,-1.,1.90335253862834));
#38149=CARTESIAN_POINT('Ctrl Pts',(0.173776635257816,-1.,1.90911693975267));
#38150=CARTESIAN_POINT('Ctrl Pts',(0.173090695383496,-1.,1.91511429159527));
#38151=CARTESIAN_POINT('Ctrl Pts',(0.172321621259513,-1.,1.9212233439798));
#38152=CARTESIAN_POINT('Ctrl Pts',(0.171471191532988,-1.,1.92731093582036));
#38153=CARTESIAN_POINT('Ctrl Pts',(0.170541253116201,-1.,1.93329183155539));
#38154=CARTESIAN_POINT('Ctrl Pts',(0.16953490481749,-1.,1.93915639211581));
#38155=CARTESIAN_POINT('Ctrl Pts',(0.168455741607556,-1.,1.94493757756931));
#38156=CARTESIAN_POINT('Ctrl Pts',(0.167307501784475,-1.,1.95069027794294));
#38157=CARTESIAN_POINT('Ctrl Pts',(0.166093592002812,-1.,1.9564675971873));
#38158=CARTESIAN_POINT('Ctrl Pts',(0.164816568920269,-1.,1.96229379940136));
#38159=CARTESIAN_POINT('Ctrl Pts',(0.163478185457734,-1.,1.96816512677967));
#38160=CARTESIAN_POINT('Ctrl Pts',(0.162079693556288,-1.,1.97406280235188));
#38161=CARTESIAN_POINT('Ctrl Pts',(0.160622060784611,-1.,1.97996195437559));
#38162=CARTESIAN_POINT('Ctrl Pts',(0.159106226437299,-1.,1.98584238283292));
#38163=CARTESIAN_POINT('Ctrl Pts',(0.157533331459227,-1.,1.99169810931908));
#38164=CARTESIAN_POINT('Ctrl Pts',(0.155904629548783,-1.,1.99753284771497));
#38165=CARTESIAN_POINT('Ctrl Pts',(0.154221403049722,-1.,2.00335565310543));
#38166=CARTESIAN_POINT('Ctrl Pts',(0.152484883621449,-1.,2.00917680318424));
#38167=CARTESIAN_POINT('Ctrl Pts',(0.150696157673078,-1.,2.01500291940238));
#38168=CARTESIAN_POINT('Ctrl Pts',(0.148856124775337,-1.,2.02083464969894));
#38169=CARTESIAN_POINT('Ctrl Pts',(0.146965557332583,-1.,2.02666926182017));
#38170=CARTESIAN_POINT('Ctrl Pts',(0.145025140186057,-1.,2.03250223739942));
#38171=CARTESIAN_POINT('Ctrl Pts',(0.143035515058208,-1.,2.03832911025912));
#38172=CARTESIAN_POINT('Ctrl Pts',(0.140997332152546,-1.,2.04414757947916));
#38173=CARTESIAN_POINT('Ctrl Pts',(0.138911255368966,-1.,2.04995762001328));
#38174=CARTESIAN_POINT('Ctrl Pts',(0.136777941218043,-1.,2.05576044414264));
#38175=CARTESIAN_POINT('Ctrl Pts',(0.134598026192106,-1.,2.06155781517842));
#38176=CARTESIAN_POINT('Ctrl Pts',(0.13237211154771,-1.,2.06735123910326));
#38177=CARTESIAN_POINT('Ctrl Pts',(0.130100748328403,-1.,2.07314114713063));
#38178=CARTESIAN_POINT('Ctrl Pts',(0.12778444527612,-1.,2.07892715110987));
#38179=CARTESIAN_POINT('Ctrl Pts',(0.125423679412061,-1.,2.08470840653643));
#38180=CARTESIAN_POINT('Ctrl Pts',(0.123018905621083,-1.,2.09048392424825));
#38181=CARTESIAN_POINT('Ctrl Pts',(0.120570567965122,-1.,2.0962529286773));
#38182=CARTESIAN_POINT('Ctrl Pts',(0.118079107988355,-1.,2.102015121329));
#38183=CARTESIAN_POINT('Ctrl Pts',(0.115544957687926,-1.,2.10777050261309));
#38184=CARTESIAN_POINT('Ctrl Pts',(0.112968534419737,-1.,2.11351924490306));
#38185=CARTESIAN_POINT('Ctrl Pts',(0.110350236135025,-1.,2.11926155590865));
#38186=CARTESIAN_POINT('Ctrl Pts',(0.10769043523109,-1.,2.12499752307));
#38187=CARTESIAN_POINT('Ctrl Pts',(0.104989479152739,-1.,2.13072704887293));
#38188=CARTESIAN_POINT('Ctrl Pts',(0.1022477005561,-1.,2.13644992667165));
#38189=CARTESIAN_POINT('Ctrl Pts',(0.0994654261990913,-1.,2.14216588396025));
#38190=CARTESIAN_POINT('Ctrl Pts',(0.0966429852305456,-1.,2.14787463531795));
#38191=CARTESIAN_POINT('Ctrl Pts',(0.0937807218867641,-1.,2.1535759397817));
#38192=CARTESIAN_POINT('Ctrl Pts',(0.0908789888107263,-1.,2.15926961544516));
#38193=CARTESIAN_POINT('Ctrl Pts',(0.087938129138692,-1.,2.16495552645014));
#38194=CARTESIAN_POINT('Ctrl Pts',(0.084958462083537,-1.,2.17063357870952));
#38195=CARTESIAN_POINT('Ctrl Pts',(0.0819402680872763,-1.,2.176303712113));
#38196=CARTESIAN_POINT('Ctrl Pts',(0.078883772768524,-1.,2.18196589448887));
#38197=CARTESIAN_POINT('Ctrl Pts',(0.0757891465836145,-1.,2.1876201139953));
#38198=CARTESIAN_POINT('Ctrl Pts',(0.0732830357306722,-1.,2.19213712013662));
#38199=CARTESIAN_POINT('Ctrl Pts',(0.0713863779526151,-1.,2.19552129484002));
#38200=CARTESIAN_POINT('Ctrl Pts',(0.0701143536325487,-1.,2.19777582085423));
#38201=CARTESIAN_POINT('Ctrl Pts',(0.0694764450219578,-1.,2.19890268624765));
#38202=CARTESIAN_POINT('',(-0.0694764450219586,-1.,2.19890268624765));
#38203=CARTESIAN_POINT('',(0.0694764450219578,-1.,2.19890268624765));
#38204=CARTESIAN_POINT('',(-0.163289472382896,-1.,1.74236521665491));
#38205=CARTESIAN_POINT('Ctrl Pts',(-0.0694764450219586,-1.,2.19890268624765));
#38206=CARTESIAN_POINT('Ctrl Pts',(-0.0701143536324929,-1.,2.19777582085261));
#38207=CARTESIAN_POINT('Ctrl Pts',(-0.071386377952463,-1.,2.19552129483562));
#38208=CARTESIAN_POINT('Ctrl Pts',(-0.0732830357304279,-1.,2.19213712012956));
#38209=CARTESIAN_POINT('Ctrl Pts',(-0.0757891465833414,-1.,2.1876201139874));
#38210=CARTESIAN_POINT('Ctrl Pts',(-0.078883772768323,-1.,2.18196589448304));
#38211=CARTESIAN_POINT('Ctrl Pts',(-0.0819402680871942,-1.,2.1763037121106));
#38212=CARTESIAN_POINT('Ctrl Pts',(-0.0849584620835646,-1.,2.17063357871031));
#38213=CARTESIAN_POINT('Ctrl Pts',(-0.0879381291387825,-1.,2.16495552645275));
#38214=CARTESIAN_POINT('Ctrl Pts',(-0.0908789888108269,-1.,2.15926961544808));
#38215=CARTESIAN_POINT('Ctrl Pts',(-0.0937807218868348,-1.,2.15357593978377));
#38216=CARTESIAN_POINT('Ctrl Pts',(-0.0966429852305691,-1.,2.14787463531864));
#38217=CARTESIAN_POINT('Ctrl Pts',(-0.0994654261990745,-1.,2.14216588395974));
#38218=CARTESIAN_POINT('Ctrl Pts',(-0.102247700556064,-1.,2.13644992667052));
#38219=CARTESIAN_POINT('Ctrl Pts',(-0.104989479152703,-1.,2.1307270488718));
#38220=CARTESIAN_POINT('Ctrl Pts',(-0.107690435231068,-1.,2.12499752306927));
#38221=CARTESIAN_POINT('Ctrl Pts',(-0.11035023613502,-1.,2.11926155590849));
#38222=CARTESIAN_POINT('Ctrl Pts',(-0.112968534419746,-1.,2.11351924490335));
#38223=CARTESIAN_POINT('Ctrl Pts',(-0.115544957687941,-1.,2.10777050261359));
#38224=CARTESIAN_POINT('Ctrl Pts',(-0.118079107988368,-1.,2.10201512132945));
#38225=CARTESIAN_POINT('Ctrl Pts',(-0.120570567965129,-1.,2.09625292867756));
#38226=CARTESIAN_POINT('Ctrl Pts',(-0.123018905621083,-1.,2.09048392424826));
#38227=CARTESIAN_POINT('Ctrl Pts',(-0.125423679412058,-1.,2.08470840653628));
#38228=CARTESIAN_POINT('Ctrl Pts',(-0.127784445276116,-1.,2.07892715110967));
#38229=CARTESIAN_POINT('Ctrl Pts',(-0.130100748328401,-1.,2.07314114713047));
#38230=CARTESIAN_POINT('Ctrl Pts',(-0.13237211154771,-1.,2.06735123910319));
#38231=CARTESIAN_POINT('Ctrl Pts',(-0.134598026192107,-1.,2.06155781517844));
#38232=CARTESIAN_POINT('Ctrl Pts',(-0.136777941218044,-1.,2.0557604441427));
#38233=CARTESIAN_POINT('Ctrl Pts',(-0.138911255368966,-1.,2.04995762001333));
#38234=CARTESIAN_POINT('Ctrl Pts',(-0.140997332152546,-1.,2.04414757947919));
#38235=CARTESIAN_POINT('Ctrl Pts',(-0.143035515058208,-1.,2.03832911025913));
#38236=CARTESIAN_POINT('Ctrl Pts',(-0.145025140186058,-1.,2.03250223739941));
#38237=CARTESIAN_POINT('Ctrl Pts',(-0.146965557332586,-1.,2.02666926182017));
#38238=CARTESIAN_POINT('Ctrl Pts',(-0.148856124775343,-1.,2.02083464969897));
#38239=CARTESIAN_POINT('Ctrl Pts',(-0.150696157673084,-1.,2.01500291940243));
#38240=CARTESIAN_POINT('Ctrl Pts',(-0.152484883621452,-1.,2.00917680318426));
#38241=CARTESIAN_POINT('Ctrl Pts',(-0.154221403049719,-1.,2.00335565310539));
#38242=CARTESIAN_POINT('Ctrl Pts',(-0.155904629548775,-1.,1.99753284771487));
#38243=CARTESIAN_POINT('Ctrl Pts',(-0.157533331459215,-1.,1.99169810931893));
#38244=CARTESIAN_POINT('Ctrl Pts',(-0.159106226437289,-1.,1.98584238283279));
#38245=CARTESIAN_POINT('Ctrl Pts',(-0.16062206078461,-1.,1.97996195437557));
#38246=CARTESIAN_POINT('Ctrl Pts',(-0.162079693556302,-1.,1.97406280235204));
#38247=CARTESIAN_POINT('Ctrl Pts',(-0.16347818545776,-1.,1.96816512678));
#38248=CARTESIAN_POINT('Ctrl Pts',(-0.1648165689203,-1.,1.96229379940174));
#38249=CARTESIAN_POINT('Ctrl Pts',(-0.166093592002833,-1.,1.95646759718755));
#38250=CARTESIAN_POINT('Ctrl Pts',(-0.167307501784469,-1.,1.95069027794286));
#38251=CARTESIAN_POINT('Ctrl Pts',(-0.168455741607516,-1.,1.94493757756879));
#38252=CARTESIAN_POINT('Ctrl Pts',(-0.169534904817425,-1.,1.93915639211497));
#38253=CARTESIAN_POINT('Ctrl Pts',(-0.170541253116136,-1.,1.93329183155455));
#38254=CARTESIAN_POINT('Ctrl Pts',(-0.17147119153296,-1.,1.92731093582));
#38255=CARTESIAN_POINT('Ctrl Pts',(-0.172321621259557,-1.,1.92122334398034));
#38256=CARTESIAN_POINT('Ctrl Pts',(-0.173090695383619,-1.,1.91511429159681));
#38257=CARTESIAN_POINT('Ctrl Pts',(-0.173776635257984,-1.,1.90911693975475));
#38258=CARTESIAN_POINT('Ctrl Pts',(-0.174375518661222,-1.,1.90335253863003));
#38259=CARTESIAN_POINT('Ctrl Pts',(-0.174879405091277,-1.,1.89788101117148));
#38260=CARTESIAN_POINT('Ctrl Pts',(-0.175274276190664,-1.,1.89264630198279));
#38261=CARTESIAN_POINT('Ctrl Pts',(-0.175538155840286,-1.,1.88742606272818));
#38262=CARTESIAN_POINT('Ctrl Pts',(-0.175644148889271,-1.,1.88188663144846));
#38263=CARTESIAN_POINT('Ctrl Pts',(-0.175563480746206,-1.,1.87563767773249));
#38264=CARTESIAN_POINT('Ctrl Pts',(-0.175268337590901,-1.,1.86828349694972));
#38265=CARTESIAN_POINT('Ctrl Pts',(-0.174735259276856,-1.,1.85948367089838));
#38266=CARTESIAN_POINT('Ctrl Pts',(-0.173946627589401,-1.,1.84898113200543));
#38267=CARTESIAN_POINT('Ctrl Pts',(-0.17288944289442,-1.,1.83658380530747));
#38268=CARTESIAN_POINT('Ctrl Pts',(-0.171554770207306,-1.,1.82215766815414));
#38269=CARTESIAN_POINT('Ctrl Pts',(-0.169936923908078,-1.,1.80561530633924));
#38270=CARTESIAN_POINT('Ctrl Pts',(-0.16803277280837,-1.,1.78690649988931));
#38271=CARTESIAN_POINT('Ctrl Pts',(-0.166279355148738,-1.,1.77018771687692));
#38272=CARTESIAN_POINT('Ctrl Pts',(-0.164834765708484,-1.,1.75666056640041));
#38273=CARTESIAN_POINT('Ctrl Pts',(-0.163814161002474,-1.,1.74720349503904));
#38274=CARTESIAN_POINT('Ctrl Pts',(-0.163289472382896,-1.,1.74236521665491));
#38275=CARTESIAN_POINT('',(-0.383122945602004,-1.,1.7075470150345));
#38276=CARTESIAN_POINT('Origin',(0.,-1.,0.));
#38277=CARTESIAN_POINT('',(-0.61342227326009,-1.,2.11275013067528));
#38278=CARTESIAN_POINT('Ctrl Pts',(-0.383122945602004,-1.,1.7075470150345));
#38279=CARTESIAN_POINT('Ctrl Pts',(-0.384119047314215,-1.,1.71231062891398));
#38280=CARTESIAN_POINT('Ctrl Pts',(-0.386070790323281,-1.,1.72162022244582));
#38281=CARTESIAN_POINT('Ctrl Pts',(-0.388877023502615,-1.,1.73493170972829));
#38282=CARTESIAN_POINT('Ctrl Pts',(-0.392375812285395,-1.,1.75137405310193));
#38283=CARTESIAN_POINT('Ctrl Pts',(-0.396346196110688,-1.,1.76975560043442));
#38284=CARTESIAN_POINT('Ctrl Pts',(-0.399919403774155,-1.,1.78598826343754));
#38285=CARTESIAN_POINT('Ctrl Pts',(-0.403107976163396,-1.,1.80012077173238));
#38286=CARTESIAN_POINT('Ctrl Pts',(-0.405933518407175,-1.,1.81223801812013));
#38287=CARTESIAN_POINT('Ctrl Pts',(-0.408428948106227,-1.,1.82247022677562));
#38288=CARTESIAN_POINT('Ctrl Pts',(-0.410641256301276,-1.,1.83100408895047));
#38289=CARTESIAN_POINT('Ctrl Pts',(-0.412633125322945,-1.,1.8380895347617));
#38290=CARTESIAN_POINT('Ctrl Pts',(-0.414487438255542,-1.,1.84405757074218));
#38291=CARTESIAN_POINT('Ctrl Pts',(-0.416300022039885,-1.,1.84929312930314));
#38292=CARTESIAN_POINT('Ctrl Pts',(-0.418164129144045,-1.,1.8541763285645));
#38293=CARTESIAN_POINT('Ctrl Pts',(-0.420157287975583,-1.,1.8590328109667));
#38294=CARTESIAN_POINT('Ctrl Pts',(-0.422327307417885,-1.,1.86408083333863));
#38295=CARTESIAN_POINT('Ctrl Pts',(-0.424678177290876,-1.,1.8693780394412));
#38296=CARTESIAN_POINT('Ctrl Pts',(-0.427183828518743,-1.,1.87486989291333));
#38297=CARTESIAN_POINT('Ctrl Pts',(-0.429803062482217,-1.,1.88044229001778));
#38298=CARTESIAN_POINT('Ctrl Pts',(-0.432493038548833,-1.,1.88596913666828));
#38299=CARTESIAN_POINT('Ctrl Pts',(-0.43522566096358,-1.,1.89136993975585));
#38300=CARTESIAN_POINT('Ctrl Pts',(-0.437995003948443,-1.,1.89663648956549));
#38301=CARTESIAN_POINT('Ctrl Pts',(-0.440807833704161,-1.,1.90180124389137));
#38302=CARTESIAN_POINT('Ctrl Pts',(-0.44367755684917,-1.,1.90691756144906));
#38303=CARTESIAN_POINT('Ctrl Pts',(-0.446617343485651,-1.,1.91203699981095));
#38304=CARTESIAN_POINT('Ctrl Pts',(-0.449632260106572,-1.,1.91718342555717));
#38305=CARTESIAN_POINT('Ctrl Pts',(-0.452719478359356,-1.,1.9223538064847));
#38306=CARTESIAN_POINT('Ctrl Pts',(-0.455872005174335,-1.,1.92753067150461));
#38307=CARTESIAN_POINT('Ctrl Pts',(-0.459081234547931,-1.,1.93269066517936));
#38308=CARTESIAN_POINT('Ctrl Pts',(-0.462340031009087,-1.,1.93781486640834));
#38309=CARTESIAN_POINT('Ctrl Pts',(-0.465645462026065,-1.,1.94289794196205));
#38310=CARTESIAN_POINT('Ctrl Pts',(-0.468997482913158,-1.,1.94794381136524));
#38311=CARTESIAN_POINT('Ctrl Pts',(-0.47239767226408,-1.,1.95296148278136));
#38312=CARTESIAN_POINT('Ctrl Pts',(-0.475848034683172,-1.,1.95796111148175));
#38313=CARTESIAN_POINT('Ctrl Pts',(-0.479349583074846,-1.,1.96294933055938));
#38314=CARTESIAN_POINT('Ctrl Pts',(-0.482901662120687,-1.,1.96792703422358));
#38315=CARTESIAN_POINT('Ctrl Pts',(-0.486502692907661,-1.,1.97289186263272));
#38316=CARTESIAN_POINT('Ctrl Pts',(-0.490150627860955,-1.,1.97783973019229));
#38317=CARTESIAN_POINT('Ctrl Pts',(-0.493843476541492,-1.,1.9827665876182));
#38318=CARTESIAN_POINT('Ctrl Pts',(-0.497579909545564,-1.,1.98767044752929));
#38319=CARTESIAN_POINT('Ctrl Pts',(-0.501359287727129,-1.,1.9925514912615));
#38320=CARTESIAN_POINT('Ctrl Pts',(-0.505181361323011,-1.,1.99741107463567));
#38321=CARTESIAN_POINT('Ctrl Pts',(-0.509046069886152,-1.,2.00225107134733));
#38322=CARTESIAN_POINT('Ctrl Pts',(-0.512953306961814,-1.,2.00707309946955));
#38323=CARTESIAN_POINT('Ctrl Pts',(-0.516902681728733,-1.,2.01187773939257));
#38324=CARTESIAN_POINT('Ctrl Pts',(-0.520893590399428,-1.,2.01666477917305));
#38325=CARTESIAN_POINT('Ctrl Pts',(-0.524925318333518,-1.,2.02143356304712));
#38326=CARTESIAN_POINT('Ctrl Pts',(-0.528997127241911,-1.,2.02618329083289));
#38327=CARTESIAN_POINT('Ctrl Pts',(-0.533108355132905,-1.,2.03091336214401));
#38328=CARTESIAN_POINT('Ctrl Pts',(-0.537258489833134,-1.,2.03562362953993));
#38329=CARTESIAN_POINT('Ctrl Pts',(-0.54144712061552,-1.,2.0403142269048));
#38330=CARTESIAN_POINT('Ctrl Pts',(-0.545673903817348,-1.,2.0449854471456));
#38331=CARTESIAN_POINT('Ctrl Pts',(-0.549938525150342,-1.,2.04963761077974));
#38332=CARTESIAN_POINT('Ctrl Pts',(-0.55424065746411,-1.,2.05427091604482));
#38333=CARTESIAN_POINT('Ctrl Pts',(-0.558579940185467,-1.,2.05888537756571));
#38334=CARTESIAN_POINT('Ctrl Pts',(-0.562955993082574,-1.,2.06348090160697));
#38335=CARTESIAN_POINT('Ctrl Pts',(-0.567368421181229,-1.,2.06805732997383));
#38336=CARTESIAN_POINT('Ctrl Pts',(-0.571816823242411,-1.,2.07261449292757));
#38337=CARTESIAN_POINT('Ctrl Pts',(-0.576300797416275,-1.,2.07715226767361));
#38338=CARTESIAN_POINT('Ctrl Pts',(-0.580819952107257,-1.,2.08167059018138));
#38339=CARTESIAN_POINT('Ctrl Pts',(-0.585373918990895,-1.,2.086169437277));
#38340=CARTESIAN_POINT('Ctrl Pts',(-0.589962365403189,-1.,2.09064881812053));
#38341=CARTESIAN_POINT('Ctrl Pts',(-0.594585006052824,-1.,2.09510876220501));
#38342=CARTESIAN_POINT('Ctrl Pts',(-0.599241616422144,-1.,2.09954930865331));
#38343=CARTESIAN_POINT('Ctrl Pts',(-0.603932030738212,-1.,2.10397049887709));
#38344=CARTESIAN_POINT('Ctrl Pts',(-0.607711315456826,-1.,2.10749199615859));
#38345=CARTESIAN_POINT('Ctrl Pts',(-0.610560911691113,-1.,2.11012443807661));
#38346=CARTESIAN_POINT('Ctrl Pts',(-0.61246736556225,-1.,2.11187554260142));
#38347=CARTESIAN_POINT('Ctrl Pts',(-0.61342227326009,-1.,2.11275013067528));
#38348=CARTESIAN_POINT('',(-0.745574324794401,-1.,2.0698113262342));
#38349=CARTESIAN_POINT('',(-0.61342227326009,-1.,2.11275013067528));
#38350=CARTESIAN_POINT('',(-0.693717979106306,-1.,1.60662857109684));
#38351=CARTESIAN_POINT('Ctrl Pts',(-0.745574324794401,-1.,2.0698113262342));
#38352=CARTESIAN_POINT('Ctrl Pts',(-0.74583279137781,-1.,2.06854248895575));
#38353=CARTESIAN_POINT('Ctrl Pts',(-0.746345871542696,-1.,2.06600523016401));
#38354=CARTESIAN_POINT('Ctrl Pts',(-0.747103932785504,-1.,2.06220058927162));
#38355=CARTESIAN_POINT('Ctrl Pts',(-0.748091554181101,-1.,2.05713023030263));
#38356=CARTESIAN_POINT('Ctrl Pts',(-0.749287468663053,-1.,2.05079645591606));
#38357=CARTESIAN_POINT('Ctrl Pts',(-0.750444657874758,-1.,2.04446689147754));
#38358=CARTESIAN_POINT('Ctrl Pts',(-0.751562963361384,-1.,2.03814160092173));
#38359=CARTESIAN_POINT('Ctrl Pts',(-0.752642180488104,-1.,2.03182068456467));
#38360=CARTESIAN_POINT('Ctrl Pts',(-0.753682061113766,-1.,2.02550428623587));
#38361=CARTESIAN_POINT('Ctrl Pts',(-0.75468233072352,-1.,2.01919259406003));
#38362=CARTESIAN_POINT('Ctrl Pts',(-0.7556427049581,-1.,2.01288584328149));
#38363=CARTESIAN_POINT('Ctrl Pts',(-0.756562904646496,-1.,2.00658431587682));
#38364=CARTESIAN_POINT('Ctrl Pts',(-0.757442676862341,-1.,2.00028834739072));
#38365=CARTESIAN_POINT('Ctrl Pts',(-0.758281796766377,-1.,1.9939983109871));
#38366=CARTESIAN_POINT('Ctrl Pts',(-0.759080037802243,-1.,1.98771456680806));
#38367=CARTESIAN_POINT('Ctrl Pts',(-0.759837147452135,-1.,1.98143741418156));
#38368=CARTESIAN_POINT('Ctrl Pts',(-0.760552825409855,-1.,1.97516705321521));
#38369=CARTESIAN_POINT('Ctrl Pts',(-0.761226690483986,-1.,1.96890351582545));
#38370=CARTESIAN_POINT('Ctrl Pts',(-0.761858300014575,-1.,1.96264672744229));
#38371=CARTESIAN_POINT('Ctrl Pts',(-0.762447203806263,-1.,1.95639665309893));
#38372=CARTESIAN_POINT('Ctrl Pts',(-0.762992990878774,-1.,1.95015342590025));
#38373=CARTESIAN_POINT('Ctrl Pts',(-0.76349533353858,-1.,1.94391746617626));
#38374=CARTESIAN_POINT('Ctrl Pts',(-0.763954049121393,-1.,1.93768964875867));
#38375=CARTESIAN_POINT('Ctrl Pts',(-0.764369010673889,-1.,1.93147105496367));
#38376=CARTESIAN_POINT('Ctrl Pts',(-0.764740025488189,-1.,1.92526263537041));
#38377=CARTESIAN_POINT('Ctrl Pts',(-0.765066729667095,-1.,1.91906491634197));
#38378=CARTESIAN_POINT('Ctrl Pts',(-0.765348465884739,-1.,1.91287765805174));
#38379=CARTESIAN_POINT('Ctrl Pts',(-0.765584196937936,-1.,1.90669961402362));
#38380=CARTESIAN_POINT('Ctrl Pts',(-0.765772772593395,-1.,1.90052930393599));
#38381=CARTESIAN_POINT('Ctrl Pts',(-0.765913193856979,-1.,1.89436577771389));
#38382=CARTESIAN_POINT('Ctrl Pts',(-0.76600483706209,-1.,1.88820926433409));
#38383=CARTESIAN_POINT('Ctrl Pts',(-0.766047794851869,-1.,1.88206215302561));
#38384=CARTESIAN_POINT('Ctrl Pts',(-0.766042837036759,-1.,1.87592888967886));
#38385=CARTESIAN_POINT('Ctrl Pts',(-0.765990708546111,-1.,1.86981398314345));
#38386=CARTESIAN_POINT('Ctrl Pts',(-0.765891519092557,-1.,1.86372027063314));
#38387=CARTESIAN_POINT('Ctrl Pts',(-0.765744212909305,-1.,1.85764741390391));
#38388=CARTESIAN_POINT('Ctrl Pts',(-0.765545710619023,-1.,1.85158945130054));
#38389=CARTESIAN_POINT('Ctrl Pts',(-0.765291664861971,-1.,1.8455369887591));
#38390=CARTESIAN_POINT('Ctrl Pts',(-0.764978057881687,-1.,1.83948181064823));
#38391=CARTESIAN_POINT('Ctrl Pts',(-0.764602549687845,-1.,1.8334207722714));
#38392=CARTESIAN_POINT('Ctrl Pts',(-0.764165902606055,-1.,1.8273599120008));
#38393=CARTESIAN_POINT('Ctrl Pts',(-0.763673465462854,-1.,1.82131873145297));
#38394=CARTESIAN_POINT('Ctrl Pts',(-0.763132003836783,-1.,1.81532118405566));
#38395=CARTESIAN_POINT('Ctrl Pts',(-0.762546129464036,-1.,1.80938551463989));
#38396=CARTESIAN_POINT('Ctrl Pts',(-0.761915336443516,-1.,1.80351583877334));
#38397=CARTESIAN_POINT('Ctrl Pts',(-0.761229695230359,-1.,1.79768986997735));
#38398=CARTESIAN_POINT('Ctrl Pts',(-0.760469555880425,-1.,1.79185815610802));
#38399=CARTESIAN_POINT('Ctrl Pts',(-0.759614401109868,-1.,1.78596964884526));
#38400=CARTESIAN_POINT('Ctrl Pts',(-0.75865062667738,-1.,1.77999411220912));
#38401=CARTESIAN_POINT('Ctrl Pts',(-0.757578264077238,-1.,1.77394167108342));
#38402=CARTESIAN_POINT('Ctrl Pts',(-0.756421896028403,-1.,1.76789396003141));
#38403=CARTESIAN_POINT('Ctrl Pts',(-0.755220979975262,-1.,1.7619781724032));
#38404=CARTESIAN_POINT('Ctrl Pts',(-0.75400925402848,-1.,1.75631083600175));
#38405=CARTESIAN_POINT('Ctrl Pts',(-0.752797683531377,-1.,1.75095139468809));
#38406=CARTESIAN_POINT('Ctrl Pts',(-0.751555614163629,-1.,1.74585086852298));
#38407=CARTESIAN_POINT('Ctrl Pts',(-0.75019343597954,-1.,1.74080458266705));
#38408=CARTESIAN_POINT('Ctrl Pts',(-0.748582462954855,-1.,1.73550351679848));
#38409=CARTESIAN_POINT('Ctrl Pts',(-0.746574710096436,-1.,1.72958533647399));
#38410=CARTESIAN_POINT('Ctrl Pts',(-0.744021445433764,-1.,1.7226822991693));
#38411=CARTESIAN_POINT('Ctrl Pts',(-0.740795162032088,-1.,1.71447789751927));
#38412=CARTESIAN_POINT('Ctrl Pts',(-0.736799665724771,-1.,1.70473309006121));
#38413=CARTESIAN_POINT('Ctrl Pts',(-0.731963238697195,-1.,1.69326921975743));
#38414=CARTESIAN_POINT('Ctrl Pts',(-0.726235967997433,-1.,1.67996158455503));
#38415=CARTESIAN_POINT('Ctrl Pts',(-0.719585433804282,-1.,1.6647288055568));
#38416=CARTESIAN_POINT('Ctrl Pts',(-0.711993139355394,-1.,1.64752408832016));
#38417=CARTESIAN_POINT('Ctrl Pts',(-0.705159151988319,-1.,1.63216541664676));
#38418=CARTESIAN_POINT('Ctrl Pts',(-0.699605146405088,-1.,1.61974673472612));
#38419=CARTESIAN_POINT('Ctrl Pts',(-0.695712097881194,-1.,1.61106790958151));
#38420=CARTESIAN_POINT('Ctrl Pts',(-0.693717979106306,-1.,1.60662857109684));
#38421=CARTESIAN_POINT('',(-0.892032620296855,-1.,1.5055822144029));
#38422=CARTESIAN_POINT('Origin',(0.,-1.,0.));
#38423=CARTESIAN_POINT('',(-1.23627494547115,-1.,1.81978687191668));
#38424=CARTESIAN_POINT('Ctrl Pts',(-0.892032620296855,-1.,1.5055822144029));
#38425=CARTESIAN_POINT('Ctrl Pts',(-0.894452006964543,-1.,1.50980486806688));
#38426=CARTESIAN_POINT('Ctrl Pts',(-0.899185047483511,-1.,1.51805569590094));
#38427=CARTESIAN_POINT('Ctrl Pts',(-0.905967409625651,-1.,1.52984849887993));
#38428=CARTESIAN_POINT('Ctrl Pts',(-0.914375919026456,-1.,1.54440491149498));
#38429=CARTESIAN_POINT('Ctrl Pts',(-0.923832188944341,-1.,1.56065988578893));
#38430=CARTESIAN_POINT('Ctrl Pts',(-0.932246680108685,-1.,1.57499388382243));
#38431=CARTESIAN_POINT('Ctrl Pts',(-0.939646377893399,-1.,1.58744937487176));
#38432=CARTESIAN_POINT('Ctrl Pts',(-0.946078063315257,-1.,1.59810042043673));
#38433=CARTESIAN_POINT('Ctrl Pts',(-0.951613284356035,-1.,1.60706069896936));
#38434=CARTESIAN_POINT('Ctrl Pts',(-0.956354422920671,-1.,1.61449324337085));
#38435=CARTESIAN_POINT('Ctrl Pts',(-0.960438326101729,-1.,1.62061638140221));
#38436=CARTESIAN_POINT('Ctrl Pts',(-0.964046107040536,-1.,1.62571930670187));
#38437=CARTESIAN_POINT('Ctrl Pts',(-0.967387853230345,-1.,1.63013849959461));
#38438=CARTESIAN_POINT('Ctrl Pts',(-0.970669715997509,-1.,1.63420665729798));
#38439=CARTESIAN_POINT('Ctrl Pts',(-0.974066058287418,-1.,1.63820952658144));
#38440=CARTESIAN_POINT('Ctrl Pts',(-0.977689794119416,-1.,1.64233990826687));
#38441=CARTESIAN_POINT('Ctrl Pts',(-0.981562530939489,-1.,1.64665139190656));
#38442=CARTESIAN_POINT('Ctrl Pts',(-0.985642622920821,-1.,1.65110016612638));
#38443=CARTESIAN_POINT('Ctrl Pts',(-0.989855627854165,-1.,1.65559044289699));
#38444=CARTESIAN_POINT('Ctrl Pts',(-0.994121836661306,-1.,1.66001553809947));
#38445=CARTESIAN_POINT('Ctrl Pts',(-0.998389654952758,-1.,1.66430758030376));
#38446=CARTESIAN_POINT('Ctrl Pts',(-1.00265091003727,-1.,1.66846059277303));
#38447=CARTESIAN_POINT('Ctrl Pts',(-1.00692206696414,-1.,1.67250335383293));
#38448=CARTESIAN_POINT('Ctrl Pts',(-1.01123236493511,-1.,1.67648246776464));
#38449=CARTESIAN_POINT('Ctrl Pts',(-1.01561026162773,-1.,1.68044289894798));
#38450=CARTESIAN_POINT('Ctrl Pts',(-1.02006795074201,-1.,1.68440578021706));
#38451=CARTESIAN_POINT('Ctrl Pts',(-1.02460180535255,-1.,1.68836910178447));
#38452=CARTESIAN_POINT('Ctrl Pts',(-1.02919977579147,-1.,1.69231840863458));
#38453=CARTESIAN_POINT('Ctrl Pts',(-1.03384646003588,-1.,1.69623414782771));
#38454=CARTESIAN_POINT('Ctrl Pts',(-1.03852922490789,-1.,1.70010052930962));
#38455=CARTESIAN_POINT('Ctrl Pts',(-1.04324363334554,-1.,1.70391338707982));
#38456=CARTESIAN_POINT('Ctrl Pts',(-1.04799085404995,-1.,1.70767646263649));
#38457=CARTESIAN_POINT('Ctrl Pts',(-1.05277517202855,-1.,1.71139783543989));
#38458=CARTESIAN_POINT('Ctrl Pts',(-1.05760163192479,-1.,1.7150865442702));
#38459=CARTESIAN_POINT('Ctrl Pts',(-1.06247324680647,-1.,1.71874858456904));
#38460=CARTESIAN_POINT('Ctrl Pts',(-1.06738966975462,-1.,1.72238500928453));
#38461=CARTESIAN_POINT('Ctrl Pts',(-1.07234866990252,-1.,1.72599406198488));
#38462=CARTESIAN_POINT('Ctrl Pts',(-1.0773470373727,-1.,1.72957248977424));
#38463=CARTESIAN_POINT('Ctrl Pts',(-1.08238162784749,-1.,1.73311705663407));
#38464=CARTESIAN_POINT('Ctrl Pts',(-1.08745056285427,-1.,1.73662628326091));
#38465=CARTESIAN_POINT('Ctrl Pts',(-1.09255329056493,-1.,1.74010053962247));
#38466=CARTESIAN_POINT('Ctrl Pts',(-1.09768999241225,-1.,1.74354119236208));
#38467=CARTESIAN_POINT('Ctrl Pts',(-1.10286118991143,-1.,1.74695004214923));
#38468=CARTESIAN_POINT('Ctrl Pts',(-1.10806728183007,-1.,1.7503286607592));
#38469=CARTESIAN_POINT('Ctrl Pts',(-1.11330807582551,-1.,1.7536777209463));
#38470=CARTESIAN_POINT('Ctrl Pts',(-1.11858293216763,-1.,1.75699720772105));
#38471=CARTESIAN_POINT('Ctrl Pts',(-1.12389096855086,-1.,1.76028671825096));
#38472=CARTESIAN_POINT('Ctrl Pts',(-1.12923123555075,-1.,1.7635457196617));
#38473=CARTESIAN_POINT('Ctrl Pts',(-1.1346029180462,-1.,1.76677384551862));
#38474=CARTESIAN_POINT('Ctrl Pts',(-1.14000548336975,-1.,1.76997111386769));
#38475=CARTESIAN_POINT('Ctrl Pts',(-1.1454385822692,-1.,1.77313777896194));
#38476=CARTESIAN_POINT('Ctrl Pts',(-1.15090197841515,-1.,1.7762742255701));
#38477=CARTESIAN_POINT('Ctrl Pts',(-1.15639547194698,-1.,1.77938085564275));
#38478=CARTESIAN_POINT('Ctrl Pts',(-1.16191881298499,-1.,1.78245795881009));
#38479=CARTESIAN_POINT('Ctrl Pts',(-1.16747166312303,-1.,1.78550566040443));
#38480=CARTESIAN_POINT('Ctrl Pts',(-1.17305363177328,-1.,1.78852398877616));
#38481=CARTESIAN_POINT('Ctrl Pts',(-1.17866429440809,-1.,1.79151291552689));
#38482=CARTESIAN_POINT('Ctrl Pts',(-1.18430321697432,-1.,1.79447240321515));
#38483=CARTESIAN_POINT('Ctrl Pts',(-1.18996997934445,-1.,1.79740245923478));
#38484=CARTESIAN_POINT('Ctrl Pts',(-1.19566418930242,-1.,1.80030314369879));
#38485=CARTESIAN_POINT('Ctrl Pts',(-1.20138548938974,-1.,1.80317454838603));
#38486=CARTESIAN_POINT('Ctrl Pts',(-1.20713356605475,-1.,1.80601678480707));
#38487=CARTESIAN_POINT('Ctrl Pts',(-1.21290815708314,-1.,1.80882996917129));
#38488=CARTESIAN_POINT('Ctrl Pts',(-1.21870906103557,-1.,1.81161420806656));
#38489=CARTESIAN_POINT('Ctrl Pts',(-1.2245361330495,-1.,1.81436959210434));
#38490=CARTESIAN_POINT('Ctrl Pts',(-1.2292186489137,-1.,1.8165508718364));
#38491=CARTESIAN_POINT('Ctrl Pts',(-1.2327422452705,-1.,1.81817389921279));
#38492=CARTESIAN_POINT('Ctrl Pts',(-1.23509651170476,-1.,1.81925017193666));
#38493=CARTESIAN_POINT('Ctrl Pts',(-1.23627494547115,-1.,1.81978687191668));
#38494=CARTESIAN_POINT('',(-1.34869019493419,-1.,1.73811241238545));
#38495=CARTESIAN_POINT('',(-1.23627494547115,-1.,1.81978687191668));
#38496=CARTESIAN_POINT('',(-1.15624053661742,-1.,1.31362392696032));
#38497=CARTESIAN_POINT('Ctrl Pts',(-1.34869019493419,-1.,1.73811241238545));
#38498=CARTESIAN_POINT('Ctrl Pts',(-1.34854391898045,-1.,1.73682580585691));
#38499=CARTESIAN_POINT('Ctrl Pts',(-1.34824783112887,-1.,1.73425417885907));
#38500=CARTESIAN_POINT('Ctrl Pts',(-1.34779309152035,-1.,1.7304014965394));
#38501=CARTESIAN_POINT('Ctrl Pts',(-1.34716554819527,-1.,1.72527410680674));
#38502=CARTESIAN_POINT('Ctrl Pts',(-1.34634568653227,-1.,1.7188807715049));
#38503=CARTESIAN_POINT('Ctrl Pts',(-1.34549029589416,-1.,1.71250340686822));
#38504=CARTESIAN_POINT('Ctrl Pts',(-1.34459924533831,-1.,1.70614212266738));
#38505=CARTESIAN_POINT('Ctrl Pts',(-1.34367237124483,-1.,1.69979707754427));
#38506=CARTESIAN_POINT('Ctrl Pts',(-1.34270948206319,-1.,1.6934684849687));
#38507=CARTESIAN_POINT('Ctrl Pts',(-1.341710374848,-1.,1.68715660868764));
#38508=CARTESIAN_POINT('Ctrl Pts',(-1.34067485185203,-1.,1.68086176030362));
#38509=CARTESIAN_POINT('Ctrl Pts',(-1.3396027347034,-1.,1.67458429426086));
#38510=CARTESIAN_POINT('Ctrl Pts',(-1.33849388654388,-1.,1.66832460783989));
#38511=CARTESIAN_POINT('Ctrl Pts',(-1.33734820885262,-1.,1.66208312541983));
#38512=CARTESIAN_POINT('Ctrl Pts',(-1.33616559745172,-1.,1.65586025952593));
#38513=CARTESIAN_POINT('Ctrl Pts',(-1.33494590467993,-1.,1.6496563728683));
#38514=CARTESIAN_POINT('Ctrl Pts',(-1.33368890676572,-1.,1.6434717485603));
#38515=CARTESIAN_POINT('Ctrl Pts',(-1.33239425103724,-1.,1.63730653475089));
#38516=CARTESIAN_POINT('Ctrl Pts',(-1.33106149345645,-1.,1.63116079730923));
#38517=CARTESIAN_POINT('Ctrl Pts',(-1.3296901950568,-1.,1.62503464209797));
#38518=CARTESIAN_POINT('Ctrl Pts',(-1.32828000610449,-1.,1.61892832270724));
#38519=CARTESIAN_POINT('Ctrl Pts',(-1.32683074483356,-1.,1.6128423401575));
#38520=CARTESIAN_POINT('Ctrl Pts',(-1.32534250785782,-1.,1.60677758290954));
#38521=CARTESIAN_POINT('Ctrl Pts',(-1.32381550858256,-1.,1.60073511858687));
#38522=CARTESIAN_POINT('Ctrl Pts',(-1.32224985747682,-1.,1.59471591079403));
#38523=CARTESIAN_POINT('Ctrl Pts',(-1.32064537110892,-1.,1.58872057258245));
#38524=CARTESIAN_POINT('Ctrl Pts',(-1.31900135021432,-1.,1.58274907898834));
#38525=CARTESIAN_POINT('Ctrl Pts',(-1.31731642317187,-1.,1.5768005650559));
#38526=CARTESIAN_POINT('Ctrl Pts',(-1.31558903860016,-1.,1.57087397835723));
#38527=CARTESIAN_POINT('Ctrl Pts',(-1.31381795281002,-1.,1.56496872402353));
#38528=CARTESIAN_POINT('Ctrl Pts',(-1.31200264341696,-1.,1.55908521254821));
#38529=CARTESIAN_POINT('Ctrl Pts',(-1.31014393684222,-1.,1.55322568759481));
#38530=CARTESIAN_POINT('Ctrl Pts',(-1.30824393907473,-1.,1.54739413957185));
#38531=CARTESIAN_POINT('Ctrl Pts',(-1.30630475189556,-1.,1.54159462645432));
#38532=CARTESIAN_POINT('Ctrl Pts',(-1.30432735639489,-1.,1.53582981268977));
#38533=CARTESIAN_POINT('Ctrl Pts',(-1.30231064395568,-1.,1.53009970283891));
#38534=CARTESIAN_POINT('Ctrl Pts',(-1.30024984366328,-1.,1.52439957861062));
#38535=CARTESIAN_POINT('Ctrl Pts',(-1.29813791800747,-1.,1.51872184912724));
#38536=CARTESIAN_POINT('Ctrl Pts',(-1.29596850710509,-1.,1.51305994241402));
#38537=CARTESIAN_POINT('Ctrl Pts',(-1.29373841372842,-1.,1.50741159078365));
#38538=CARTESIAN_POINT('Ctrl Pts',(-1.29145022885181,-1.,1.50178230149776));
#38539=CARTESIAN_POINT('Ctrl Pts',(-1.28911506584254,-1.,1.49618896881754));
#38540=CARTESIAN_POINT('Ctrl Pts',(-1.2867467611644,-1.,1.4906522831278));
#38541=CARTESIAN_POINT('Ctrl Pts',(-1.28435533880201,-1.,1.4851881711891));
#38542=CARTESIAN_POINT('Ctrl Pts',(-1.28194158939517,-1.,1.47980070347095));
#38543=CARTESIAN_POINT('Ctrl Pts',(-1.2794891824849,-1.,1.4744717526707));
#38544=CARTESIAN_POINT('Ctrl Pts',(-1.27696414831089,-1.,1.46916035917133));
#38545=CARTESIAN_POINT('Ctrl Pts',(-1.27433119897822,-1.,1.46382431332476));
#38546=CARTESIAN_POINT('Ctrl Pts',(-1.27156805265289,-1.,1.45843906294697));
#38547=CARTESIAN_POINT('Ctrl Pts',(-1.2686778680489,-1.,1.45301422764247));
#38548=CARTESIAN_POINT('Ctrl Pts',(-1.26570925118868,-1.,1.44761985001662));
#38549=CARTESIAN_POINT('Ctrl Pts',(-1.26273903323859,-1.,1.44236470511303));
#38550=CARTESIAN_POINT('Ctrl Pts',(-1.25983531012005,-1.,1.43734919180848));
#38551=CARTESIAN_POINT('Ctrl Pts',(-1.25702687965755,-1.,1.43262645609691));
#38552=CARTESIAN_POINT('Ctrl Pts',(-1.25426945222639,-1.,1.42815938799387));
#38553=CARTESIAN_POINT('Ctrl Pts',(-1.2514145557001,-1.,1.42378102115575));
#38554=CARTESIAN_POINT('Ctrl Pts',(-1.24824430986571,-1.,1.41923722596025));
#38555=CARTESIAN_POINT('Ctrl Pts',(-1.24450600513056,-1.,1.41422913175179));
#38556=CARTESIAN_POINT('Ctrl Pts',(-1.23994455029534,-1.,1.40845295531283));
#38557=CARTESIAN_POINT('Ctrl Pts',(-1.23434087290423,-1.,1.40164708206106));
#38558=CARTESIAN_POINT('Ctrl Pts',(-1.22752961899387,-1.,1.39361389568796));
#38559=CARTESIAN_POINT('Ctrl Pts',(-1.21938737280852,-1.,1.38420564527715));
#38560=CARTESIAN_POINT('Ctrl Pts',(-1.20982812925645,-1.,1.37331915607905));
#38561=CARTESIAN_POINT('Ctrl Pts',(-1.1987959077932,-1.,1.36088705043885));
#38562=CARTESIAN_POINT('Ctrl Pts',(-1.18625865667441,-1.,1.34687054001093));
#38563=CARTESIAN_POINT('Ctrl Pts',(-1.17501305789857,-1.,1.33437539347008));
#38564=CARTESIAN_POINT('Ctrl Pts',(-1.16589330093588,-1.,1.32428080721772));
#38565=CARTESIAN_POINT('Ctrl Pts',(-1.15950888730809,-1.,1.31722977216397));
#38566=CARTESIAN_POINT('Ctrl Pts',(-1.15624053661742,-1.,1.31362392696032));
#38567=CARTESIAN_POINT('',(-1.31362392696033,-1.,1.15624053661742));
#38568=CARTESIAN_POINT('Origin',(0.,-1.,0.));
#38569=CARTESIAN_POINT('',(-1.73811241238545,-1.,1.34869019493419));
#38570=CARTESIAN_POINT('Ctrl Pts',(-1.31362392696033,-1.,1.15624053661742));
#38571=CARTESIAN_POINT('Ctrl Pts',(-1.3172297721596,-1.,1.15950888730433));
#38572=CARTESIAN_POINT('Ctrl Pts',(-1.32428080720544,-1.,1.16589330092532));
#38573=CARTESIAN_POINT('Ctrl Pts',(-1.33437539344842,-1.,1.17501305787994));
#38574=CARTESIAN_POINT('Ctrl Pts',(-1.34687053998157,-1.,1.18625865664915));
#38575=CARTESIAN_POINT('Ctrl Pts',(-1.36088705040677,-1.,1.1987959077656));
#38576=CARTESIAN_POINT('Ctrl Pts',(-1.37331915604962,-1.,1.20982812923113));
#38577=CARTESIAN_POINT('Ctrl Pts',(-1.38420564525391,-1.,1.21938737278853));
#38578=CARTESIAN_POINT('Ctrl Pts',(-1.39361389567257,-1.,1.22752961898063));
#38579=CARTESIAN_POINT('Ctrl Pts',(-1.40164708205345,-1.,1.23434087289768));
#38580=CARTESIAN_POINT('Ctrl Pts',(-1.40845295531151,-1.,1.23994455029421));
#38581=CARTESIAN_POINT('Ctrl Pts',(-1.41422913175437,-1.,1.24450600513278));
#38582=CARTESIAN_POINT('Ctrl Pts',(-1.41923722596421,-1.,1.24824430986911));
#38583=CARTESIAN_POINT('Ctrl Pts',(-1.42378102115911,-1.,1.25141455570299));
#38584=CARTESIAN_POINT('Ctrl Pts',(-1.42815938799555,-1.,1.25426945222783));
#38585=CARTESIAN_POINT('Ctrl Pts',(-1.43262645609679,-1.,1.25702687965744));
#38586=CARTESIAN_POINT('Ctrl Pts',(-1.43734919180719,-1.,1.25983531011894));
#38587=CARTESIAN_POINT('Ctrl Pts',(-1.44236470511145,-1.,1.26273903323723));
#38588=CARTESIAN_POINT('Ctrl Pts',(-1.44761985001544,-1.,1.26570925118767));
#38589=CARTESIAN_POINT('Ctrl Pts',(-1.45301422764205,-1.,1.26867786804854));
#38590=CARTESIAN_POINT('Ctrl Pts',(-1.45843906294725,-1.,1.27156805265312));
#38591=CARTESIAN_POINT('Ctrl Pts',(-1.4638243133254,-1.,1.27433119897877));
#38592=CARTESIAN_POINT('Ctrl Pts',(-1.46916035917197,-1.,1.27696414831144));
#38593=CARTESIAN_POINT('Ctrl Pts',(-1.4744717526711,-1.,1.27948918248524));
#38594=CARTESIAN_POINT('Ctrl Pts',(-1.47980070347102,-1.,1.28194158939522));
#38595=CARTESIAN_POINT('Ctrl Pts',(-1.48518817118891,-1.,1.28435533880184));
#38596=CARTESIAN_POINT('Ctrl Pts',(-1.4906522831275,-1.,1.28674676116415));
#38597=CARTESIAN_POINT('Ctrl Pts',(-1.49618896881729,-1.,1.28911506584232));
#38598=CARTESIAN_POINT('Ctrl Pts',(-1.50178230149764,-1.,1.29145022885171));
#38599=CARTESIAN_POINT('Ctrl Pts',(-1.50741159078367,-1.,1.29373841372843));
#38600=CARTESIAN_POINT('Ctrl Pts',(-1.51305994241412,-1.,1.29596850710518));
#38601=CARTESIAN_POINT('Ctrl Pts',(-1.51872184912735,-1.,1.29813791800757));
#38602=CARTESIAN_POINT('Ctrl Pts',(-1.5243995786107,-1.,1.30024984366334));
#38603=CARTESIAN_POINT('Ctrl Pts',(-1.53009970283893,-1.,1.3023106439557));
#38604=CARTESIAN_POINT('Ctrl Pts',(-1.53582981268976,-1.,1.30432735639487));
#38605=CARTESIAN_POINT('Ctrl Pts',(-1.54159462645428,-1.,1.30630475189553));
#38606=CARTESIAN_POINT('Ctrl Pts',(-1.54739413957183,-1.,1.30824393907471));
#38607=CARTESIAN_POINT('Ctrl Pts',(-1.55322568759481,-1.,1.31014393684221));
#38608=CARTESIAN_POINT('Ctrl Pts',(-1.55908521254822,-1.,1.31200264341696));
#38609=CARTESIAN_POINT('Ctrl Pts',(-1.56496872402352,-1.,1.31381795281002));
#38610=CARTESIAN_POINT('Ctrl Pts',(-1.57087397835721,-1.,1.31558903860015));
#38611=CARTESIAN_POINT('Ctrl Pts',(-1.57680056505585,-1.,1.31731642317183));
#38612=CARTESIAN_POINT('Ctrl Pts',(-1.58274907898829,-1.,1.31900135021428));
#38613=CARTESIAN_POINT('Ctrl Pts',(-1.58872057258244,-1.,1.32064537110891));
#38614=CARTESIAN_POINT('Ctrl Pts',(-1.59471591079408,-1.,1.32224985747686));
#38615=CARTESIAN_POINT('Ctrl Pts',(-1.600735118587,-1.,1.32381550858266));
#38616=CARTESIAN_POINT('Ctrl Pts',(-1.6067775829097,-1.,1.32534250785794));
#38617=CARTESIAN_POINT('Ctrl Pts',(-1.61284234015762,-1.,1.32683074483365));
#38618=CARTESIAN_POINT('Ctrl Pts',(-1.61892832270723,-1.,1.32828000610448));
#38619=CARTESIAN_POINT('Ctrl Pts',(-1.62503464209777,-1.,1.32969019505665));
#38620=CARTESIAN_POINT('Ctrl Pts',(-1.63116079730887,-1.,1.33106149345618));
#38621=CARTESIAN_POINT('Ctrl Pts',(-1.6373065347505,-1.,1.33239425103694));
#38622=CARTESIAN_POINT('Ctrl Pts',(-1.64347174856007,-1.,1.33368890676554));
#38623=CARTESIAN_POINT('Ctrl Pts',(-1.64965637286843,-1.,1.33494590468003));
#38624=CARTESIAN_POINT('Ctrl Pts',(-1.65586025952651,-1.,1.33616559745217));
#38625=CARTESIAN_POINT('Ctrl Pts',(-1.66208312542073,-1.,1.33734820885331));
#38626=CARTESIAN_POINT('Ctrl Pts',(-1.66832460784078,-1.,1.33849388654458));
#38627=CARTESIAN_POINT('Ctrl Pts',(-1.67458429426126,-1.,1.33960273470372));
#38628=CARTESIAN_POINT('Ctrl Pts',(-1.68086176030308,-1.,1.3406748518516));
#38629=CARTESIAN_POINT('Ctrl Pts',(-1.68715660868602,-1.,1.34171037484673));
#38630=CARTESIAN_POINT('Ctrl Pts',(-1.6934684849664,-1.,1.34270948206139));
#38631=CARTESIAN_POINT('Ctrl Pts',(-1.69979707754221,-1.,1.34367237124322));
#38632=CARTESIAN_POINT('Ctrl Pts',(-1.70614212266676,-1.,1.34459924533783));
#38633=CARTESIAN_POINT('Ctrl Pts',(-1.71250340687011,-1.,1.34549029589563));
#38634=CARTESIAN_POINT('Ctrl Pts',(-1.7188807715095,-1.,1.34634568653586));
#38635=CARTESIAN_POINT('Ctrl Pts',(-1.72527410681298,-1.,1.34716554820013));
#38636=CARTESIAN_POINT('Ctrl Pts',(-1.73040149654497,-1.,1.3477930915247));
#38637=CARTESIAN_POINT('Ctrl Pts',(-1.73425417886255,-1.,1.34824783113158));
#38638=CARTESIAN_POINT('Ctrl Pts',(-1.73682580585819,-1.,1.34854391898145));
#38639=CARTESIAN_POINT('Ctrl Pts',(-1.73811241238545,-1.,1.34869019493419));
#38640=CARTESIAN_POINT('',(-1.81978687191668,-1.,1.23627494547115));
#38641=CARTESIAN_POINT('',(-1.73811241238545,-1.,1.34869019493419));
#38642=CARTESIAN_POINT('',(-1.5055822144029,-1.,0.892032620296855));
#38643=CARTESIAN_POINT('Ctrl Pts',(-1.81978687191668,-1.,1.23627494547115));
#38644=CARTESIAN_POINT('Ctrl Pts',(-1.81925017193531,-1.,1.23509651170384));
#38645=CARTESIAN_POINT('Ctrl Pts',(-1.81817389920914,-1.,1.23274224526804));
#38646=CARTESIAN_POINT('Ctrl Pts',(-1.81655087183054,-1.,1.22921864890975));
#38647=CARTESIAN_POINT('Ctrl Pts',(-1.81436959209778,-1.,1.22453613304507));
#38648=CARTESIAN_POINT('Ctrl Pts',(-1.81161420806172,-1.,1.2187090610323));
#38649=CARTESIAN_POINT('Ctrl Pts',(-1.80882996916931,-1.,1.2129081570818));
#38650=CARTESIAN_POINT('Ctrl Pts',(-1.80601678480772,-1.,1.20713356605519));
#38651=CARTESIAN_POINT('Ctrl Pts',(-1.8031745483882,-1.,1.2013854893912));
#38652=CARTESIAN_POINT('Ctrl Pts',(-1.80030314370121,-1.,1.19566418930405));
#38653=CARTESIAN_POINT('Ctrl Pts',(-1.79740245923649,-1.,1.1899699793456));
#38654=CARTESIAN_POINT('Ctrl Pts',(-1.79447240321572,-1.,1.18430321697471));
#38655=CARTESIAN_POINT('Ctrl Pts',(-1.79151291552646,-1.,1.17866429440781));
#38656=CARTESIAN_POINT('Ctrl Pts',(-1.78852398877523,-1.,1.17305363177265));
#38657=CARTESIAN_POINT('Ctrl Pts',(-1.78550566040349,-1.,1.16747166312239));
#38658=CARTESIAN_POINT('Ctrl Pts',(-1.78245795880949,-1.,1.16191881298458));
#38659=CARTESIAN_POINT('Ctrl Pts',(-1.77938085564261,-1.,1.15639547194689));
#38660=CARTESIAN_POINT('Ctrl Pts',(-1.77627422557034,-1.,1.15090197841531));
#38661=CARTESIAN_POINT('Ctrl Pts',(-1.77313777896234,-1.,1.14543858226948));
#38662=CARTESIAN_POINT('Ctrl Pts',(-1.76997111386806,-1.,1.14000548337));
#38663=CARTESIAN_POINT('Ctrl Pts',(-1.76677384551883,-1.,1.13460291804635));
#38664=CARTESIAN_POINT('Ctrl Pts',(-1.76354571966171,-1.,1.12923123555076));
#38665=CARTESIAN_POINT('Ctrl Pts',(-1.76028671825084,-1.,1.12389096855078));
#38666=CARTESIAN_POINT('Ctrl Pts',(-1.75699720772089,-1.,1.11858293216752));
#38667=CARTESIAN_POINT('Ctrl Pts',(-1.75367772094617,-1.,1.11330807582542));
#38668=CARTESIAN_POINT('Ctrl Pts',(-1.75032866075914,-1.,1.10806728183003));
#38669=CARTESIAN_POINT('Ctrl Pts',(-1.74695004214924,-1.,1.10286118991144));
#38670=CARTESIAN_POINT('Ctrl Pts',(-1.74354119236212,-1.,1.09768999241229));
#38671=CARTESIAN_POINT('Ctrl Pts',(-1.74010053962252,-1.,1.09255329056496));
#38672=CARTESIAN_POINT('Ctrl Pts',(-1.73662628326093,-1.,1.08745056285429));
#38673=CARTESIAN_POINT('Ctrl Pts',(-1.73311705663407,-1.,1.08238162784749));
#38674=CARTESIAN_POINT('Ctrl Pts',(-1.72957248977424,-1.,1.0773470373727));
#38675=CARTESIAN_POINT('Ctrl Pts',(-1.72599406198489,-1.,1.07234866990252));
#38676=CARTESIAN_POINT('Ctrl Pts',(-1.72238500928456,-1.,1.06738966975463));
#38677=CARTESIAN_POINT('Ctrl Pts',(-1.71874858456908,-1.,1.0624732468065));
#38678=CARTESIAN_POINT('Ctrl Pts',(-1.71508654427022,-1.,1.05760163192481));
#38679=CARTESIAN_POINT('Ctrl Pts',(-1.71139783543986,-1.,1.05277517202854));
#38680=CARTESIAN_POINT('Ctrl Pts',(-1.70767646263641,-1.,1.0479908540499));
#38681=CARTESIAN_POINT('Ctrl Pts',(-1.70391338707969,-1.,1.04324363334546));
#38682=CARTESIAN_POINT('Ctrl Pts',(-1.70010052930951,-1.,1.03852922490782));
#38683=CARTESIAN_POINT('Ctrl Pts',(-1.69623414782769,-1.,1.03384646003587));
#38684=CARTESIAN_POINT('Ctrl Pts',(-1.69231840863471,-1.,1.02919977579155));
#38685=CARTESIAN_POINT('Ctrl Pts',(-1.68836910178475,-1.,1.02460180535272));
#38686=CARTESIAN_POINT('Ctrl Pts',(-1.68440578021739,-1.,1.02006795074222));
#38687=CARTESIAN_POINT('Ctrl Pts',(-1.6804428989482,-1.,1.01561026162787));
#38688=CARTESIAN_POINT('Ctrl Pts',(-1.67648246776457,-1.,1.01123236493507));
#38689=CARTESIAN_POINT('Ctrl Pts',(-1.67250335383248,-1.,1.00692206696387));
#38690=CARTESIAN_POINT('Ctrl Pts',(-1.66846059277231,-1.,1.00265091003682));
#38691=CARTESIAN_POINT('Ctrl Pts',(-1.66430758030304,-1.,0.998389654952317));
#38692=CARTESIAN_POINT('Ctrl Pts',(-1.66001553809916,-1.,0.994121836661116));
#38693=CARTESIAN_POINT('Ctrl Pts',(-1.65559044289746,-1.,0.98985562785445));
#38694=CARTESIAN_POINT('Ctrl Pts',(-1.6511001661277,-1.,0.985642622921626));
#38695=CARTESIAN_POINT('Ctrl Pts',(-1.64665139190834,-1.,0.981562530940574));
#38696=CARTESIAN_POINT('Ctrl Pts',(-1.64233990826831,-1.,0.977689794120297));
#38697=CARTESIAN_POINT('Ctrl Pts',(-1.63820952658157,-1.,0.974066058287501));
#38698=CARTESIAN_POINT('Ctrl Pts',(-1.63420665729609,-1.,0.970669715996356));
#38699=CARTESIAN_POINT('Ctrl Pts',(-1.63013849959083,-1.,0.967387853228041));
#38700=CARTESIAN_POINT('Ctrl Pts',(-1.6257193066974,-1.,0.964046107037821));
#38701=CARTESIAN_POINT('Ctrl Pts',(-1.62061638139929,-1.,0.960438326099958));
#38702=CARTESIAN_POINT('Ctrl Pts',(-1.61449324337233,-1.,0.956354422921573));
#38703=CARTESIAN_POINT('Ctrl Pts',(-1.60706069897794,-1.,0.951613284361248));
#38704=CARTESIAN_POINT('Ctrl Pts',(-1.59810042045408,-1.,0.946078063325796));
#38705=CARTESIAN_POINT('Ctrl Pts',(-1.58744937489796,-1.,0.939646377909319));
#38706=CARTESIAN_POINT('Ctrl Pts',(-1.57499388385561,-1.,0.932246680128849));
#38707=CARTESIAN_POINT('Ctrl Pts',(-1.56065988582509,-1.,0.923832188966322));
#38708=CARTESIAN_POINT('Ctrl Pts',(-1.54440491152808,-1.,0.91437591904658));
#38709=CARTESIAN_POINT('Ctrl Pts',(-1.52984849890434,-1.,0.905967409640499));
#38710=CARTESIAN_POINT('Ctrl Pts',(-1.51805569591479,-1.,0.89918504749193));
#38711=CARTESIAN_POINT('Ctrl Pts',(-1.50980486807181,-1.,0.894452006967538));
#38712=CARTESIAN_POINT('Ctrl Pts',(-1.5055822144029,-1.,0.892032620296855));
#38713=CARTESIAN_POINT('',(-1.60662857109684,-1.,0.693717979106305));
#38714=CARTESIAN_POINT('Origin',(0.,-1.,0.));
#38715=CARTESIAN_POINT('',(-2.0698113262342,-1.,0.7455743247944));
#38716=CARTESIAN_POINT('Ctrl Pts',(-1.60662857109684,-1.,0.693717979106305));
#38717=CARTESIAN_POINT('Ctrl Pts',(-1.61106790957619,-1.,0.69571209787897));
#38718=CARTESIAN_POINT('Ctrl Pts',(-1.61974673471117,-1.,0.699605146398837));
#38719=CARTESIAN_POINT('Ctrl Pts',(-1.6321654166204,-1.,0.705159151977294));
#38720=CARTESIAN_POINT('Ctrl Pts',(-1.64752408828442,-1.,0.711993139340447));
#38721=CARTESIAN_POINT('Ctrl Pts',(-1.66472880551777,-1.,0.71958543378795));
#38722=CARTESIAN_POINT('Ctrl Pts',(-1.67996158451922,-1.,0.726235967982445));
#38723=CARTESIAN_POINT('Ctrl Pts',(-1.69326921972915,-1.,0.731963238685357));
#38724=CARTESIAN_POINT('Ctrl Pts',(-1.70473309004249,-1.,0.736799665716932));
#38725=CARTESIAN_POINT('Ctrl Pts',(-1.71447789751001,-1.,0.74079516202821));
#38726=CARTESIAN_POINT('Ctrl Pts',(-1.72268229916769,-1.,0.744021445433093));
#38727=CARTESIAN_POINT('Ctrl Pts',(-1.72958533647714,-1.,0.746574710097752));
#38728=CARTESIAN_POINT('Ctrl Pts',(-1.7355035168033,-1.,0.74858246295687));
#38729=CARTESIAN_POINT('Ctrl Pts',(-1.74080458267114,-1.,0.750193435981249));
#38730=CARTESIAN_POINT('Ctrl Pts',(-1.74585086852502,-1.,0.751555614164482));
#38731=CARTESIAN_POINT('Ctrl Pts',(-1.75095139468794,-1.,0.752797683531314));
#38732=CARTESIAN_POINT('Ctrl Pts',(-1.75631083600019,-1.,0.754009254027829));
#38733=CARTESIAN_POINT('Ctrl Pts',(-1.76197817240128,-1.,0.755220979974461));
#38734=CARTESIAN_POINT('Ctrl Pts',(-1.76789396002998,-1.,0.75642189602781));
#38735=CARTESIAN_POINT('Ctrl Pts',(-1.77394167108292,-1.,0.757578264077029));
#38736=CARTESIAN_POINT('Ctrl Pts',(-1.77999411220945,-1.,0.758650626677518));
#38737=CARTESIAN_POINT('Ctrl Pts',(-1.78596964884604,-1.,0.759614401110189));
#38738=CARTESIAN_POINT('Ctrl Pts',(-1.7918581561088,-1.,0.760469555880749));
#38739=CARTESIAN_POINT('Ctrl Pts',(-1.79768986997783,-1.,0.761229695230558));
#38740=CARTESIAN_POINT('Ctrl Pts',(-1.80351583877342,-1.,0.761915336443547));
#38741=CARTESIAN_POINT('Ctrl Pts',(-1.80938551463965,-1.,0.762546129463938));
#38742=CARTESIAN_POINT('Ctrl Pts',(-1.8153211840553,-1.,0.763132003836634));
#38743=CARTESIAN_POINT('Ctrl Pts',(-1.82131873145266,-1.,0.763673465462726));
#38744=CARTESIAN_POINT('Ctrl Pts',(-1.82735991200065,-1.,0.764165902605995));
#38745=CARTESIAN_POINT('Ctrl Pts',(-1.83342077227142,-1.,0.764602549687853));
#38746=CARTESIAN_POINT('Ctrl Pts',(-1.83948181064835,-1.,0.764978057881737));
#38747=CARTESIAN_POINT('Ctrl Pts',(-1.84553698875924,-1.,0.765291664862029));
#38748=CARTESIAN_POINT('Ctrl Pts',(-1.85158945130063,-1.,0.765545710619062));
#38749=CARTESIAN_POINT('Ctrl Pts',(-1.85764741390394,-1.,0.765744212909318));
#38750=CARTESIAN_POINT('Ctrl Pts',(-1.86372027063312,-1.,0.765891519092547));
#38751=CARTESIAN_POINT('Ctrl Pts',(-1.86981398314341,-1.,0.765990708546091));
#38752=CARTESIAN_POINT('Ctrl Pts',(-1.87592888967883,-1.,0.766042837036744));
#38753=CARTESIAN_POINT('Ctrl Pts',(-1.88206215302561,-1.,0.766047794851864));
#38754=CARTESIAN_POINT('Ctrl Pts',(-1.88820926433409,-1.,0.766004837062091));
#38755=CARTESIAN_POINT('Ctrl Pts',(-1.89436577771388,-1.,0.765913193856978));
#38756=CARTESIAN_POINT('Ctrl Pts',(-1.90052930393596,-1.,0.765772772593386));
#38757=CARTESIAN_POINT('Ctrl Pts',(-1.90669961402356,-1.,0.765584196937919));
#38758=CARTESIAN_POINT('Ctrl Pts',(-1.91287765805169,-1.,0.765348465884722));
#38759=CARTESIAN_POINT('Ctrl Pts',(-1.91906491634196,-1.,0.765066729667088));
#38760=CARTESIAN_POINT('Ctrl Pts',(-1.92526263537048,-1.,0.764740025488211));
#38761=CARTESIAN_POINT('Ctrl Pts',(-1.93147105496382,-1.,0.76436901067394));
#38762=CARTESIAN_POINT('Ctrl Pts',(-1.93768964875886,-1.,0.763954049121458));
#38763=CARTESIAN_POINT('Ctrl Pts',(-1.9439174661764,-1.,0.763495333538629));
#38764=CARTESIAN_POINT('Ctrl Pts',(-1.95015342590024,-1.,0.762992990878769));
#38765=CARTESIAN_POINT('Ctrl Pts',(-1.95639665309869,-1.,0.762447203806179));
#38766=CARTESIAN_POINT('Ctrl Pts',(-1.96264672744186,-1.,0.761858300014423));
#38767=CARTESIAN_POINT('Ctrl Pts',(-1.96890351582499,-1.,0.76122669048382));
#38768=CARTESIAN_POINT('Ctrl Pts',(-1.97516705321494,-1.,0.760552825409757));
#38769=CARTESIAN_POINT('Ctrl Pts',(-1.98143741418172,-1.,0.75983714745219));
#38770=CARTESIAN_POINT('Ctrl Pts',(-1.98771456680874,-1.,0.759080037802488));
#38771=CARTESIAN_POINT('Ctrl Pts',(-1.99399831098817,-1.,0.758281796766761));
#38772=CARTESIAN_POINT('Ctrl Pts',(-2.00028834739178,-1.,0.757442676862724));
#38773=CARTESIAN_POINT('Ctrl Pts',(-2.0065843158773,-1.,0.75656290464667));
#38774=CARTESIAN_POINT('Ctrl Pts',(-2.01288584328084,-1.,0.755642704957865));
#38775=CARTESIAN_POINT('Ctrl Pts',(-2.01919259405809,-1.,0.754682330722816));
#38776=CARTESIAN_POINT('Ctrl Pts',(-2.02550428623313,-1.,0.753682061112768));
#38777=CARTESIAN_POINT('Ctrl Pts',(-2.03182068456221,-1.,0.752642180487211));
#38778=CARTESIAN_POINT('Ctrl Pts',(-2.03814160092099,-1.,0.751562963361115));
#38779=CARTESIAN_POINT('Ctrl Pts',(-2.04446689147979,-1.,0.750444657875576));
#38780=CARTESIAN_POINT('Ctrl Pts',(-2.05079645592154,-1.,0.749287468665046));
#38781=CARTESIAN_POINT('Ctrl Pts',(-2.05713023031006,-1.,0.748091554183802));
#38782=CARTESIAN_POINT('Ctrl Pts',(-2.06220058927826,-1.,0.747103932787919));
#38783=CARTESIAN_POINT('Ctrl Pts',(-2.06600523016815,-1.,0.7463458715442));
#38784=CARTESIAN_POINT('Ctrl Pts',(-2.06854248895728,-1.,0.745832791378367));
#38785=CARTESIAN_POINT('Ctrl Pts',(-2.0698113262342,-1.,0.7455743247944));
#38786=CARTESIAN_POINT('',(-2.11275013067528,-1.,0.61342227326009));
#38787=CARTESIAN_POINT('',(-2.0698113262342,-1.,0.7455743247944));
#38788=CARTESIAN_POINT('',(-1.7075470150345,-1.,0.383122945602004));
#38789=CARTESIAN_POINT('Ctrl Pts',(-2.11275013067528,-1.,0.61342227326009));
#38790=CARTESIAN_POINT('Ctrl Pts',(-2.11187554259986,-1.,0.6124673655618));
#38791=CARTESIAN_POINT('Ctrl Pts',(-2.11012443807238,-1.,0.610560911689899));
#38792=CARTESIAN_POINT('Ctrl Pts',(-2.1074919961518,-1.,0.607711315454876));
#38793=CARTESIAN_POINT('Ctrl Pts',(-2.10397049886949,-1.,0.60393203073603));
#38794=CARTESIAN_POINT('Ctrl Pts',(-2.0995493086477,-1.,0.599241616420533));
#38795=CARTESIAN_POINT('Ctrl Pts',(-2.0951087622027,-1.,0.594585006052162));
#38796=CARTESIAN_POINT('Ctrl Pts',(-2.09064881812129,-1.,0.589962365403406));
#38797=CARTESIAN_POINT('Ctrl Pts',(-2.08616943727951,-1.,0.585373918991617));
#38798=CARTESIAN_POINT('Ctrl Pts',(-2.08167059018418,-1.,0.580819952108063));
#38799=CARTESIAN_POINT('Ctrl Pts',(-2.07715226767559,-1.,0.576300797416844));
#38800=CARTESIAN_POINT('Ctrl Pts',(-2.07261449292824,-1.,0.571816823242603));
#38801=CARTESIAN_POINT('Ctrl Pts',(-2.06805732997334,-1.,0.567368421181087));
#38802=CARTESIAN_POINT('Ctrl Pts',(-2.06348090160589,-1.,0.562955993082261));
#38803=CARTESIAN_POINT('Ctrl Pts',(-2.05888537756462,-1.,0.558579940185151));
#38804=CARTESIAN_POINT('Ctrl Pts',(-2.05427091604413,-1.,0.554240657463906));
#38805=CARTESIAN_POINT('Ctrl Pts',(-2.04963761077958,-1.,0.549938525150295));
#38806=CARTESIAN_POINT('Ctrl Pts',(-2.04498544714588,-1.,0.54567390381743));
#38807=CARTESIAN_POINT('Ctrl Pts',(-2.04031422690527,-1.,0.541447120615659));
#38808=CARTESIAN_POINT('Ctrl Pts',(-2.03562362954037,-1.,0.537258489833262));
#38809=CARTESIAN_POINT('Ctrl Pts',(-2.03091336214426,-1.,0.533108355132976));
#38810=CARTESIAN_POINT('Ctrl Pts',(-2.0261832908329,-1.,0.528997127241914));
#38811=CARTESIAN_POINT('Ctrl Pts',(-2.02143356304698,-1.,0.524925318333476));
#38812=CARTESIAN_POINT('Ctrl Pts',(-2.01666477917286,-1.,0.52089359039937));
#38813=CARTESIAN_POINT('Ctrl Pts',(-2.01187773939242,-1.,0.516902681728687));
#38814=CARTESIAN_POINT('Ctrl Pts',(-2.00707309946949,-1.,0.512953306961792));
#38815=CARTESIAN_POINT('Ctrl Pts',(-2.00225107134734,-1.,0.509046069886157));
#38816=CARTESIAN_POINT('Ctrl Pts',(-1.99741107463572,-1.,0.505181361323026));
#38817=CARTESIAN_POINT('Ctrl Pts',(-1.99255149126155,-1.,0.501359287727146));
#38818=CARTESIAN_POINT('Ctrl Pts',(-1.98767044752932,-1.,0.497579909545574));
#38819=CARTESIAN_POINT('Ctrl Pts',(-1.98276658761821,-1.,0.493843476541494));
#38820=CARTESIAN_POINT('Ctrl Pts',(-1.97783973019229,-1.,0.490150627860952));
#38821=CARTESIAN_POINT('Ctrl Pts',(-1.97289186263272,-1.,0.486502692907659));
#38822=CARTESIAN_POINT('Ctrl Pts',(-1.96792703422362,-1.,0.48290166212069));
#38823=CARTESIAN_POINT('Ctrl Pts',(-1.96294933055943,-1.,0.479349583074855));
#38824=CARTESIAN_POINT('Ctrl Pts',(-1.95796111148177,-1.,0.475848034683176));
#38825=CARTESIAN_POINT('Ctrl Pts',(-1.95296148278133,-1.,0.472397672264072));
#38826=CARTESIAN_POINT('Ctrl Pts',(-1.94794381136514,-1.,0.468997482913135));
#38827=CARTESIAN_POINT('Ctrl Pts',(-1.9428979419619,-1.,0.46564546202603));
#38828=CARTESIAN_POINT('Ctrl Pts',(-1.93781486640821,-1.,0.462340031009056));
#38829=CARTESIAN_POINT('Ctrl Pts',(-1.93269066517934,-1.,0.459081234547926));
#38830=CARTESIAN_POINT('Ctrl Pts',(-1.92753067150476,-1.,0.455872005174371));
#38831=CARTESIAN_POINT('Ctrl Pts',(-1.92235380648502,-1.,0.452719478359432));
#38832=CARTESIAN_POINT('Ctrl Pts',(-1.91718342555755,-1.,0.449632260106662));
#38833=CARTESIAN_POINT('Ctrl Pts',(-1.9120369998112,-1.,0.446617343485711));
#38834=CARTESIAN_POINT('Ctrl Pts',(-1.90691756144898,-1.,0.44367755684915));
#38835=CARTESIAN_POINT('Ctrl Pts',(-1.90180124389086,-1.,0.440807833704038));
#38836=CARTESIAN_POINT('Ctrl Pts',(-1.89663648956466,-1.,0.437995003948244));
#38837=CARTESIAN_POINT('Ctrl Pts',(-1.89136993975504,-1.,0.435225660963383));
#38838=CARTESIAN_POINT('Ctrl Pts',(-1.88596913666793,-1.,0.432493038548748));
#38839=CARTESIAN_POINT('Ctrl Pts',(-1.88044229001832,-1.,0.429803062482344));
#38840=CARTESIAN_POINT('Ctrl Pts',(-1.87486989291484,-1.,0.427183828519102));
#38841=CARTESIAN_POINT('Ctrl Pts',(-1.86937803944323,-1.,0.424678177291359));
#38842=CARTESIAN_POINT('Ctrl Pts',(-1.86408083334028,-1.,0.422327307418275));
#38843=CARTESIAN_POINT('Ctrl Pts',(-1.85903281096686,-1.,0.420157287975619));
#38844=CARTESIAN_POINT('Ctrl Pts',(-1.85417632856234,-1.,0.418164129143534));
#38845=CARTESIAN_POINT('Ctrl Pts',(-1.84929312929882,-1.,0.416300022038864));
#38846=CARTESIAN_POINT('Ctrl Pts',(-1.8440575707371,-1.,0.41448743825434));
#38847=CARTESIAN_POINT('Ctrl Pts',(-1.83808953475839,-1.,0.412633125322161));
#38848=CARTESIAN_POINT('Ctrl Pts',(-1.83100408895216,-1.,0.410641256301675));
#38849=CARTESIAN_POINT('Ctrl Pts',(-1.8224702267854,-1.,0.408428948108533));
#38850=CARTESIAN_POINT('Ctrl Pts',(-1.81223801813988,-1.,0.405933518411838));
#38851=CARTESIAN_POINT('Ctrl Pts',(-1.80012077176221,-1.,0.403107976170441));
#38852=CARTESIAN_POINT('Ctrl Pts',(-1.78598826347533,-1.,0.39991940378308));
#38853=CARTESIAN_POINT('Ctrl Pts',(-1.7697556004756,-1.,0.39634619612042));
#38854=CARTESIAN_POINT('Ctrl Pts',(-1.75137405313962,-1.,0.392375812294307));
#38855=CARTESIAN_POINT('Ctrl Pts',(-1.7349317097561,-1.,0.388877023509191));
#38856=CARTESIAN_POINT('Ctrl Pts',(-1.72162022246158,-1.,0.38607079032701));
#38857=CARTESIAN_POINT('Ctrl Pts',(-1.71231062891958,-1.,0.384119047315542));
#38858=CARTESIAN_POINT('Ctrl Pts',(-1.7075470150345,-1.,0.383122945602004));
#38859=CARTESIAN_POINT('',(-1.74236521665491,-1.,0.163289472382896));
#38860=CARTESIAN_POINT('Origin',(0.,-1.,0.));
#38861=CARTESIAN_POINT('',(-2.19890268624765,-1.,0.069476445021958));
#38862=CARTESIAN_POINT('Ctrl Pts',(-1.74236521665491,-1.,0.163289472382896));
#38863=CARTESIAN_POINT('Ctrl Pts',(-1.7472034950333,-1.,0.163814161002002));
#38864=CARTESIAN_POINT('Ctrl Pts',(-1.75666056638427,-1.,0.164834765707158));
#38865=CARTESIAN_POINT('Ctrl Pts',(-1.77018771684844,-1.,0.1662793551464));
#38866=CARTESIAN_POINT('Ctrl Pts',(-1.7869064998507,-1.,0.168032772805197));
#38867=CARTESIAN_POINT('Ctrl Pts',(-1.80561530629706,-1.,0.169936923904608));
#38868=CARTESIAN_POINT('Ctrl Pts',(-1.82215766811545,-1.,0.171554770204119));
#38869=CARTESIAN_POINT('Ctrl Pts',(-1.83658380527692,-1.,0.1728894428919));
#38870=CARTESIAN_POINT('Ctrl Pts',(-1.8489811319852,-1.,0.173946627587731));
#38871=CARTESIAN_POINT('Ctrl Pts',(-1.85948367088837,-1.,0.17473525927603));
#38872=CARTESIAN_POINT('Ctrl Pts',(-1.86828349694799,-1.,0.175268337590758));
#38873=CARTESIAN_POINT('Ctrl Pts',(-1.87563767773588,-1.,0.175563480746485));
#38874=CARTESIAN_POINT('Ctrl Pts',(-1.88188663145367,-1.,0.175644148889698));
#38875=CARTESIAN_POINT('Ctrl Pts',(-1.88742606273259,-1.,0.175538155840648));
#38876=CARTESIAN_POINT('Ctrl Pts',(-1.892646301985,-1.,0.175274276190844));
#38877=CARTESIAN_POINT('Ctrl Pts',(-1.89788101117132,-1.,0.174879405091263));
#38878=CARTESIAN_POINT('Ctrl Pts',(-1.90335253862834,-1.,0.174375518661085));
#38879=CARTESIAN_POINT('Ctrl Pts',(-1.90911693975267,-1.,0.173776635257817));
#38880=CARTESIAN_POINT('Ctrl Pts',(-1.91511429159527,-1.,0.173090695383496));
#38881=CARTESIAN_POINT('Ctrl Pts',(-1.9212233439798,-1.,0.172321621259514));
#38882=CARTESIAN_POINT('Ctrl Pts',(-1.92731093582036,-1.,0.171471191532988));
#38883=CARTESIAN_POINT('Ctrl Pts',(-1.93329183155539,-1.,0.170541253116201));
#38884=CARTESIAN_POINT('Ctrl Pts',(-1.93915639211581,-1.,0.169534904817491));
#38885=CARTESIAN_POINT('Ctrl Pts',(-1.94493757756931,-1.,0.168455741607556));
#38886=CARTESIAN_POINT('Ctrl Pts',(-1.95069027794294,-1.,0.167307501784475));
#38887=CARTESIAN_POINT('Ctrl Pts',(-1.9564675971873,-1.,0.166093592002812));
#38888=CARTESIAN_POINT('Ctrl Pts',(-1.96229379940136,-1.,0.164816568920269));
#38889=CARTESIAN_POINT('Ctrl Pts',(-1.96816512677967,-1.,0.163478185457734));
#38890=CARTESIAN_POINT('Ctrl Pts',(-1.97406280235188,-1.,0.162079693556288));
#38891=CARTESIAN_POINT('Ctrl Pts',(-1.97996195437559,-1.,0.160622060784611));
#38892=CARTESIAN_POINT('Ctrl Pts',(-1.98584238283292,-1.,0.159106226437299));
#38893=CARTESIAN_POINT('Ctrl Pts',(-1.99169810931908,-1.,0.157533331459227));
#38894=CARTESIAN_POINT('Ctrl Pts',(-1.99753284771497,-1.,0.155904629548783));
#38895=CARTESIAN_POINT('Ctrl Pts',(-2.00335565310543,-1.,0.154221403049722));
#38896=CARTESIAN_POINT('Ctrl Pts',(-2.00917680318424,-1.,0.15248488362145));
#38897=CARTESIAN_POINT('Ctrl Pts',(-2.01500291940238,-1.,0.150696157673078));
#38898=CARTESIAN_POINT('Ctrl Pts',(-2.02083464969894,-1.,0.148856124775337));
#38899=CARTESIAN_POINT('Ctrl Pts',(-2.02666926182017,-1.,0.146965557332583));
#38900=CARTESIAN_POINT('Ctrl Pts',(-2.03250223739942,-1.,0.145025140186057));
#38901=CARTESIAN_POINT('Ctrl Pts',(-2.03832911025912,-1.,0.143035515058209));
#38902=CARTESIAN_POINT('Ctrl Pts',(-2.04414757947916,-1.,0.140997332152546));
#38903=CARTESIAN_POINT('Ctrl Pts',(-2.04995762001328,-1.,0.138911255368966));
#38904=CARTESIAN_POINT('Ctrl Pts',(-2.05576044414264,-1.,0.136777941218043));
#38905=CARTESIAN_POINT('Ctrl Pts',(-2.06155781517842,-1.,0.134598026192106));
#38906=CARTESIAN_POINT('Ctrl Pts',(-2.06735123910326,-1.,0.13237211154771));
#38907=CARTESIAN_POINT('Ctrl Pts',(-2.07314114713063,-1.,0.130100748328403));
#38908=CARTESIAN_POINT('Ctrl Pts',(-2.07892715110987,-1.,0.12778444527612));
#38909=CARTESIAN_POINT('Ctrl Pts',(-2.08470840653643,-1.,0.125423679412061));
#38910=CARTESIAN_POINT('Ctrl Pts',(-2.09048392424825,-1.,0.123018905621083));
#38911=CARTESIAN_POINT('Ctrl Pts',(-2.0962529286773,-1.,0.120570567965122));
#38912=CARTESIAN_POINT('Ctrl Pts',(-2.102015121329,-1.,0.118079107988355));
#38913=CARTESIAN_POINT('Ctrl Pts',(-2.10777050261309,-1.,0.115544957687926));
#38914=CARTESIAN_POINT('Ctrl Pts',(-2.11351924490306,-1.,0.112968534419737));
#38915=CARTESIAN_POINT('Ctrl Pts',(-2.11926155590865,-1.,0.110350236135025));
#38916=CARTESIAN_POINT('Ctrl Pts',(-2.12499752307,-1.,0.10769043523109));
#38917=CARTESIAN_POINT('Ctrl Pts',(-2.13072704887293,-1.,0.104989479152739));
#38918=CARTESIAN_POINT('Ctrl Pts',(-2.13644992667165,-1.,0.1022477005561));
#38919=CARTESIAN_POINT('Ctrl Pts',(-2.14216588396025,-1.,0.0994654261990914));
#38920=CARTESIAN_POINT('Ctrl Pts',(-2.14787463531795,-1.,0.0966429852305457));
#38921=CARTESIAN_POINT('Ctrl Pts',(-2.1535759397817,-1.,0.0937807218867642));
#38922=CARTESIAN_POINT('Ctrl Pts',(-2.15926961544516,-1.,0.0908789888107264));
#38923=CARTESIAN_POINT('Ctrl Pts',(-2.16495552645014,-1.,0.0879381291386921));
#38924=CARTESIAN_POINT('Ctrl Pts',(-2.17063357870952,-1.,0.0849584620835371));
#38925=CARTESIAN_POINT('Ctrl Pts',(-2.176303712113,-1.,0.0819402680872764));
#38926=CARTESIAN_POINT('Ctrl Pts',(-2.18196589448887,-1.,0.0788837727685241));
#38927=CARTESIAN_POINT('Ctrl Pts',(-2.1876201139953,-1.,0.0757891465836146));
#38928=CARTESIAN_POINT('Ctrl Pts',(-2.19213712013662,-1.,0.0732830357306724));
#38929=CARTESIAN_POINT('Ctrl Pts',(-2.19552129484002,-1.,0.0713863779526153));
#38930=CARTESIAN_POINT('Ctrl Pts',(-2.19777582085423,-1.,0.0701143536325489));
#38931=CARTESIAN_POINT('Ctrl Pts',(-2.19890268624765,-1.,0.069476445021958));
#38932=CARTESIAN_POINT('',(-2.19890268624765,-1.,-0.0694764450219585));
#38933=CARTESIAN_POINT('',(-2.19890268624765,-1.,0.069476445021958));
#38934=CARTESIAN_POINT('',(-1.74236521665491,-1.,-0.163289472382896));
#38935=CARTESIAN_POINT('Ctrl Pts',(-2.19890268624765,-1.,-0.0694764450219585));
#38936=CARTESIAN_POINT('Ctrl Pts',(-2.19777582085261,-1.,-0.0701143536324927));
#38937=CARTESIAN_POINT('Ctrl Pts',(-2.19552129483562,-1.,-0.0713863779524629));
#38938=CARTESIAN_POINT('Ctrl Pts',(-2.19213712012956,-1.,-0.0732830357304277));
#38939=CARTESIAN_POINT('Ctrl Pts',(-2.1876201139874,-1.,-0.0757891465833413));
#38940=CARTESIAN_POINT('Ctrl Pts',(-2.18196589448304,-1.,-0.0788837727683229));
#38941=CARTESIAN_POINT('Ctrl Pts',(-2.1763037121106,-1.,-0.0819402680871941));
#38942=CARTESIAN_POINT('Ctrl Pts',(-2.17063357871031,-1.,-0.0849584620835644));
#38943=CARTESIAN_POINT('Ctrl Pts',(-2.16495552645275,-1.,-0.0879381291387824));
#38944=CARTESIAN_POINT('Ctrl Pts',(-2.15926961544808,-1.,-0.0908789888108267));
#38945=CARTESIAN_POINT('Ctrl Pts',(-2.15357593978377,-1.,-0.0937807218868346));
#38946=CARTESIAN_POINT('Ctrl Pts',(-2.14787463531864,-1.,-0.096642985230569));
#38947=CARTESIAN_POINT('Ctrl Pts',(-2.14216588395974,-1.,-0.0994654261990744));
#38948=CARTESIAN_POINT('Ctrl Pts',(-2.13644992667052,-1.,-0.102247700556064));
#38949=CARTESIAN_POINT('Ctrl Pts',(-2.1307270488718,-1.,-0.104989479152703));
#38950=CARTESIAN_POINT('Ctrl Pts',(-2.12499752306927,-1.,-0.107690435231068));
#38951=CARTESIAN_POINT('Ctrl Pts',(-2.11926155590849,-1.,-0.11035023613502));
#38952=CARTESIAN_POINT('Ctrl Pts',(-2.11351924490335,-1.,-0.112968534419746));
#38953=CARTESIAN_POINT('Ctrl Pts',(-2.10777050261359,-1.,-0.11554495768794));
#38954=CARTESIAN_POINT('Ctrl Pts',(-2.10201512132945,-1.,-0.118079107988368));
#38955=CARTESIAN_POINT('Ctrl Pts',(-2.09625292867756,-1.,-0.120570567965129));
#38956=CARTESIAN_POINT('Ctrl Pts',(-2.09048392424826,-1.,-0.123018905621083));
#38957=CARTESIAN_POINT('Ctrl Pts',(-2.08470840653628,-1.,-0.125423679412058));
#38958=CARTESIAN_POINT('Ctrl Pts',(-2.07892715110967,-1.,-0.127784445276116));
#38959=CARTESIAN_POINT('Ctrl Pts',(-2.07314114713047,-1.,-0.130100748328401));
#38960=CARTESIAN_POINT('Ctrl Pts',(-2.06735123910319,-1.,-0.13237211154771));
#38961=CARTESIAN_POINT('Ctrl Pts',(-2.06155781517844,-1.,-0.134598026192107));
#38962=CARTESIAN_POINT('Ctrl Pts',(-2.0557604441427,-1.,-0.136777941218044));
#38963=CARTESIAN_POINT('Ctrl Pts',(-2.04995762001333,-1.,-0.138911255368966));
#38964=CARTESIAN_POINT('Ctrl Pts',(-2.04414757947919,-1.,-0.140997332152545));
#38965=CARTESIAN_POINT('Ctrl Pts',(-2.03832911025913,-1.,-0.143035515058208));
#38966=CARTESIAN_POINT('Ctrl Pts',(-2.03250223739941,-1.,-0.145025140186058));
#38967=CARTESIAN_POINT('Ctrl Pts',(-2.02666926182017,-1.,-0.146965557332586));
#38968=CARTESIAN_POINT('Ctrl Pts',(-2.02083464969897,-1.,-0.148856124775343));
#38969=CARTESIAN_POINT('Ctrl Pts',(-2.01500291940243,-1.,-0.150696157673084));
#38970=CARTESIAN_POINT('Ctrl Pts',(-2.00917680318426,-1.,-0.152484883621452));
#38971=CARTESIAN_POINT('Ctrl Pts',(-2.00335565310539,-1.,-0.154221403049719));
#38972=CARTESIAN_POINT('Ctrl Pts',(-1.99753284771487,-1.,-0.155904629548775));
#38973=CARTESIAN_POINT('Ctrl Pts',(-1.99169810931893,-1.,-0.157533331459215));
#38974=CARTESIAN_POINT('Ctrl Pts',(-1.98584238283279,-1.,-0.159106226437289));
#38975=CARTESIAN_POINT('Ctrl Pts',(-1.97996195437557,-1.,-0.16062206078461));
#38976=CARTESIAN_POINT('Ctrl Pts',(-1.97406280235204,-1.,-0.162079693556302));
#38977=CARTESIAN_POINT('Ctrl Pts',(-1.96816512678,-1.,-0.16347818545776));
#38978=CARTESIAN_POINT('Ctrl Pts',(-1.96229379940174,-1.,-0.1648165689203));
#38979=CARTESIAN_POINT('Ctrl Pts',(-1.95646759718755,-1.,-0.166093592002833));
#38980=CARTESIAN_POINT('Ctrl Pts',(-1.95069027794286,-1.,-0.167307501784469));
#38981=CARTESIAN_POINT('Ctrl Pts',(-1.94493757756879,-1.,-0.168455741607516));
#38982=CARTESIAN_POINT('Ctrl Pts',(-1.93915639211497,-1.,-0.169534904817425));
#38983=CARTESIAN_POINT('Ctrl Pts',(-1.93329183155455,-1.,-0.170541253116136));
#38984=CARTESIAN_POINT('Ctrl Pts',(-1.92731093582,-1.,-0.17147119153296));
#38985=CARTESIAN_POINT('Ctrl Pts',(-1.92122334398034,-1.,-0.172321621259557));
#38986=CARTESIAN_POINT('Ctrl Pts',(-1.91511429159681,-1.,-0.173090695383619));
#38987=CARTESIAN_POINT('Ctrl Pts',(-1.90911693975475,-1.,-0.173776635257984));
#38988=CARTESIAN_POINT('Ctrl Pts',(-1.90335253863003,-1.,-0.174375518661222));
#38989=CARTESIAN_POINT('Ctrl Pts',(-1.89788101117148,-1.,-0.174879405091277));
#38990=CARTESIAN_POINT('Ctrl Pts',(-1.89264630198279,-1.,-0.175274276190664));
#38991=CARTESIAN_POINT('Ctrl Pts',(-1.88742606272818,-1.,-0.175538155840286));
#38992=CARTESIAN_POINT('Ctrl Pts',(-1.88188663144846,-1.,-0.175644148889271));
#38993=CARTESIAN_POINT('Ctrl Pts',(-1.87563767773249,-1.,-0.175563480746205));
#38994=CARTESIAN_POINT('Ctrl Pts',(-1.86828349694972,-1.,-0.175268337590901));
#38995=CARTESIAN_POINT('Ctrl Pts',(-1.85948367089838,-1.,-0.174735259276856));
#38996=CARTESIAN_POINT('Ctrl Pts',(-1.84898113200543,-1.,-0.173946627589401));
#38997=CARTESIAN_POINT('Ctrl Pts',(-1.83658380530747,-1.,-0.17288944289442));
#38998=CARTESIAN_POINT('Ctrl Pts',(-1.82215766815414,-1.,-0.171554770207306));
#38999=CARTESIAN_POINT('Ctrl Pts',(-1.80561530633924,-1.,-0.169936923908078));
#39000=CARTESIAN_POINT('Ctrl Pts',(-1.78690649988931,-1.,-0.16803277280837));
#39001=CARTESIAN_POINT('Ctrl Pts',(-1.77018771687692,-1.,-0.166279355148738));
#39002=CARTESIAN_POINT('Ctrl Pts',(-1.75666056640041,-1.,-0.164834765708484));
#39003=CARTESIAN_POINT('Ctrl Pts',(-1.74720349503904,-1.,-0.163814161002474));
#39004=CARTESIAN_POINT('Ctrl Pts',(-1.74236521665491,-1.,-0.163289472382896));
#39005=CARTESIAN_POINT('',(-1.7075470150345,-1.,-0.383122945602004));
#39006=CARTESIAN_POINT('Origin',(0.,-1.,0.));
#39007=CARTESIAN_POINT('',(-2.11275013067528,-1.,-0.61342227326009));
#39008=CARTESIAN_POINT('Ctrl Pts',(-1.7075470150345,-1.,-0.383122945602004));
#39009=CARTESIAN_POINT('Ctrl Pts',(-1.71231062891398,-1.,-0.384119047314215));
#39010=CARTESIAN_POINT('Ctrl Pts',(-1.72162022244582,-1.,-0.386070790323281));
#39011=CARTESIAN_POINT('Ctrl Pts',(-1.73493170972829,-1.,-0.388877023502615));
#39012=CARTESIAN_POINT('Ctrl Pts',(-1.75137405310193,-1.,-0.392375812285395));
#39013=CARTESIAN_POINT('Ctrl Pts',(-1.76975560043442,-1.,-0.396346196110688));
#39014=CARTESIAN_POINT('Ctrl Pts',(-1.78598826343754,-1.,-0.399919403774155));
#39015=CARTESIAN_POINT('Ctrl Pts',(-1.80012077173238,-1.,-0.403107976163396));
#39016=CARTESIAN_POINT('Ctrl Pts',(-1.81223801812013,-1.,-0.405933518407175));
#39017=CARTESIAN_POINT('Ctrl Pts',(-1.82247022677562,-1.,-0.408428948106227));
#39018=CARTESIAN_POINT('Ctrl Pts',(-1.83100408895047,-1.,-0.410641256301276));
#39019=CARTESIAN_POINT('Ctrl Pts',(-1.8380895347617,-1.,-0.412633125322945));
#39020=CARTESIAN_POINT('Ctrl Pts',(-1.84405757074218,-1.,-0.414487438255542));
#39021=CARTESIAN_POINT('Ctrl Pts',(-1.84929312930314,-1.,-0.416300022039885));
#39022=CARTESIAN_POINT('Ctrl Pts',(-1.8541763285645,-1.,-0.418164129144045));
#39023=CARTESIAN_POINT('Ctrl Pts',(-1.8590328109667,-1.,-0.420157287975583));
#39024=CARTESIAN_POINT('Ctrl Pts',(-1.86408083333863,-1.,-0.422327307417884));
#39025=CARTESIAN_POINT('Ctrl Pts',(-1.8693780394412,-1.,-0.424678177290876));
#39026=CARTESIAN_POINT('Ctrl Pts',(-1.87486989291333,-1.,-0.427183828518743));
#39027=CARTESIAN_POINT('Ctrl Pts',(-1.88044229001778,-1.,-0.429803062482217));
#39028=CARTESIAN_POINT('Ctrl Pts',(-1.88596913666828,-1.,-0.432493038548833));
#39029=CARTESIAN_POINT('Ctrl Pts',(-1.89136993975585,-1.,-0.43522566096358));
#39030=CARTESIAN_POINT('Ctrl Pts',(-1.89663648956549,-1.,-0.437995003948443));
#39031=CARTESIAN_POINT('Ctrl Pts',(-1.90180124389137,-1.,-0.44080783370416));
#39032=CARTESIAN_POINT('Ctrl Pts',(-1.90691756144906,-1.,-0.44367755684917));
#39033=CARTESIAN_POINT('Ctrl Pts',(-1.91203699981095,-1.,-0.446617343485651));
#39034=CARTESIAN_POINT('Ctrl Pts',(-1.91718342555717,-1.,-0.449632260106572));
#39035=CARTESIAN_POINT('Ctrl Pts',(-1.9223538064847,-1.,-0.452719478359356));
#39036=CARTESIAN_POINT('Ctrl Pts',(-1.92753067150461,-1.,-0.455872005174335));
#39037=CARTESIAN_POINT('Ctrl Pts',(-1.93269066517936,-1.,-0.459081234547931));
#39038=CARTESIAN_POINT('Ctrl Pts',(-1.93781486640834,-1.,-0.462340031009087));
#39039=CARTESIAN_POINT('Ctrl Pts',(-1.94289794196205,-1.,-0.465645462026064));
#39040=CARTESIAN_POINT('Ctrl Pts',(-1.94794381136524,-1.,-0.468997482913158));
#39041=CARTESIAN_POINT('Ctrl Pts',(-1.95296148278136,-1.,-0.472397672264079));
#39042=CARTESIAN_POINT('Ctrl Pts',(-1.95796111148175,-1.,-0.475848034683171));
#39043=CARTESIAN_POINT('Ctrl Pts',(-1.96294933055938,-1.,-0.479349583074846));
#39044=CARTESIAN_POINT('Ctrl Pts',(-1.96792703422358,-1.,-0.482901662120686));
#39045=CARTESIAN_POINT('Ctrl Pts',(-1.97289186263272,-1.,-0.486502692907661));
#39046=CARTESIAN_POINT('Ctrl Pts',(-1.97783973019229,-1.,-0.490150627860955));
#39047=CARTESIAN_POINT('Ctrl Pts',(-1.9827665876182,-1.,-0.493843476541492));
#39048=CARTESIAN_POINT('Ctrl Pts',(-1.98767044752929,-1.,-0.497579909545564));
#39049=CARTESIAN_POINT('Ctrl Pts',(-1.9925514912615,-1.,-0.501359287727129));
#39050=CARTESIAN_POINT('Ctrl Pts',(-1.99741107463567,-1.,-0.505181361323011));
#39051=CARTESIAN_POINT('Ctrl Pts',(-2.00225107134733,-1.,-0.509046069886152));
#39052=CARTESIAN_POINT('Ctrl Pts',(-2.00707309946955,-1.,-0.512953306961813));
#39053=CARTESIAN_POINT('Ctrl Pts',(-2.01187773939257,-1.,-0.516902681728733));
#39054=CARTESIAN_POINT('Ctrl Pts',(-2.01666477917305,-1.,-0.520893590399428));
#39055=CARTESIAN_POINT('Ctrl Pts',(-2.02143356304712,-1.,-0.524925318333518));
#39056=CARTESIAN_POINT('Ctrl Pts',(-2.02618329083289,-1.,-0.52899712724191));
#39057=CARTESIAN_POINT('Ctrl Pts',(-2.03091336214401,-1.,-0.533108355132905));
#39058=CARTESIAN_POINT('Ctrl Pts',(-2.03562362953993,-1.,-0.537258489833134));
#39059=CARTESIAN_POINT('Ctrl Pts',(-2.0403142269048,-1.,-0.54144712061552));
#39060=CARTESIAN_POINT('Ctrl Pts',(-2.0449854471456,-1.,-0.545673903817348));
#39061=CARTESIAN_POINT('Ctrl Pts',(-2.04963761077974,-1.,-0.549938525150342));
#39062=CARTESIAN_POINT('Ctrl Pts',(-2.05427091604482,-1.,-0.554240657464109));
#39063=CARTESIAN_POINT('Ctrl Pts',(-2.05888537756571,-1.,-0.558579940185467));
#39064=CARTESIAN_POINT('Ctrl Pts',(-2.06348090160697,-1.,-0.562955993082574));
#39065=CARTESIAN_POINT('Ctrl Pts',(-2.06805732997383,-1.,-0.567368421181229));
#39066=CARTESIAN_POINT('Ctrl Pts',(-2.07261449292757,-1.,-0.571816823242411));
#39067=CARTESIAN_POINT('Ctrl Pts',(-2.07715226767361,-1.,-0.576300797416274));
#39068=CARTESIAN_POINT('Ctrl Pts',(-2.08167059018138,-1.,-0.580819952107257));
#39069=CARTESIAN_POINT('Ctrl Pts',(-2.086169437277,-1.,-0.585373918990895));
#39070=CARTESIAN_POINT('Ctrl Pts',(-2.09064881812053,-1.,-0.589962365403189));
#39071=CARTESIAN_POINT('Ctrl Pts',(-2.09510876220501,-1.,-0.594585006052823));
#39072=CARTESIAN_POINT('Ctrl Pts',(-2.09954930865331,-1.,-0.599241616422144));
#39073=CARTESIAN_POINT('Ctrl Pts',(-2.10397049887709,-1.,-0.603932030738212));
#39074=CARTESIAN_POINT('Ctrl Pts',(-2.10749199615859,-1.,-0.607711315456826));
#39075=CARTESIAN_POINT('Ctrl Pts',(-2.11012443807661,-1.,-0.610560911691113));
#39076=CARTESIAN_POINT('Ctrl Pts',(-2.11187554260142,-1.,-0.61246736556225));
#39077=CARTESIAN_POINT('Ctrl Pts',(-2.11275013067528,-1.,-0.61342227326009));
#39078=CARTESIAN_POINT('',(-2.0698113262342,-1.,-0.745574324794401));
#39079=CARTESIAN_POINT('',(-2.11275013067528,-1.,-0.61342227326009));
#39080=CARTESIAN_POINT('',(-1.60662857109684,-1.,-0.693717979106306));
#39081=CARTESIAN_POINT('Ctrl Pts',(-2.0698113262342,-1.,-0.745574324794401));
#39082=CARTESIAN_POINT('Ctrl Pts',(-2.06854248895575,-1.,-0.74583279137781));
#39083=CARTESIAN_POINT('Ctrl Pts',(-2.06600523016401,-1.,-0.746345871542695));
#39084=CARTESIAN_POINT('Ctrl Pts',(-2.06220058927162,-1.,-0.747103932785504));
#39085=CARTESIAN_POINT('Ctrl Pts',(-2.05713023030263,-1.,-0.748091554181101));
#39086=CARTESIAN_POINT('Ctrl Pts',(-2.05079645591606,-1.,-0.749287468663053));
#39087=CARTESIAN_POINT('Ctrl Pts',(-2.04446689147754,-1.,-0.750444657874758));
#39088=CARTESIAN_POINT('Ctrl Pts',(-2.03814160092173,-1.,-0.751562963361383));
#39089=CARTESIAN_POINT('Ctrl Pts',(-2.03182068456467,-1.,-0.752642180488104));
#39090=CARTESIAN_POINT('Ctrl Pts',(-2.02550428623587,-1.,-0.753682061113765));
#39091=CARTESIAN_POINT('Ctrl Pts',(-2.01919259406003,-1.,-0.75468233072352));
#39092=CARTESIAN_POINT('Ctrl Pts',(-2.01288584328149,-1.,-0.7556427049581));
#39093=CARTESIAN_POINT('Ctrl Pts',(-2.00658431587682,-1.,-0.756562904646496));
#39094=CARTESIAN_POINT('Ctrl Pts',(-2.00028834739072,-1.,-0.757442676862341));
#39095=CARTESIAN_POINT('Ctrl Pts',(-1.9939983109871,-1.,-0.758281796766377));
#39096=CARTESIAN_POINT('Ctrl Pts',(-1.98771456680806,-1.,-0.759080037802242));
#39097=CARTESIAN_POINT('Ctrl Pts',(-1.98143741418156,-1.,-0.759837147452135));
#39098=CARTESIAN_POINT('Ctrl Pts',(-1.97516705321521,-1.,-0.760552825409855));
#39099=CARTESIAN_POINT('Ctrl Pts',(-1.96890351582545,-1.,-0.761226690483986));
#39100=CARTESIAN_POINT('Ctrl Pts',(-1.96264672744229,-1.,-0.761858300014575));
#39101=CARTESIAN_POINT('Ctrl Pts',(-1.95639665309893,-1.,-0.762447203806263));
#39102=CARTESIAN_POINT('Ctrl Pts',(-1.95015342590025,-1.,-0.762992990878774));
#39103=CARTESIAN_POINT('Ctrl Pts',(-1.94391746617626,-1.,-0.76349533353858));
#39104=CARTESIAN_POINT('Ctrl Pts',(-1.93768964875867,-1.,-0.763954049121393));
#39105=CARTESIAN_POINT('Ctrl Pts',(-1.93147105496367,-1.,-0.764369010673889));
#39106=CARTESIAN_POINT('Ctrl Pts',(-1.92526263537041,-1.,-0.764740025488189));
#39107=CARTESIAN_POINT('Ctrl Pts',(-1.91906491634197,-1.,-0.765066729667095));
#39108=CARTESIAN_POINT('Ctrl Pts',(-1.91287765805174,-1.,-0.765348465884739));
#39109=CARTESIAN_POINT('Ctrl Pts',(-1.90669961402362,-1.,-0.765584196937936));
#39110=CARTESIAN_POINT('Ctrl Pts',(-1.90052930393599,-1.,-0.765772772593395));
#39111=CARTESIAN_POINT('Ctrl Pts',(-1.89436577771389,-1.,-0.765913193856979));
#39112=CARTESIAN_POINT('Ctrl Pts',(-1.88820926433409,-1.,-0.76600483706209));
#39113=CARTESIAN_POINT('Ctrl Pts',(-1.88206215302561,-1.,-0.766047794851868));
#39114=CARTESIAN_POINT('Ctrl Pts',(-1.87592888967886,-1.,-0.766042837036759));
#39115=CARTESIAN_POINT('Ctrl Pts',(-1.86981398314345,-1.,-0.765990708546111));
#39116=CARTESIAN_POINT('Ctrl Pts',(-1.86372027063314,-1.,-0.765891519092557));
#39117=CARTESIAN_POINT('Ctrl Pts',(-1.85764741390391,-1.,-0.765744212909305));
#39118=CARTESIAN_POINT('Ctrl Pts',(-1.85158945130054,-1.,-0.765545710619023));
#39119=CARTESIAN_POINT('Ctrl Pts',(-1.8455369887591,-1.,-0.765291664861971));
#39120=CARTESIAN_POINT('Ctrl Pts',(-1.83948181064823,-1.,-0.764978057881687));
#39121=CARTESIAN_POINT('Ctrl Pts',(-1.8334207722714,-1.,-0.764602549687845));
#39122=CARTESIAN_POINT('Ctrl Pts',(-1.8273599120008,-1.,-0.764165902606055));
#39123=CARTESIAN_POINT('Ctrl Pts',(-1.82131873145297,-1.,-0.763673465462854));
#39124=CARTESIAN_POINT('Ctrl Pts',(-1.81532118405566,-1.,-0.763132003836783));
#39125=CARTESIAN_POINT('Ctrl Pts',(-1.80938551463989,-1.,-0.762546129464036));
#39126=CARTESIAN_POINT('Ctrl Pts',(-1.80351583877334,-1.,-0.761915336443515));
#39127=CARTESIAN_POINT('Ctrl Pts',(-1.79768986997735,-1.,-0.761229695230359));
#39128=CARTESIAN_POINT('Ctrl Pts',(-1.79185815610802,-1.,-0.760469555880425));
#39129=CARTESIAN_POINT('Ctrl Pts',(-1.78596964884526,-1.,-0.759614401109868));
#39130=CARTESIAN_POINT('Ctrl Pts',(-1.77999411220912,-1.,-0.75865062667738));
#39131=CARTESIAN_POINT('Ctrl Pts',(-1.77394167108342,-1.,-0.757578264077238));
#39132=CARTESIAN_POINT('Ctrl Pts',(-1.76789396003141,-1.,-0.756421896028403));
#39133=CARTESIAN_POINT('Ctrl Pts',(-1.7619781724032,-1.,-0.755220979975262));
#39134=CARTESIAN_POINT('Ctrl Pts',(-1.75631083600175,-1.,-0.75400925402848));
#39135=CARTESIAN_POINT('Ctrl Pts',(-1.75095139468809,-1.,-0.752797683531377));
#39136=CARTESIAN_POINT('Ctrl Pts',(-1.74585086852298,-1.,-0.751555614163629));
#39137=CARTESIAN_POINT('Ctrl Pts',(-1.74080458266705,-1.,-0.75019343597954));
#39138=CARTESIAN_POINT('Ctrl Pts',(-1.73550351679848,-1.,-0.748582462954854));
#39139=CARTESIAN_POINT('Ctrl Pts',(-1.72958533647399,-1.,-0.746574710096436));
#39140=CARTESIAN_POINT('Ctrl Pts',(-1.7226822991693,-1.,-0.744021445433764));
#39141=CARTESIAN_POINT('Ctrl Pts',(-1.71447789751927,-1.,-0.740795162032087));
#39142=CARTESIAN_POINT('Ctrl Pts',(-1.70473309006121,-1.,-0.736799665724771));
#39143=CARTESIAN_POINT('Ctrl Pts',(-1.69326921975743,-1.,-0.731963238697195));
#39144=CARTESIAN_POINT('Ctrl Pts',(-1.67996158455503,-1.,-0.726235967997433));
#39145=CARTESIAN_POINT('Ctrl Pts',(-1.6647288055568,-1.,-0.719585433804282));
#39146=CARTESIAN_POINT('Ctrl Pts',(-1.64752408832016,-1.,-0.711993139355394));
#39147=CARTESIAN_POINT('Ctrl Pts',(-1.63216541664676,-1.,-0.705159151988319));
#39148=CARTESIAN_POINT('Ctrl Pts',(-1.61974673472612,-1.,-0.699605146405088));
#39149=CARTESIAN_POINT('Ctrl Pts',(-1.61106790958151,-1.,-0.695712097881194));
#39150=CARTESIAN_POINT('Ctrl Pts',(-1.60662857109684,-1.,-0.693717979106306));
#39151=CARTESIAN_POINT('',(-1.5055822144029,-1.,-0.892032620296855));
#39152=CARTESIAN_POINT('Origin',(0.,-1.,0.));
#39153=CARTESIAN_POINT('',(-1.81978687191668,-1.,-1.23627494547115));
#39154=CARTESIAN_POINT('Ctrl Pts',(-1.5055822144029,-1.,-0.892032620296855));
#39155=CARTESIAN_POINT('Ctrl Pts',(-1.50980486806688,-1.,-0.894452006964543));
#39156=CARTESIAN_POINT('Ctrl Pts',(-1.51805569590094,-1.,-0.899185047483511));
#39157=CARTESIAN_POINT('Ctrl Pts',(-1.52984849887993,-1.,-0.905967409625651));
#39158=CARTESIAN_POINT('Ctrl Pts',(-1.54440491149498,-1.,-0.914375919026456));
#39159=CARTESIAN_POINT('Ctrl Pts',(-1.56065988578893,-1.,-0.923832188944341));
#39160=CARTESIAN_POINT('Ctrl Pts',(-1.57499388382243,-1.,-0.932246680108685));
#39161=CARTESIAN_POINT('Ctrl Pts',(-1.58744937487176,-1.,-0.939646377893399));
#39162=CARTESIAN_POINT('Ctrl Pts',(-1.59810042043673,-1.,-0.946078063315257));
#39163=CARTESIAN_POINT('Ctrl Pts',(-1.60706069896936,-1.,-0.951613284356035));
#39164=CARTESIAN_POINT('Ctrl Pts',(-1.61449324337085,-1.,-0.956354422920671));
#39165=CARTESIAN_POINT('Ctrl Pts',(-1.62061638140221,-1.,-0.960438326101729));
#39166=CARTESIAN_POINT('Ctrl Pts',(-1.62571930670187,-1.,-0.964046107040536));
#39167=CARTESIAN_POINT('Ctrl Pts',(-1.63013849959461,-1.,-0.967387853230345));
#39168=CARTESIAN_POINT('Ctrl Pts',(-1.63420665729798,-1.,-0.970669715997509));
#39169=CARTESIAN_POINT('Ctrl Pts',(-1.63820952658144,-1.,-0.974066058287418));
#39170=CARTESIAN_POINT('Ctrl Pts',(-1.64233990826687,-1.,-0.977689794119416));
#39171=CARTESIAN_POINT('Ctrl Pts',(-1.64665139190656,-1.,-0.981562530939489));
#39172=CARTESIAN_POINT('Ctrl Pts',(-1.65110016612638,-1.,-0.985642622920821));
#39173=CARTESIAN_POINT('Ctrl Pts',(-1.65559044289699,-1.,-0.989855627854165));
#39174=CARTESIAN_POINT('Ctrl Pts',(-1.66001553809947,-1.,-0.994121836661306));
#39175=CARTESIAN_POINT('Ctrl Pts',(-1.66430758030376,-1.,-0.998389654952758));
#39176=CARTESIAN_POINT('Ctrl Pts',(-1.66846059277303,-1.,-1.00265091003727));
#39177=CARTESIAN_POINT('Ctrl Pts',(-1.67250335383293,-1.,-1.00692206696414));
#39178=CARTESIAN_POINT('Ctrl Pts',(-1.67648246776464,-1.,-1.01123236493511));
#39179=CARTESIAN_POINT('Ctrl Pts',(-1.68044289894798,-1.,-1.01561026162773));
#39180=CARTESIAN_POINT('Ctrl Pts',(-1.68440578021706,-1.,-1.02006795074201));
#39181=CARTESIAN_POINT('Ctrl Pts',(-1.68836910178447,-1.,-1.02460180535255));
#39182=CARTESIAN_POINT('Ctrl Pts',(-1.69231840863458,-1.,-1.02919977579147));
#39183=CARTESIAN_POINT('Ctrl Pts',(-1.69623414782771,-1.,-1.03384646003588));
#39184=CARTESIAN_POINT('Ctrl Pts',(-1.70010052930962,-1.,-1.03852922490789));
#39185=CARTESIAN_POINT('Ctrl Pts',(-1.70391338707982,-1.,-1.04324363334554));
#39186=CARTESIAN_POINT('Ctrl Pts',(-1.70767646263649,-1.,-1.04799085404995));
#39187=CARTESIAN_POINT('Ctrl Pts',(-1.71139783543989,-1.,-1.05277517202855));
#39188=CARTESIAN_POINT('Ctrl Pts',(-1.7150865442702,-1.,-1.05760163192479));
#39189=CARTESIAN_POINT('Ctrl Pts',(-1.71874858456904,-1.,-1.06247324680647));
#39190=CARTESIAN_POINT('Ctrl Pts',(-1.72238500928453,-1.,-1.06738966975462));
#39191=CARTESIAN_POINT('Ctrl Pts',(-1.72599406198488,-1.,-1.07234866990252));
#39192=CARTESIAN_POINT('Ctrl Pts',(-1.72957248977424,-1.,-1.0773470373727));
#39193=CARTESIAN_POINT('Ctrl Pts',(-1.73311705663407,-1.,-1.08238162784749));
#39194=CARTESIAN_POINT('Ctrl Pts',(-1.73662628326091,-1.,-1.08745056285427));
#39195=CARTESIAN_POINT('Ctrl Pts',(-1.74010053962247,-1.,-1.09255329056493));
#39196=CARTESIAN_POINT('Ctrl Pts',(-1.74354119236208,-1.,-1.09768999241225));
#39197=CARTESIAN_POINT('Ctrl Pts',(-1.74695004214923,-1.,-1.10286118991143));
#39198=CARTESIAN_POINT('Ctrl Pts',(-1.7503286607592,-1.,-1.10806728183007));
#39199=CARTESIAN_POINT('Ctrl Pts',(-1.7536777209463,-1.,-1.11330807582551));
#39200=CARTESIAN_POINT('Ctrl Pts',(-1.75699720772105,-1.,-1.11858293216763));
#39201=CARTESIAN_POINT('Ctrl Pts',(-1.76028671825096,-1.,-1.12389096855086));
#39202=CARTESIAN_POINT('Ctrl Pts',(-1.7635457196617,-1.,-1.12923123555075));
#39203=CARTESIAN_POINT('Ctrl Pts',(-1.76677384551862,-1.,-1.1346029180462));
#39204=CARTESIAN_POINT('Ctrl Pts',(-1.76997111386769,-1.,-1.14000548336975));
#39205=CARTESIAN_POINT('Ctrl Pts',(-1.77313777896194,-1.,-1.1454385822692));
#39206=CARTESIAN_POINT('Ctrl Pts',(-1.7762742255701,-1.,-1.15090197841515));
#39207=CARTESIAN_POINT('Ctrl Pts',(-1.77938085564275,-1.,-1.15639547194698));
#39208=CARTESIAN_POINT('Ctrl Pts',(-1.78245795881009,-1.,-1.16191881298499));
#39209=CARTESIAN_POINT('Ctrl Pts',(-1.78550566040443,-1.,-1.16747166312303));
#39210=CARTESIAN_POINT('Ctrl Pts',(-1.78852398877616,-1.,-1.17305363177328));
#39211=CARTESIAN_POINT('Ctrl Pts',(-1.79151291552689,-1.,-1.17866429440809));
#39212=CARTESIAN_POINT('Ctrl Pts',(-1.79447240321515,-1.,-1.18430321697432));
#39213=CARTESIAN_POINT('Ctrl Pts',(-1.79740245923478,-1.,-1.18996997934445));
#39214=CARTESIAN_POINT('Ctrl Pts',(-1.80030314369879,-1.,-1.19566418930242));
#39215=CARTESIAN_POINT('Ctrl Pts',(-1.80317454838603,-1.,-1.20138548938974));
#39216=CARTESIAN_POINT('Ctrl Pts',(-1.80601678480707,-1.,-1.20713356605475));
#39217=CARTESIAN_POINT('Ctrl Pts',(-1.80882996917129,-1.,-1.21290815708314));
#39218=CARTESIAN_POINT('Ctrl Pts',(-1.81161420806656,-1.,-1.21870906103557));
#39219=CARTESIAN_POINT('Ctrl Pts',(-1.81436959210434,-1.,-1.2245361330495));
#39220=CARTESIAN_POINT('Ctrl Pts',(-1.8165508718364,-1.,-1.2292186489137));
#39221=CARTESIAN_POINT('Ctrl Pts',(-1.81817389921279,-1.,-1.2327422452705));
#39222=CARTESIAN_POINT('Ctrl Pts',(-1.81925017193666,-1.,-1.23509651170476));
#39223=CARTESIAN_POINT('Ctrl Pts',(-1.81978687191668,-1.,-1.23627494547115));
#39224=CARTESIAN_POINT('',(-1.73811241238545,-1.,-1.34869019493419));
#39225=CARTESIAN_POINT('',(-1.81978687191668,-1.,-1.23627494547115));
#39226=CARTESIAN_POINT('',(-1.31362392696032,-1.,-1.15624053661742));
#39227=CARTESIAN_POINT('Ctrl Pts',(-1.73811241238545,-1.,-1.34869019493419));
#39228=CARTESIAN_POINT('Ctrl Pts',(-1.73682580585691,-1.,-1.34854391898045));
#39229=CARTESIAN_POINT('Ctrl Pts',(-1.73425417885907,-1.,-1.34824783112887));
#39230=CARTESIAN_POINT('Ctrl Pts',(-1.7304014965394,-1.,-1.34779309152035));
#39231=CARTESIAN_POINT('Ctrl Pts',(-1.72527410680674,-1.,-1.34716554819527));
#39232=CARTESIAN_POINT('Ctrl Pts',(-1.7188807715049,-1.,-1.34634568653227));
#39233=CARTESIAN_POINT('Ctrl Pts',(-1.71250340686822,-1.,-1.34549029589416));
#39234=CARTESIAN_POINT('Ctrl Pts',(-1.70614212266738,-1.,-1.34459924533831));
#39235=CARTESIAN_POINT('Ctrl Pts',(-1.69979707754427,-1.,-1.34367237124483));
#39236=CARTESIAN_POINT('Ctrl Pts',(-1.6934684849687,-1.,-1.34270948206319));
#39237=CARTESIAN_POINT('Ctrl Pts',(-1.68715660868764,-1.,-1.341710374848));
#39238=CARTESIAN_POINT('Ctrl Pts',(-1.68086176030362,-1.,-1.34067485185203));
#39239=CARTESIAN_POINT('Ctrl Pts',(-1.67458429426086,-1.,-1.3396027347034));
#39240=CARTESIAN_POINT('Ctrl Pts',(-1.66832460783989,-1.,-1.33849388654388));
#39241=CARTESIAN_POINT('Ctrl Pts',(-1.66208312541983,-1.,-1.33734820885262));
#39242=CARTESIAN_POINT('Ctrl Pts',(-1.65586025952593,-1.,-1.33616559745172));
#39243=CARTESIAN_POINT('Ctrl Pts',(-1.6496563728683,-1.,-1.33494590467993));
#39244=CARTESIAN_POINT('Ctrl Pts',(-1.6434717485603,-1.,-1.33368890676572));
#39245=CARTESIAN_POINT('Ctrl Pts',(-1.63730653475089,-1.,-1.33239425103724));
#39246=CARTESIAN_POINT('Ctrl Pts',(-1.63116079730923,-1.,-1.33106149345645));
#39247=CARTESIAN_POINT('Ctrl Pts',(-1.62503464209797,-1.,-1.3296901950568));
#39248=CARTESIAN_POINT('Ctrl Pts',(-1.61892832270724,-1.,-1.32828000610449));
#39249=CARTESIAN_POINT('Ctrl Pts',(-1.6128423401575,-1.,-1.32683074483356));
#39250=CARTESIAN_POINT('Ctrl Pts',(-1.60677758290954,-1.,-1.32534250785782));
#39251=CARTESIAN_POINT('Ctrl Pts',(-1.60073511858687,-1.,-1.32381550858256));
#39252=CARTESIAN_POINT('Ctrl Pts',(-1.59471591079403,-1.,-1.32224985747682));
#39253=CARTESIAN_POINT('Ctrl Pts',(-1.58872057258245,-1.,-1.32064537110892));
#39254=CARTESIAN_POINT('Ctrl Pts',(-1.58274907898834,-1.,-1.31900135021432));
#39255=CARTESIAN_POINT('Ctrl Pts',(-1.5768005650559,-1.,-1.31731642317187));
#39256=CARTESIAN_POINT('Ctrl Pts',(-1.57087397835723,-1.,-1.31558903860016));
#39257=CARTESIAN_POINT('Ctrl Pts',(-1.56496872402353,-1.,-1.31381795281002));
#39258=CARTESIAN_POINT('Ctrl Pts',(-1.55908521254821,-1.,-1.31200264341696));
#39259=CARTESIAN_POINT('Ctrl Pts',(-1.55322568759481,-1.,-1.31014393684222));
#39260=CARTESIAN_POINT('Ctrl Pts',(-1.54739413957185,-1.,-1.30824393907473));
#39261=CARTESIAN_POINT('Ctrl Pts',(-1.54159462645432,-1.,-1.30630475189556));
#39262=CARTESIAN_POINT('Ctrl Pts',(-1.53582981268977,-1.,-1.30432735639489));
#39263=CARTESIAN_POINT('Ctrl Pts',(-1.53009970283891,-1.,-1.30231064395568));
#39264=CARTESIAN_POINT('Ctrl Pts',(-1.52439957861062,-1.,-1.30024984366328));
#39265=CARTESIAN_POINT('Ctrl Pts',(-1.51872184912724,-1.,-1.29813791800747));
#39266=CARTESIAN_POINT('Ctrl Pts',(-1.51305994241402,-1.,-1.29596850710509));
#39267=CARTESIAN_POINT('Ctrl Pts',(-1.50741159078365,-1.,-1.29373841372842));
#39268=CARTESIAN_POINT('Ctrl Pts',(-1.50178230149776,-1.,-1.29145022885181));
#39269=CARTESIAN_POINT('Ctrl Pts',(-1.49618896881754,-1.,-1.28911506584254));
#39270=CARTESIAN_POINT('Ctrl Pts',(-1.4906522831278,-1.,-1.2867467611644));
#39271=CARTESIAN_POINT('Ctrl Pts',(-1.4851881711891,-1.,-1.28435533880201));
#39272=CARTESIAN_POINT('Ctrl Pts',(-1.47980070347095,-1.,-1.28194158939517));
#39273=CARTESIAN_POINT('Ctrl Pts',(-1.4744717526707,-1.,-1.2794891824849));
#39274=CARTESIAN_POINT('Ctrl Pts',(-1.46916035917133,-1.,-1.27696414831089));
#39275=CARTESIAN_POINT('Ctrl Pts',(-1.46382431332476,-1.,-1.27433119897822));
#39276=CARTESIAN_POINT('Ctrl Pts',(-1.45843906294697,-1.,-1.27156805265289));
#39277=CARTESIAN_POINT('Ctrl Pts',(-1.45301422764247,-1.,-1.2686778680489));
#39278=CARTESIAN_POINT('Ctrl Pts',(-1.44761985001662,-1.,-1.26570925118868));
#39279=CARTESIAN_POINT('Ctrl Pts',(-1.44236470511303,-1.,-1.26273903323859));
#39280=CARTESIAN_POINT('Ctrl Pts',(-1.43734919180848,-1.,-1.25983531012005));
#39281=CARTESIAN_POINT('Ctrl Pts',(-1.43262645609691,-1.,-1.25702687965755));
#39282=CARTESIAN_POINT('Ctrl Pts',(-1.42815938799387,-1.,-1.25426945222639));
#39283=CARTESIAN_POINT('Ctrl Pts',(-1.42378102115575,-1.,-1.2514145557001));
#39284=CARTESIAN_POINT('Ctrl Pts',(-1.41923722596025,-1.,-1.24824430986571));
#39285=CARTESIAN_POINT('Ctrl Pts',(-1.41422913175179,-1.,-1.24450600513056));
#39286=CARTESIAN_POINT('Ctrl Pts',(-1.40845295531283,-1.,-1.23994455029534));
#39287=CARTESIAN_POINT('Ctrl Pts',(-1.40164708206106,-1.,-1.23434087290423));
#39288=CARTESIAN_POINT('Ctrl Pts',(-1.39361389568796,-1.,-1.22752961899387));
#39289=CARTESIAN_POINT('Ctrl Pts',(-1.38420564527715,-1.,-1.21938737280852));
#39290=CARTESIAN_POINT('Ctrl Pts',(-1.37331915607905,-1.,-1.20982812925645));
#39291=CARTESIAN_POINT('Ctrl Pts',(-1.36088705043885,-1.,-1.1987959077932));
#39292=CARTESIAN_POINT('Ctrl Pts',(-1.34687054001093,-1.,-1.18625865667441));
#39293=CARTESIAN_POINT('Ctrl Pts',(-1.33437539347008,-1.,-1.17501305789857));
#39294=CARTESIAN_POINT('Ctrl Pts',(-1.32428080721772,-1.,-1.16589330093588));
#39295=CARTESIAN_POINT('Ctrl Pts',(-1.31722977216397,-1.,-1.15950888730809));
#39296=CARTESIAN_POINT('Ctrl Pts',(-1.31362392696032,-1.,-1.15624053661742));
#39297=CARTESIAN_POINT('',(-1.15624053661742,-1.,-1.31362392696033));
#39298=CARTESIAN_POINT('Origin',(0.,-1.,0.));
#39299=CARTESIAN_POINT('',(-1.34869019493419,-1.,-1.73811241238545));
#39300=CARTESIAN_POINT('Ctrl Pts',(-1.15624053661742,-1.,-1.31362392696033));
#39301=CARTESIAN_POINT('Ctrl Pts',(-1.15950888730433,-1.,-1.3172297721596));
#39302=CARTESIAN_POINT('Ctrl Pts',(-1.16589330092532,-1.,-1.32428080720544));
#39303=CARTESIAN_POINT('Ctrl Pts',(-1.17501305787994,-1.,-1.33437539344842));
#39304=CARTESIAN_POINT('Ctrl Pts',(-1.18625865664915,-1.,-1.34687053998157));
#39305=CARTESIAN_POINT('Ctrl Pts',(-1.1987959077656,-1.,-1.36088705040677));
#39306=CARTESIAN_POINT('Ctrl Pts',(-1.20982812923113,-1.,-1.37331915604962));
#39307=CARTESIAN_POINT('Ctrl Pts',(-1.21938737278853,-1.,-1.38420564525391));
#39308=CARTESIAN_POINT('Ctrl Pts',(-1.22752961898063,-1.,-1.39361389567257));
#39309=CARTESIAN_POINT('Ctrl Pts',(-1.23434087289768,-1.,-1.40164708205345));
#39310=CARTESIAN_POINT('Ctrl Pts',(-1.23994455029421,-1.,-1.40845295531151));
#39311=CARTESIAN_POINT('Ctrl Pts',(-1.24450600513278,-1.,-1.41422913175437));
#39312=CARTESIAN_POINT('Ctrl Pts',(-1.24824430986911,-1.,-1.41923722596421));
#39313=CARTESIAN_POINT('Ctrl Pts',(-1.25141455570299,-1.,-1.42378102115911));
#39314=CARTESIAN_POINT('Ctrl Pts',(-1.25426945222783,-1.,-1.42815938799555));
#39315=CARTESIAN_POINT('Ctrl Pts',(-1.25702687965744,-1.,-1.43262645609679));
#39316=CARTESIAN_POINT('Ctrl Pts',(-1.25983531011894,-1.,-1.43734919180719));
#39317=CARTESIAN_POINT('Ctrl Pts',(-1.26273903323723,-1.,-1.44236470511145));
#39318=CARTESIAN_POINT('Ctrl Pts',(-1.26570925118767,-1.,-1.44761985001544));
#39319=CARTESIAN_POINT('Ctrl Pts',(-1.26867786804854,-1.,-1.45301422764205));
#39320=CARTESIAN_POINT('Ctrl Pts',(-1.27156805265312,-1.,-1.45843906294725));
#39321=CARTESIAN_POINT('Ctrl Pts',(-1.27433119897877,-1.,-1.4638243133254));
#39322=CARTESIAN_POINT('Ctrl Pts',(-1.27696414831144,-1.,-1.46916035917197));
#39323=CARTESIAN_POINT('Ctrl Pts',(-1.27948918248524,-1.,-1.4744717526711));
#39324=CARTESIAN_POINT('Ctrl Pts',(-1.28194158939522,-1.,-1.47980070347102));
#39325=CARTESIAN_POINT('Ctrl Pts',(-1.28435533880184,-1.,-1.48518817118891));
#39326=CARTESIAN_POINT('Ctrl Pts',(-1.28674676116415,-1.,-1.4906522831275));
#39327=CARTESIAN_POINT('Ctrl Pts',(-1.28911506584232,-1.,-1.49618896881729));
#39328=CARTESIAN_POINT('Ctrl Pts',(-1.29145022885171,-1.,-1.50178230149764));
#39329=CARTESIAN_POINT('Ctrl Pts',(-1.29373841372843,-1.,-1.50741159078367));
#39330=CARTESIAN_POINT('Ctrl Pts',(-1.29596850710518,-1.,-1.51305994241412));
#39331=CARTESIAN_POINT('Ctrl Pts',(-1.29813791800757,-1.,-1.51872184912735));
#39332=CARTESIAN_POINT('Ctrl Pts',(-1.30024984366334,-1.,-1.5243995786107));
#39333=CARTESIAN_POINT('Ctrl Pts',(-1.3023106439557,-1.,-1.53009970283893));
#39334=CARTESIAN_POINT('Ctrl Pts',(-1.30432735639487,-1.,-1.53582981268976));
#39335=CARTESIAN_POINT('Ctrl Pts',(-1.30630475189553,-1.,-1.54159462645428));
#39336=CARTESIAN_POINT('Ctrl Pts',(-1.30824393907471,-1.,-1.54739413957183));
#39337=CARTESIAN_POINT('Ctrl Pts',(-1.31014393684221,-1.,-1.55322568759481));
#39338=CARTESIAN_POINT('Ctrl Pts',(-1.31200264341696,-1.,-1.55908521254822));
#39339=CARTESIAN_POINT('Ctrl Pts',(-1.31381795281002,-1.,-1.56496872402352));
#39340=CARTESIAN_POINT('Ctrl Pts',(-1.31558903860015,-1.,-1.57087397835721));
#39341=CARTESIAN_POINT('Ctrl Pts',(-1.31731642317183,-1.,-1.57680056505585));
#39342=CARTESIAN_POINT('Ctrl Pts',(-1.31900135021428,-1.,-1.58274907898829));
#39343=CARTESIAN_POINT('Ctrl Pts',(-1.32064537110891,-1.,-1.58872057258244));
#39344=CARTESIAN_POINT('Ctrl Pts',(-1.32224985747686,-1.,-1.59471591079408));
#39345=CARTESIAN_POINT('Ctrl Pts',(-1.32381550858266,-1.,-1.600735118587));
#39346=CARTESIAN_POINT('Ctrl Pts',(-1.32534250785794,-1.,-1.6067775829097));
#39347=CARTESIAN_POINT('Ctrl Pts',(-1.32683074483365,-1.,-1.61284234015762));
#39348=CARTESIAN_POINT('Ctrl Pts',(-1.32828000610448,-1.,-1.61892832270723));
#39349=CARTESIAN_POINT('Ctrl Pts',(-1.32969019505665,-1.,-1.62503464209777));
#39350=CARTESIAN_POINT('Ctrl Pts',(-1.33106149345618,-1.,-1.63116079730887));
#39351=CARTESIAN_POINT('Ctrl Pts',(-1.33239425103694,-1.,-1.6373065347505));
#39352=CARTESIAN_POINT('Ctrl Pts',(-1.33368890676554,-1.,-1.64347174856007));
#39353=CARTESIAN_POINT('Ctrl Pts',(-1.33494590468003,-1.,-1.64965637286843));
#39354=CARTESIAN_POINT('Ctrl Pts',(-1.33616559745217,-1.,-1.65586025952651));
#39355=CARTESIAN_POINT('Ctrl Pts',(-1.33734820885331,-1.,-1.66208312542073));
#39356=CARTESIAN_POINT('Ctrl Pts',(-1.33849388654458,-1.,-1.66832460784078));
#39357=CARTESIAN_POINT('Ctrl Pts',(-1.33960273470372,-1.,-1.67458429426126));
#39358=CARTESIAN_POINT('Ctrl Pts',(-1.3406748518516,-1.,-1.68086176030308));
#39359=CARTESIAN_POINT('Ctrl Pts',(-1.34171037484673,-1.,-1.68715660868602));
#39360=CARTESIAN_POINT('Ctrl Pts',(-1.34270948206139,-1.,-1.6934684849664));
#39361=CARTESIAN_POINT('Ctrl Pts',(-1.34367237124322,-1.,-1.69979707754221));
#39362=CARTESIAN_POINT('Ctrl Pts',(-1.34459924533783,-1.,-1.70614212266676));
#39363=CARTESIAN_POINT('Ctrl Pts',(-1.34549029589563,-1.,-1.71250340687011));
#39364=CARTESIAN_POINT('Ctrl Pts',(-1.34634568653586,-1.,-1.7188807715095));
#39365=CARTESIAN_POINT('Ctrl Pts',(-1.34716554820013,-1.,-1.72527410681298));
#39366=CARTESIAN_POINT('Ctrl Pts',(-1.3477930915247,-1.,-1.73040149654497));
#39367=CARTESIAN_POINT('Ctrl Pts',(-1.34824783113158,-1.,-1.73425417886255));
#39368=CARTESIAN_POINT('Ctrl Pts',(-1.34854391898145,-1.,-1.73682580585819));
#39369=CARTESIAN_POINT('Ctrl Pts',(-1.34869019493419,-1.,-1.73811241238545));
#39370=CARTESIAN_POINT('',(-1.23627494547115,-1.,-1.81978687191668));
#39371=CARTESIAN_POINT('',(-1.34869019493419,-1.,-1.73811241238545));
#39372=CARTESIAN_POINT('',(-0.892032620296855,-1.,-1.5055822144029));
#39373=CARTESIAN_POINT('Ctrl Pts',(-1.23627494547115,-1.,-1.81978687191668));
#39374=CARTESIAN_POINT('Ctrl Pts',(-1.23509651170384,-1.,-1.81925017193531));
#39375=CARTESIAN_POINT('Ctrl Pts',(-1.23274224526804,-1.,-1.81817389920914));
#39376=CARTESIAN_POINT('Ctrl Pts',(-1.22921864890975,-1.,-1.81655087183054));
#39377=CARTESIAN_POINT('Ctrl Pts',(-1.22453613304507,-1.,-1.81436959209778));
#39378=CARTESIAN_POINT('Ctrl Pts',(-1.2187090610323,-1.,-1.81161420806172));
#39379=CARTESIAN_POINT('Ctrl Pts',(-1.2129081570818,-1.,-1.80882996916931));
#39380=CARTESIAN_POINT('Ctrl Pts',(-1.20713356605519,-1.,-1.80601678480772));
#39381=CARTESIAN_POINT('Ctrl Pts',(-1.2013854893912,-1.,-1.8031745483882));
#39382=CARTESIAN_POINT('Ctrl Pts',(-1.19566418930405,-1.,-1.80030314370121));
#39383=CARTESIAN_POINT('Ctrl Pts',(-1.1899699793456,-1.,-1.79740245923649));
#39384=CARTESIAN_POINT('Ctrl Pts',(-1.18430321697471,-1.,-1.79447240321572));
#39385=CARTESIAN_POINT('Ctrl Pts',(-1.17866429440781,-1.,-1.79151291552646));
#39386=CARTESIAN_POINT('Ctrl Pts',(-1.17305363177265,-1.,-1.78852398877523));
#39387=CARTESIAN_POINT('Ctrl Pts',(-1.16747166312239,-1.,-1.78550566040349));
#39388=CARTESIAN_POINT('Ctrl Pts',(-1.16191881298458,-1.,-1.78245795880949));
#39389=CARTESIAN_POINT('Ctrl Pts',(-1.15639547194689,-1.,-1.77938085564261));
#39390=CARTESIAN_POINT('Ctrl Pts',(-1.15090197841531,-1.,-1.77627422557034));
#39391=CARTESIAN_POINT('Ctrl Pts',(-1.14543858226948,-1.,-1.77313777896234));
#39392=CARTESIAN_POINT('Ctrl Pts',(-1.14000548337,-1.,-1.76997111386806));
#39393=CARTESIAN_POINT('Ctrl Pts',(-1.13460291804635,-1.,-1.76677384551883));
#39394=CARTESIAN_POINT('Ctrl Pts',(-1.12923123555076,-1.,-1.76354571966171));
#39395=CARTESIAN_POINT('Ctrl Pts',(-1.12389096855078,-1.,-1.76028671825084));
#39396=CARTESIAN_POINT('Ctrl Pts',(-1.11858293216752,-1.,-1.75699720772089));
#39397=CARTESIAN_POINT('Ctrl Pts',(-1.11330807582542,-1.,-1.75367772094617));
#39398=CARTESIAN_POINT('Ctrl Pts',(-1.10806728183003,-1.,-1.75032866075914));
#39399=CARTESIAN_POINT('Ctrl Pts',(-1.10286118991144,-1.,-1.74695004214924));
#39400=CARTESIAN_POINT('Ctrl Pts',(-1.09768999241229,-1.,-1.74354119236212));
#39401=CARTESIAN_POINT('Ctrl Pts',(-1.09255329056496,-1.,-1.74010053962252));
#39402=CARTESIAN_POINT('Ctrl Pts',(-1.08745056285429,-1.,-1.73662628326093));
#39403=CARTESIAN_POINT('Ctrl Pts',(-1.08238162784749,-1.,-1.73311705663407));
#39404=CARTESIAN_POINT('Ctrl Pts',(-1.0773470373727,-1.,-1.72957248977424));
#39405=CARTESIAN_POINT('Ctrl Pts',(-1.07234866990252,-1.,-1.72599406198489));
#39406=CARTESIAN_POINT('Ctrl Pts',(-1.06738966975463,-1.,-1.72238500928456));
#39407=CARTESIAN_POINT('Ctrl Pts',(-1.0624732468065,-1.,-1.71874858456908));
#39408=CARTESIAN_POINT('Ctrl Pts',(-1.05760163192481,-1.,-1.71508654427022));
#39409=CARTESIAN_POINT('Ctrl Pts',(-1.05277517202854,-1.,-1.71139783543986));
#39410=CARTESIAN_POINT('Ctrl Pts',(-1.0479908540499,-1.,-1.70767646263641));
#39411=CARTESIAN_POINT('Ctrl Pts',(-1.04324363334546,-1.,-1.70391338707969));
#39412=CARTESIAN_POINT('Ctrl Pts',(-1.03852922490782,-1.,-1.70010052930951));
#39413=CARTESIAN_POINT('Ctrl Pts',(-1.03384646003587,-1.,-1.69623414782769));
#39414=CARTESIAN_POINT('Ctrl Pts',(-1.02919977579155,-1.,-1.69231840863471));
#39415=CARTESIAN_POINT('Ctrl Pts',(-1.02460180535272,-1.,-1.68836910178475));
#39416=CARTESIAN_POINT('Ctrl Pts',(-1.02006795074222,-1.,-1.68440578021739));
#39417=CARTESIAN_POINT('Ctrl Pts',(-1.01561026162787,-1.,-1.6804428989482));
#39418=CARTESIAN_POINT('Ctrl Pts',(-1.01123236493507,-1.,-1.67648246776457));
#39419=CARTESIAN_POINT('Ctrl Pts',(-1.00692206696387,-1.,-1.67250335383248));
#39420=CARTESIAN_POINT('Ctrl Pts',(-1.00265091003682,-1.,-1.66846059277231));
#39421=CARTESIAN_POINT('Ctrl Pts',(-0.998389654952317,-1.,-1.66430758030304));
#39422=CARTESIAN_POINT('Ctrl Pts',(-0.994121836661116,-1.,-1.66001553809916));
#39423=CARTESIAN_POINT('Ctrl Pts',(-0.98985562785445,-1.,-1.65559044289746));
#39424=CARTESIAN_POINT('Ctrl Pts',(-0.985642622921626,-1.,-1.6511001661277));
#39425=CARTESIAN_POINT('Ctrl Pts',(-0.981562530940574,-1.,-1.64665139190834));
#39426=CARTESIAN_POINT('Ctrl Pts',(-0.977689794120297,-1.,-1.64233990826831));
#39427=CARTESIAN_POINT('Ctrl Pts',(-0.974066058287501,-1.,-1.63820952658157));
#39428=CARTESIAN_POINT('Ctrl Pts',(-0.970669715996356,-1.,-1.63420665729609));
#39429=CARTESIAN_POINT('Ctrl Pts',(-0.967387853228041,-1.,-1.63013849959083));
#39430=CARTESIAN_POINT('Ctrl Pts',(-0.964046107037821,-1.,-1.6257193066974));
#39431=CARTESIAN_POINT('Ctrl Pts',(-0.960438326099958,-1.,-1.62061638139929));
#39432=CARTESIAN_POINT('Ctrl Pts',(-0.956354422921573,-1.,-1.61449324337233));
#39433=CARTESIAN_POINT('Ctrl Pts',(-0.951613284361248,-1.,-1.60706069897794));
#39434=CARTESIAN_POINT('Ctrl Pts',(-0.946078063325796,-1.,-1.59810042045408));
#39435=CARTESIAN_POINT('Ctrl Pts',(-0.939646377909319,-1.,-1.58744937489796));
#39436=CARTESIAN_POINT('Ctrl Pts',(-0.932246680128849,-1.,-1.57499388385561));
#39437=CARTESIAN_POINT('Ctrl Pts',(-0.923832188966322,-1.,-1.56065988582509));
#39438=CARTESIAN_POINT('Ctrl Pts',(-0.91437591904658,-1.,-1.54440491152808));
#39439=CARTESIAN_POINT('Ctrl Pts',(-0.905967409640499,-1.,-1.52984849890434));
#39440=CARTESIAN_POINT('Ctrl Pts',(-0.89918504749193,-1.,-1.51805569591479));
#39441=CARTESIAN_POINT('Ctrl Pts',(-0.894452006967538,-1.,-1.50980486807181));
#39442=CARTESIAN_POINT('Ctrl Pts',(-0.892032620296855,-1.,-1.5055822144029));
#39443=CARTESIAN_POINT('',(-0.693717979106305,-1.,-1.60662857109684));
#39444=CARTESIAN_POINT('Origin',(0.,-1.,0.));
#39445=CARTESIAN_POINT('',(-0.745574324794401,-1.,-2.0698113262342));
#39446=CARTESIAN_POINT('Ctrl Pts',(-0.693717979106305,-1.,-1.60662857109684));
#39447=CARTESIAN_POINT('Ctrl Pts',(-0.69571209787897,-1.,-1.61106790957619));
#39448=CARTESIAN_POINT('Ctrl Pts',(-0.699605146398837,-1.,-1.61974673471117));
#39449=CARTESIAN_POINT('Ctrl Pts',(-0.705159151977294,-1.,-1.6321654166204));
#39450=CARTESIAN_POINT('Ctrl Pts',(-0.711993139340447,-1.,-1.64752408828442));
#39451=CARTESIAN_POINT('Ctrl Pts',(-0.71958543378795,-1.,-1.66472880551777));
#39452=CARTESIAN_POINT('Ctrl Pts',(-0.726235967982445,-1.,-1.67996158451922));
#39453=CARTESIAN_POINT('Ctrl Pts',(-0.731963238685357,-1.,-1.69326921972915));
#39454=CARTESIAN_POINT('Ctrl Pts',(-0.736799665716932,-1.,-1.70473309004249));
#39455=CARTESIAN_POINT('Ctrl Pts',(-0.74079516202821,-1.,-1.71447789751001));
#39456=CARTESIAN_POINT('Ctrl Pts',(-0.744021445433093,-1.,-1.72268229916769));
#39457=CARTESIAN_POINT('Ctrl Pts',(-0.746574710097752,-1.,-1.72958533647714));
#39458=CARTESIAN_POINT('Ctrl Pts',(-0.74858246295687,-1.,-1.7355035168033));
#39459=CARTESIAN_POINT('Ctrl Pts',(-0.750193435981249,-1.,-1.74080458267114));
#39460=CARTESIAN_POINT('Ctrl Pts',(-0.751555614164482,-1.,-1.74585086852502));
#39461=CARTESIAN_POINT('Ctrl Pts',(-0.752797683531314,-1.,-1.75095139468794));
#39462=CARTESIAN_POINT('Ctrl Pts',(-0.754009254027829,-1.,-1.75631083600019));
#39463=CARTESIAN_POINT('Ctrl Pts',(-0.755220979974461,-1.,-1.76197817240128));
#39464=CARTESIAN_POINT('Ctrl Pts',(-0.75642189602781,-1.,-1.76789396002998));
#39465=CARTESIAN_POINT('Ctrl Pts',(-0.757578264077029,-1.,-1.77394167108292));
#39466=CARTESIAN_POINT('Ctrl Pts',(-0.758650626677518,-1.,-1.77999411220945));
#39467=CARTESIAN_POINT('Ctrl Pts',(-0.759614401110189,-1.,-1.78596964884604));
#39468=CARTESIAN_POINT('Ctrl Pts',(-0.760469555880749,-1.,-1.7918581561088));
#39469=CARTESIAN_POINT('Ctrl Pts',(-0.761229695230558,-1.,-1.79768986997783));
#39470=CARTESIAN_POINT('Ctrl Pts',(-0.761915336443547,-1.,-1.80351583877342));
#39471=CARTESIAN_POINT('Ctrl Pts',(-0.762546129463938,-1.,-1.80938551463965));
#39472=CARTESIAN_POINT('Ctrl Pts',(-0.763132003836634,-1.,-1.8153211840553));
#39473=CARTESIAN_POINT('Ctrl Pts',(-0.763673465462726,-1.,-1.82131873145266));
#39474=CARTESIAN_POINT('Ctrl Pts',(-0.764165902605995,-1.,-1.82735991200065));
#39475=CARTESIAN_POINT('Ctrl Pts',(-0.764602549687853,-1.,-1.83342077227142));
#39476=CARTESIAN_POINT('Ctrl Pts',(-0.764978057881737,-1.,-1.83948181064835));
#39477=CARTESIAN_POINT('Ctrl Pts',(-0.765291664862029,-1.,-1.84553698875924));
#39478=CARTESIAN_POINT('Ctrl Pts',(-0.765545710619062,-1.,-1.85158945130063));
#39479=CARTESIAN_POINT('Ctrl Pts',(-0.765744212909318,-1.,-1.85764741390394));
#39480=CARTESIAN_POINT('Ctrl Pts',(-0.765891519092547,-1.,-1.86372027063312));
#39481=CARTESIAN_POINT('Ctrl Pts',(-0.765990708546091,-1.,-1.86981398314341));
#39482=CARTESIAN_POINT('Ctrl Pts',(-0.766042837036744,-1.,-1.87592888967883));
#39483=CARTESIAN_POINT('Ctrl Pts',(-0.766047794851865,-1.,-1.88206215302561));
#39484=CARTESIAN_POINT('Ctrl Pts',(-0.766004837062091,-1.,-1.88820926433409));
#39485=CARTESIAN_POINT('Ctrl Pts',(-0.765913193856978,-1.,-1.89436577771388));
#39486=CARTESIAN_POINT('Ctrl Pts',(-0.765772772593386,-1.,-1.90052930393596));
#39487=CARTESIAN_POINT('Ctrl Pts',(-0.765584196937919,-1.,-1.90669961402356));
#39488=CARTESIAN_POINT('Ctrl Pts',(-0.765348465884722,-1.,-1.91287765805169));
#39489=CARTESIAN_POINT('Ctrl Pts',(-0.765066729667088,-1.,-1.91906491634196));
#39490=CARTESIAN_POINT('Ctrl Pts',(-0.764740025488211,-1.,-1.92526263537048));
#39491=CARTESIAN_POINT('Ctrl Pts',(-0.764369010673941,-1.,-1.93147105496382));
#39492=CARTESIAN_POINT('Ctrl Pts',(-0.763954049121458,-1.,-1.93768964875886));
#39493=CARTESIAN_POINT('Ctrl Pts',(-0.763495333538629,-1.,-1.9439174661764));
#39494=CARTESIAN_POINT('Ctrl Pts',(-0.762992990878769,-1.,-1.95015342590024));
#39495=CARTESIAN_POINT('Ctrl Pts',(-0.762447203806179,-1.,-1.95639665309869));
#39496=CARTESIAN_POINT('Ctrl Pts',(-0.761858300014423,-1.,-1.96264672744186));
#39497=CARTESIAN_POINT('Ctrl Pts',(-0.76122669048382,-1.,-1.96890351582499));
#39498=CARTESIAN_POINT('Ctrl Pts',(-0.760552825409757,-1.,-1.97516705321494));
#39499=CARTESIAN_POINT('Ctrl Pts',(-0.75983714745219,-1.,-1.98143741418172));
#39500=CARTESIAN_POINT('Ctrl Pts',(-0.759080037802488,-1.,-1.98771456680874));
#39501=CARTESIAN_POINT('Ctrl Pts',(-0.758281796766761,-1.,-1.99399831098817));
#39502=CARTESIAN_POINT('Ctrl Pts',(-0.757442676862724,-1.,-2.00028834739178));
#39503=CARTESIAN_POINT('Ctrl Pts',(-0.75656290464667,-1.,-2.0065843158773));
#39504=CARTESIAN_POINT('Ctrl Pts',(-0.755642704957865,-1.,-2.01288584328084));
#39505=CARTESIAN_POINT('Ctrl Pts',(-0.754682330722816,-1.,-2.01919259405809));
#39506=CARTESIAN_POINT('Ctrl Pts',(-0.753682061112768,-1.,-2.02550428623313));
#39507=CARTESIAN_POINT('Ctrl Pts',(-0.752642180487211,-1.,-2.03182068456221));
#39508=CARTESIAN_POINT('Ctrl Pts',(-0.751562963361115,-1.,-2.03814160092099));
#39509=CARTESIAN_POINT('Ctrl Pts',(-0.750444657875576,-1.,-2.04446689147979));
#39510=CARTESIAN_POINT('Ctrl Pts',(-0.749287468665046,-1.,-2.05079645592154));
#39511=CARTESIAN_POINT('Ctrl Pts',(-0.748091554183802,-1.,-2.05713023031006));
#39512=CARTESIAN_POINT('Ctrl Pts',(-0.747103932787919,-1.,-2.06220058927826));
#39513=CARTESIAN_POINT('Ctrl Pts',(-0.7463458715442,-1.,-2.06600523016815));
#39514=CARTESIAN_POINT('Ctrl Pts',(-0.745832791378367,-1.,-2.06854248895728));
#39515=CARTESIAN_POINT('Ctrl Pts',(-0.745574324794401,-1.,-2.0698113262342));
#39516=CARTESIAN_POINT('',(-0.61342227326009,-1.,-2.11275013067528));
#39517=CARTESIAN_POINT('',(-0.745574324794401,-1.,-2.0698113262342));
#39518=CARTESIAN_POINT('',(-0.383122945602004,-1.,-1.7075470150345));
#39519=CARTESIAN_POINT('Ctrl Pts',(-0.61342227326009,-1.,-2.11275013067528));
#39520=CARTESIAN_POINT('Ctrl Pts',(-0.6124673655618,-1.,-2.11187554259986));
#39521=CARTESIAN_POINT('Ctrl Pts',(-0.610560911689899,-1.,-2.11012443807238));
#39522=CARTESIAN_POINT('Ctrl Pts',(-0.607711315454876,-1.,-2.1074919961518));
#39523=CARTESIAN_POINT('Ctrl Pts',(-0.60393203073603,-1.,-2.10397049886949));
#39524=CARTESIAN_POINT('Ctrl Pts',(-0.599241616420533,-1.,-2.0995493086477));
#39525=CARTESIAN_POINT('Ctrl Pts',(-0.594585006052162,-1.,-2.0951087622027));
#39526=CARTESIAN_POINT('Ctrl Pts',(-0.589962365403406,-1.,-2.09064881812129));
#39527=CARTESIAN_POINT('Ctrl Pts',(-0.585373918991617,-1.,-2.08616943727951));
#39528=CARTESIAN_POINT('Ctrl Pts',(-0.580819952108063,-1.,-2.08167059018418));
#39529=CARTESIAN_POINT('Ctrl Pts',(-0.576300797416844,-1.,-2.07715226767559));
#39530=CARTESIAN_POINT('Ctrl Pts',(-0.571816823242603,-1.,-2.07261449292824));
#39531=CARTESIAN_POINT('Ctrl Pts',(-0.567368421181087,-1.,-2.06805732997334));
#39532=CARTESIAN_POINT('Ctrl Pts',(-0.562955993082261,-1.,-2.06348090160589));
#39533=CARTESIAN_POINT('Ctrl Pts',(-0.558579940185151,-1.,-2.05888537756462));
#39534=CARTESIAN_POINT('Ctrl Pts',(-0.554240657463906,-1.,-2.05427091604413));
#39535=CARTESIAN_POINT('Ctrl Pts',(-0.549938525150295,-1.,-2.04963761077958));
#39536=CARTESIAN_POINT('Ctrl Pts',(-0.54567390381743,-1.,-2.04498544714588));
#39537=CARTESIAN_POINT('Ctrl Pts',(-0.541447120615659,-1.,-2.04031422690527));
#39538=CARTESIAN_POINT('Ctrl Pts',(-0.537258489833262,-1.,-2.03562362954037));
#39539=CARTESIAN_POINT('Ctrl Pts',(-0.533108355132977,-1.,-2.03091336214426));
#39540=CARTESIAN_POINT('Ctrl Pts',(-0.528997127241914,-1.,-2.0261832908329));
#39541=CARTESIAN_POINT('Ctrl Pts',(-0.524925318333476,-1.,-2.02143356304698));
#39542=CARTESIAN_POINT('Ctrl Pts',(-0.52089359039937,-1.,-2.01666477917286));
#39543=CARTESIAN_POINT('Ctrl Pts',(-0.516902681728687,-1.,-2.01187773939242));
#39544=CARTESIAN_POINT('Ctrl Pts',(-0.512953306961792,-1.,-2.00707309946949));
#39545=CARTESIAN_POINT('Ctrl Pts',(-0.509046069886157,-1.,-2.00225107134734));
#39546=CARTESIAN_POINT('Ctrl Pts',(-0.505181361323026,-1.,-1.99741107463572));
#39547=CARTESIAN_POINT('Ctrl Pts',(-0.501359287727146,-1.,-1.99255149126155));
#39548=CARTESIAN_POINT('Ctrl Pts',(-0.497579909545574,-1.,-1.98767044752932));
#39549=CARTESIAN_POINT('Ctrl Pts',(-0.493843476541495,-1.,-1.98276658761821));
#39550=CARTESIAN_POINT('Ctrl Pts',(-0.490150627860952,-1.,-1.97783973019229));
#39551=CARTESIAN_POINT('Ctrl Pts',(-0.486502692907659,-1.,-1.97289186263272));
#39552=CARTESIAN_POINT('Ctrl Pts',(-0.482901662120691,-1.,-1.96792703422362));
#39553=CARTESIAN_POINT('Ctrl Pts',(-0.479349583074855,-1.,-1.96294933055943));
#39554=CARTESIAN_POINT('Ctrl Pts',(-0.475848034683176,-1.,-1.95796111148177));
#39555=CARTESIAN_POINT('Ctrl Pts',(-0.472397672264072,-1.,-1.95296148278133));
#39556=CARTESIAN_POINT('Ctrl Pts',(-0.468997482913135,-1.,-1.94794381136514));
#39557=CARTESIAN_POINT('Ctrl Pts',(-0.46564546202603,-1.,-1.9428979419619));
#39558=CARTESIAN_POINT('Ctrl Pts',(-0.462340031009056,-1.,-1.93781486640821));
#39559=CARTESIAN_POINT('Ctrl Pts',(-0.459081234547926,-1.,-1.93269066517934));
#39560=CARTESIAN_POINT('Ctrl Pts',(-0.455872005174371,-1.,-1.92753067150476));
#39561=CARTESIAN_POINT('Ctrl Pts',(-0.452719478359432,-1.,-1.92235380648502));
#39562=CARTESIAN_POINT('Ctrl Pts',(-0.449632260106662,-1.,-1.91718342555755));
#39563=CARTESIAN_POINT('Ctrl Pts',(-0.446617343485711,-1.,-1.9120369998112));
#39564=CARTESIAN_POINT('Ctrl Pts',(-0.443677556849151,-1.,-1.90691756144898));
#39565=CARTESIAN_POINT('Ctrl Pts',(-0.440807833704038,-1.,-1.90180124389086));
#39566=CARTESIAN_POINT('Ctrl Pts',(-0.437995003948244,-1.,-1.89663648956466));
#39567=CARTESIAN_POINT('Ctrl Pts',(-0.435225660963383,-1.,-1.89136993975504));
#39568=CARTESIAN_POINT('Ctrl Pts',(-0.432493038548748,-1.,-1.88596913666793));
#39569=CARTESIAN_POINT('Ctrl Pts',(-0.429803062482344,-1.,-1.88044229001832));
#39570=CARTESIAN_POINT('Ctrl Pts',(-0.427183828519102,-1.,-1.87486989291484));
#39571=CARTESIAN_POINT('Ctrl Pts',(-0.424678177291359,-1.,-1.86937803944323));
#39572=CARTESIAN_POINT('Ctrl Pts',(-0.422327307418275,-1.,-1.86408083334028));
#39573=CARTESIAN_POINT('Ctrl Pts',(-0.420157287975619,-1.,-1.85903281096686));
#39574=CARTESIAN_POINT('Ctrl Pts',(-0.418164129143534,-1.,-1.85417632856234));
#39575=CARTESIAN_POINT('Ctrl Pts',(-0.416300022038864,-1.,-1.84929312929882));
#39576=CARTESIAN_POINT('Ctrl Pts',(-0.41448743825434,-1.,-1.8440575707371));
#39577=CARTESIAN_POINT('Ctrl Pts',(-0.412633125322162,-1.,-1.83808953475839));
#39578=CARTESIAN_POINT('Ctrl Pts',(-0.410641256301675,-1.,-1.83100408895216));
#39579=CARTESIAN_POINT('Ctrl Pts',(-0.408428948108533,-1.,-1.8224702267854));
#39580=CARTESIAN_POINT('Ctrl Pts',(-0.405933518411838,-1.,-1.81223801813988));
#39581=CARTESIAN_POINT('Ctrl Pts',(-0.403107976170441,-1.,-1.80012077176221));
#39582=CARTESIAN_POINT('Ctrl Pts',(-0.39991940378308,-1.,-1.78598826347533));
#39583=CARTESIAN_POINT('Ctrl Pts',(-0.39634619612042,-1.,-1.7697556004756));
#39584=CARTESIAN_POINT('Ctrl Pts',(-0.392375812294307,-1.,-1.75137405313962));
#39585=CARTESIAN_POINT('Ctrl Pts',(-0.388877023509191,-1.,-1.7349317097561));
#39586=CARTESIAN_POINT('Ctrl Pts',(-0.38607079032701,-1.,-1.72162022246158));
#39587=CARTESIAN_POINT('Ctrl Pts',(-0.384119047315542,-1.,-1.71231062891958));
#39588=CARTESIAN_POINT('Ctrl Pts',(-0.383122945602004,-1.,-1.7075470150345));
#39589=CARTESIAN_POINT('',(-0.163289472382896,-1.,-1.74236521665491));
#39590=CARTESIAN_POINT('Origin',(0.,-1.,0.));
#39591=CARTESIAN_POINT('',(-0.0694764450219581,-1.,-2.19890268624765));
#39592=CARTESIAN_POINT('Ctrl Pts',(-0.163289472382896,-1.,-1.74236521665491));
#39593=CARTESIAN_POINT('Ctrl Pts',(-0.163814161002002,-1.,-1.7472034950333));
#39594=CARTESIAN_POINT('Ctrl Pts',(-0.164834765707158,-1.,-1.75666056638427));
#39595=CARTESIAN_POINT('Ctrl Pts',(-0.1662793551464,-1.,-1.77018771684844));
#39596=CARTESIAN_POINT('Ctrl Pts',(-0.168032772805197,-1.,-1.7869064998507));
#39597=CARTESIAN_POINT('Ctrl Pts',(-0.169936923904608,-1.,-1.80561530629706));
#39598=CARTESIAN_POINT('Ctrl Pts',(-0.171554770204119,-1.,-1.82215766811545));
#39599=CARTESIAN_POINT('Ctrl Pts',(-0.1728894428919,-1.,-1.83658380527692));
#39600=CARTESIAN_POINT('Ctrl Pts',(-0.173946627587731,-1.,-1.8489811319852));
#39601=CARTESIAN_POINT('Ctrl Pts',(-0.17473525927603,-1.,-1.85948367088837));
#39602=CARTESIAN_POINT('Ctrl Pts',(-0.175268337590758,-1.,-1.86828349694799));
#39603=CARTESIAN_POINT('Ctrl Pts',(-0.175563480746485,-1.,-1.87563767773588));
#39604=CARTESIAN_POINT('Ctrl Pts',(-0.175644148889699,-1.,-1.88188663145367));
#39605=CARTESIAN_POINT('Ctrl Pts',(-0.175538155840648,-1.,-1.88742606273259));
#39606=CARTESIAN_POINT('Ctrl Pts',(-0.175274276190844,-1.,-1.892646301985));
#39607=CARTESIAN_POINT('Ctrl Pts',(-0.174879405091263,-1.,-1.89788101117132));
#39608=CARTESIAN_POINT('Ctrl Pts',(-0.174375518661085,-1.,-1.90335253862834));
#39609=CARTESIAN_POINT('Ctrl Pts',(-0.173776635257817,-1.,-1.90911693975267));
#39610=CARTESIAN_POINT('Ctrl Pts',(-0.173090695383496,-1.,-1.91511429159527));
#39611=CARTESIAN_POINT('Ctrl Pts',(-0.172321621259514,-1.,-1.9212233439798));
#39612=CARTESIAN_POINT('Ctrl Pts',(-0.171471191532988,-1.,-1.92731093582036));
#39613=CARTESIAN_POINT('Ctrl Pts',(-0.170541253116202,-1.,-1.93329183155539));
#39614=CARTESIAN_POINT('Ctrl Pts',(-0.169534904817491,-1.,-1.93915639211581));
#39615=CARTESIAN_POINT('Ctrl Pts',(-0.168455741607556,-1.,-1.94493757756931));
#39616=CARTESIAN_POINT('Ctrl Pts',(-0.167307501784475,-1.,-1.95069027794294));
#39617=CARTESIAN_POINT('Ctrl Pts',(-0.166093592002812,-1.,-1.9564675971873));
#39618=CARTESIAN_POINT('Ctrl Pts',(-0.164816568920269,-1.,-1.96229379940136));
#39619=CARTESIAN_POINT('Ctrl Pts',(-0.163478185457734,-1.,-1.96816512677967));
#39620=CARTESIAN_POINT('Ctrl Pts',(-0.162079693556289,-1.,-1.97406280235188));
#39621=CARTESIAN_POINT('Ctrl Pts',(-0.160622060784611,-1.,-1.97996195437559));
#39622=CARTESIAN_POINT('Ctrl Pts',(-0.159106226437299,-1.,-1.98584238283292));
#39623=CARTESIAN_POINT('Ctrl Pts',(-0.157533331459227,-1.,-1.99169810931908));
#39624=CARTESIAN_POINT('Ctrl Pts',(-0.155904629548783,-1.,-1.99753284771497));
#39625=CARTESIAN_POINT('Ctrl Pts',(-0.154221403049722,-1.,-2.00335565310543));
#39626=CARTESIAN_POINT('Ctrl Pts',(-0.15248488362145,-1.,-2.00917680318424));
#39627=CARTESIAN_POINT('Ctrl Pts',(-0.150696157673078,-1.,-2.01500291940238));
#39628=CARTESIAN_POINT('Ctrl Pts',(-0.148856124775337,-1.,-2.02083464969894));
#39629=CARTESIAN_POINT('Ctrl Pts',(-0.146965557332583,-1.,-2.02666926182017));
#39630=CARTESIAN_POINT('Ctrl Pts',(-0.145025140186057,-1.,-2.03250223739942));
#39631=CARTESIAN_POINT('Ctrl Pts',(-0.143035515058209,-1.,-2.03832911025912));
#39632=CARTESIAN_POINT('Ctrl Pts',(-0.140997332152546,-1.,-2.04414757947916));
#39633=CARTESIAN_POINT('Ctrl Pts',(-0.138911255368966,-1.,-2.04995762001328));
#39634=CARTESIAN_POINT('Ctrl Pts',(-0.136777941218044,-1.,-2.05576044414264));
#39635=CARTESIAN_POINT('Ctrl Pts',(-0.134598026192106,-1.,-2.06155781517842));
#39636=CARTESIAN_POINT('Ctrl Pts',(-0.13237211154771,-1.,-2.06735123910326));
#39637=CARTESIAN_POINT('Ctrl Pts',(-0.130100748328403,-1.,-2.07314114713063));
#39638=CARTESIAN_POINT('Ctrl Pts',(-0.12778444527612,-1.,-2.07892715110987));
#39639=CARTESIAN_POINT('Ctrl Pts',(-0.125423679412061,-1.,-2.08470840653643));
#39640=CARTESIAN_POINT('Ctrl Pts',(-0.123018905621083,-1.,-2.09048392424825));
#39641=CARTESIAN_POINT('Ctrl Pts',(-0.120570567965122,-1.,-2.0962529286773));
#39642=CARTESIAN_POINT('Ctrl Pts',(-0.118079107988355,-1.,-2.102015121329));
#39643=CARTESIAN_POINT('Ctrl Pts',(-0.115544957687926,-1.,-2.10777050261309));
#39644=CARTESIAN_POINT('Ctrl Pts',(-0.112968534419737,-1.,-2.11351924490306));
#39645=CARTESIAN_POINT('Ctrl Pts',(-0.110350236135025,-1.,-2.11926155590865));
#39646=CARTESIAN_POINT('Ctrl Pts',(-0.10769043523109,-1.,-2.12499752307));
#39647=CARTESIAN_POINT('Ctrl Pts',(-0.104989479152739,-1.,-2.13072704887293));
#39648=CARTESIAN_POINT('Ctrl Pts',(-0.1022477005561,-1.,-2.13644992667165));
#39649=CARTESIAN_POINT('Ctrl Pts',(-0.0994654261990915,-1.,-2.14216588396025));
#39650=CARTESIAN_POINT('Ctrl Pts',(-0.0966429852305459,-1.,-2.14787463531795));
#39651=CARTESIAN_POINT('Ctrl Pts',(-0.0937807218867643,-1.,-2.1535759397817));
#39652=CARTESIAN_POINT('Ctrl Pts',(-0.0908789888107265,-1.,-2.15926961544516));
#39653=CARTESIAN_POINT('Ctrl Pts',(-0.0879381291386923,-1.,-2.16495552645014));
#39654=CARTESIAN_POINT('Ctrl Pts',(-0.0849584620835372,-1.,-2.17063357870952));
#39655=CARTESIAN_POINT('Ctrl Pts',(-0.0819402680872765,-1.,-2.176303712113));
#39656=CARTESIAN_POINT('Ctrl Pts',(-0.0788837727685243,-1.,-2.18196589448887));
#39657=CARTESIAN_POINT('Ctrl Pts',(-0.0757891465836148,-1.,-2.1876201139953));
#39658=CARTESIAN_POINT('Ctrl Pts',(-0.0732830357306725,-1.,-2.19213712013662));
#39659=CARTESIAN_POINT('Ctrl Pts',(-0.0713863779526154,-1.,-2.19552129484002));
#39660=CARTESIAN_POINT('Ctrl Pts',(-0.070114353632549,-1.,-2.19777582085423));
#39661=CARTESIAN_POINT('Ctrl Pts',(-0.0694764450219581,-1.,-2.19890268624765));
#39662=CARTESIAN_POINT('',(0.0694764450219584,-1.,-2.19890268624765));
#39663=CARTESIAN_POINT('',(-0.0694764450219581,-1.,-2.19890268624765));
#39664=CARTESIAN_POINT('',(0.163289472382896,-1.,-1.74236521665491));
#39665=CARTESIAN_POINT('Ctrl Pts',(0.0694764450219584,-1.,-2.19890268624765));
#39666=CARTESIAN_POINT('Ctrl Pts',(0.0701143536324926,-1.,-2.19777582085261));
#39667=CARTESIAN_POINT('Ctrl Pts',(0.0713863779524627,-1.,-2.19552129483562));
#39668=CARTESIAN_POINT('Ctrl Pts',(0.0732830357304276,-1.,-2.19213712012956));
#39669=CARTESIAN_POINT('Ctrl Pts',(0.0757891465833411,-1.,-2.1876201139874));
#39670=CARTESIAN_POINT('Ctrl Pts',(0.0788837727683228,-1.,-2.18196589448304));
#39671=CARTESIAN_POINT('Ctrl Pts',(0.0819402680871939,-1.,-2.1763037121106));
#39672=CARTESIAN_POINT('Ctrl Pts',(0.0849584620835643,-1.,-2.17063357871031));
#39673=CARTESIAN_POINT('Ctrl Pts',(0.0879381291387823,-1.,-2.16495552645275));
#39674=CARTESIAN_POINT('Ctrl Pts',(0.0908789888108266,-1.,-2.15926961544808));
#39675=CARTESIAN_POINT('Ctrl Pts',(0.0937807218868345,-1.,-2.15357593978377));
#39676=CARTESIAN_POINT('Ctrl Pts',(0.0966429852305689,-1.,-2.14787463531864));
#39677=CARTESIAN_POINT('Ctrl Pts',(0.0994654261990743,-1.,-2.14216588395974));
#39678=CARTESIAN_POINT('Ctrl Pts',(0.102247700556064,-1.,-2.13644992667052));
#39679=CARTESIAN_POINT('Ctrl Pts',(0.104989479152703,-1.,-2.1307270488718));
#39680=CARTESIAN_POINT('Ctrl Pts',(0.107690435231068,-1.,-2.12499752306927));
#39681=CARTESIAN_POINT('Ctrl Pts',(0.11035023613502,-1.,-2.11926155590849));
#39682=CARTESIAN_POINT('Ctrl Pts',(0.112968534419746,-1.,-2.11351924490335));
#39683=CARTESIAN_POINT('Ctrl Pts',(0.11554495768794,-1.,-2.10777050261359));
#39684=CARTESIAN_POINT('Ctrl Pts',(0.118079107988368,-1.,-2.10201512132945));
#39685=CARTESIAN_POINT('Ctrl Pts',(0.120570567965129,-1.,-2.09625292867756));
#39686=CARTESIAN_POINT('Ctrl Pts',(0.123018905621083,-1.,-2.09048392424826));
#39687=CARTESIAN_POINT('Ctrl Pts',(0.125423679412058,-1.,-2.08470840653628));
#39688=CARTESIAN_POINT('Ctrl Pts',(0.127784445276116,-1.,-2.07892715110967));
#39689=CARTESIAN_POINT('Ctrl Pts',(0.1301007483284,-1.,-2.07314114713047));
#39690=CARTESIAN_POINT('Ctrl Pts',(0.13237211154771,-1.,-2.06735123910319));
#39691=CARTESIAN_POINT('Ctrl Pts',(0.134598026192107,-1.,-2.06155781517844));
#39692=CARTESIAN_POINT('Ctrl Pts',(0.136777941218044,-1.,-2.0557604441427));
#39693=CARTESIAN_POINT('Ctrl Pts',(0.138911255368966,-1.,-2.04995762001333));
#39694=CARTESIAN_POINT('Ctrl Pts',(0.140997332152545,-1.,-2.04414757947919));
#39695=CARTESIAN_POINT('Ctrl Pts',(0.143035515058208,-1.,-2.03832911025913));
#39696=CARTESIAN_POINT('Ctrl Pts',(0.145025140186058,-1.,-2.03250223739941));
#39697=CARTESIAN_POINT('Ctrl Pts',(0.146965557332586,-1.,-2.02666926182017));
#39698=CARTESIAN_POINT('Ctrl Pts',(0.148856124775343,-1.,-2.02083464969897));
#39699=CARTESIAN_POINT('Ctrl Pts',(0.150696157673084,-1.,-2.01500291940243));
#39700=CARTESIAN_POINT('Ctrl Pts',(0.152484883621452,-1.,-2.00917680318426));
#39701=CARTESIAN_POINT('Ctrl Pts',(0.154221403049719,-1.,-2.00335565310539));
#39702=CARTESIAN_POINT('Ctrl Pts',(0.155904629548774,-1.,-1.99753284771487));
#39703=CARTESIAN_POINT('Ctrl Pts',(0.157533331459215,-1.,-1.99169810931893));
#39704=CARTESIAN_POINT('Ctrl Pts',(0.159106226437288,-1.,-1.98584238283279));
#39705=CARTESIAN_POINT('Ctrl Pts',(0.16062206078461,-1.,-1.97996195437557));
#39706=CARTESIAN_POINT('Ctrl Pts',(0.162079693556302,-1.,-1.97406280235204));
#39707=CARTESIAN_POINT('Ctrl Pts',(0.16347818545776,-1.,-1.96816512678));
#39708=CARTESIAN_POINT('Ctrl Pts',(0.1648165689203,-1.,-1.96229379940174));
#39709=CARTESIAN_POINT('Ctrl Pts',(0.166093592002833,-1.,-1.95646759718755));
#39710=CARTESIAN_POINT('Ctrl Pts',(0.167307501784469,-1.,-1.95069027794286));
#39711=CARTESIAN_POINT('Ctrl Pts',(0.168455741607516,-1.,-1.94493757756879));
#39712=CARTESIAN_POINT('Ctrl Pts',(0.169534904817425,-1.,-1.93915639211497));
#39713=CARTESIAN_POINT('Ctrl Pts',(0.170541253116136,-1.,-1.93329183155455));
#39714=CARTESIAN_POINT('Ctrl Pts',(0.17147119153296,-1.,-1.92731093582));
#39715=CARTESIAN_POINT('Ctrl Pts',(0.172321621259557,-1.,-1.92122334398034));
#39716=CARTESIAN_POINT('Ctrl Pts',(0.173090695383619,-1.,-1.91511429159681));
#39717=CARTESIAN_POINT('Ctrl Pts',(0.173776635257984,-1.,-1.90911693975475));
#39718=CARTESIAN_POINT('Ctrl Pts',(0.174375518661222,-1.,-1.90335253863003));
#39719=CARTESIAN_POINT('Ctrl Pts',(0.174879405091277,-1.,-1.89788101117148));
#39720=CARTESIAN_POINT('Ctrl Pts',(0.175274276190664,-1.,-1.89264630198279));
#39721=CARTESIAN_POINT('Ctrl Pts',(0.175538155840286,-1.,-1.88742606272818));
#39722=CARTESIAN_POINT('Ctrl Pts',(0.175644148889271,-1.,-1.88188663144846));
#39723=CARTESIAN_POINT('Ctrl Pts',(0.175563480746205,-1.,-1.87563767773249));
#39724=CARTESIAN_POINT('Ctrl Pts',(0.175268337590901,-1.,-1.86828349694972));
#39725=CARTESIAN_POINT('Ctrl Pts',(0.174735259276856,-1.,-1.85948367089838));
#39726=CARTESIAN_POINT('Ctrl Pts',(0.173946627589401,-1.,-1.84898113200543));
#39727=CARTESIAN_POINT('Ctrl Pts',(0.17288944289442,-1.,-1.83658380530747));
#39728=CARTESIAN_POINT('Ctrl Pts',(0.171554770207306,-1.,-1.82215766815414));
#39729=CARTESIAN_POINT('Ctrl Pts',(0.169936923908078,-1.,-1.80561530633924));
#39730=CARTESIAN_POINT('Ctrl Pts',(0.16803277280837,-1.,-1.78690649988931));
#39731=CARTESIAN_POINT('Ctrl Pts',(0.166279355148738,-1.,-1.77018771687692));
#39732=CARTESIAN_POINT('Ctrl Pts',(0.164834765708484,-1.,-1.75666056640041));
#39733=CARTESIAN_POINT('Ctrl Pts',(0.163814161002474,-1.,-1.74720349503904));
#39734=CARTESIAN_POINT('Ctrl Pts',(0.163289472382896,-1.,-1.74236521665491));
#39735=CARTESIAN_POINT('',(0.383122945602004,-1.,-1.7075470150345));
#39736=CARTESIAN_POINT('Origin',(0.,-1.,0.));
#39737=CARTESIAN_POINT('',(0.61342227326009,-1.,-2.11275013067528));
#39738=CARTESIAN_POINT('Ctrl Pts',(0.383122945602004,-1.,-1.7075470150345));
#39739=CARTESIAN_POINT('Ctrl Pts',(0.384119047314215,-1.,-1.71231062891398));
#39740=CARTESIAN_POINT('Ctrl Pts',(0.386070790323281,-1.,-1.72162022244582));
#39741=CARTESIAN_POINT('Ctrl Pts',(0.388877023502615,-1.,-1.73493170972829));
#39742=CARTESIAN_POINT('Ctrl Pts',(0.392375812285395,-1.,-1.75137405310193));
#39743=CARTESIAN_POINT('Ctrl Pts',(0.396346196110688,-1.,-1.76975560043442));
#39744=CARTESIAN_POINT('Ctrl Pts',(0.399919403774155,-1.,-1.78598826343754));
#39745=CARTESIAN_POINT('Ctrl Pts',(0.403107976163396,-1.,-1.80012077173238));
#39746=CARTESIAN_POINT('Ctrl Pts',(0.405933518407175,-1.,-1.81223801812013));
#39747=CARTESIAN_POINT('Ctrl Pts',(0.408428948106227,-1.,-1.82247022677562));
#39748=CARTESIAN_POINT('Ctrl Pts',(0.410641256301276,-1.,-1.83100408895047));
#39749=CARTESIAN_POINT('Ctrl Pts',(0.412633125322945,-1.,-1.8380895347617));
#39750=CARTESIAN_POINT('Ctrl Pts',(0.414487438255542,-1.,-1.84405757074218));
#39751=CARTESIAN_POINT('Ctrl Pts',(0.416300022039885,-1.,-1.84929312930314));
#39752=CARTESIAN_POINT('Ctrl Pts',(0.418164129144045,-1.,-1.8541763285645));
#39753=CARTESIAN_POINT('Ctrl Pts',(0.420157287975583,-1.,-1.8590328109667));
#39754=CARTESIAN_POINT('Ctrl Pts',(0.422327307417884,-1.,-1.86408083333863));
#39755=CARTESIAN_POINT('Ctrl Pts',(0.424678177290876,-1.,-1.8693780394412));
#39756=CARTESIAN_POINT('Ctrl Pts',(0.427183828518743,-1.,-1.87486989291334));
#39757=CARTESIAN_POINT('Ctrl Pts',(0.429803062482217,-1.,-1.88044229001779));
#39758=CARTESIAN_POINT('Ctrl Pts',(0.432493038548833,-1.,-1.88596913666828));
#39759=CARTESIAN_POINT('Ctrl Pts',(0.43522566096358,-1.,-1.89136993975585));
#39760=CARTESIAN_POINT('Ctrl Pts',(0.437995003948443,-1.,-1.89663648956549));
#39761=CARTESIAN_POINT('Ctrl Pts',(0.44080783370416,-1.,-1.90180124389137));
#39762=CARTESIAN_POINT('Ctrl Pts',(0.44367755684917,-1.,-1.90691756144906));
#39763=CARTESIAN_POINT('Ctrl Pts',(0.446617343485651,-1.,-1.91203699981095));
#39764=CARTESIAN_POINT('Ctrl Pts',(0.449632260106572,-1.,-1.91718342555717));
#39765=CARTESIAN_POINT('Ctrl Pts',(0.452719478359356,-1.,-1.9223538064847));
#39766=CARTESIAN_POINT('Ctrl Pts',(0.455872005174335,-1.,-1.92753067150461));
#39767=CARTESIAN_POINT('Ctrl Pts',(0.459081234547931,-1.,-1.93269066517936));
#39768=CARTESIAN_POINT('Ctrl Pts',(0.462340031009087,-1.,-1.93781486640834));
#39769=CARTESIAN_POINT('Ctrl Pts',(0.465645462026064,-1.,-1.94289794196205));
#39770=CARTESIAN_POINT('Ctrl Pts',(0.468997482913158,-1.,-1.94794381136524));
#39771=CARTESIAN_POINT('Ctrl Pts',(0.472397672264079,-1.,-1.95296148278136));
#39772=CARTESIAN_POINT('Ctrl Pts',(0.475848034683171,-1.,-1.95796111148175));
#39773=CARTESIAN_POINT('Ctrl Pts',(0.479349583074846,-1.,-1.96294933055938));
#39774=CARTESIAN_POINT('Ctrl Pts',(0.482901662120686,-1.,-1.96792703422358));
#39775=CARTESIAN_POINT('Ctrl Pts',(0.486502692907661,-1.,-1.97289186263272));
#39776=CARTESIAN_POINT('Ctrl Pts',(0.490150627860955,-1.,-1.97783973019229));
#39777=CARTESIAN_POINT('Ctrl Pts',(0.493843476541492,-1.,-1.9827665876182));
#39778=CARTESIAN_POINT('Ctrl Pts',(0.497579909545564,-1.,-1.98767044752929));
#39779=CARTESIAN_POINT('Ctrl Pts',(0.501359287727129,-1.,-1.9925514912615));
#39780=CARTESIAN_POINT('Ctrl Pts',(0.505181361323011,-1.,-1.99741107463567));
#39781=CARTESIAN_POINT('Ctrl Pts',(0.509046069886152,-1.,-2.00225107134733));
#39782=CARTESIAN_POINT('Ctrl Pts',(0.512953306961813,-1.,-2.00707309946955));
#39783=CARTESIAN_POINT('Ctrl Pts',(0.516902681728733,-1.,-2.01187773939257));
#39784=CARTESIAN_POINT('Ctrl Pts',(0.520893590399428,-1.,-2.01666477917306));
#39785=CARTESIAN_POINT('Ctrl Pts',(0.524925318333518,-1.,-2.02143356304712));
#39786=CARTESIAN_POINT('Ctrl Pts',(0.52899712724191,-1.,-2.02618329083289));
#39787=CARTESIAN_POINT('Ctrl Pts',(0.533108355132905,-1.,-2.03091336214401));
#39788=CARTESIAN_POINT('Ctrl Pts',(0.537258489833134,-1.,-2.03562362953993));
#39789=CARTESIAN_POINT('Ctrl Pts',(0.54144712061552,-1.,-2.0403142269048));
#39790=CARTESIAN_POINT('Ctrl Pts',(0.545673903817348,-1.,-2.0449854471456));
#39791=CARTESIAN_POINT('Ctrl Pts',(0.549938525150342,-1.,-2.04963761077974));
#39792=CARTESIAN_POINT('Ctrl Pts',(0.554240657464109,-1.,-2.05427091604482));
#39793=CARTESIAN_POINT('Ctrl Pts',(0.558579940185467,-1.,-2.05888537756571));
#39794=CARTESIAN_POINT('Ctrl Pts',(0.562955993082574,-1.,-2.06348090160697));
#39795=CARTESIAN_POINT('Ctrl Pts',(0.567368421181229,-1.,-2.06805732997383));
#39796=CARTESIAN_POINT('Ctrl Pts',(0.571816823242411,-1.,-2.07261449292758));
#39797=CARTESIAN_POINT('Ctrl Pts',(0.576300797416274,-1.,-2.07715226767361));
#39798=CARTESIAN_POINT('Ctrl Pts',(0.580819952107256,-1.,-2.08167059018138));
#39799=CARTESIAN_POINT('Ctrl Pts',(0.585373918990895,-1.,-2.086169437277));
#39800=CARTESIAN_POINT('Ctrl Pts',(0.589962365403189,-1.,-2.09064881812053));
#39801=CARTESIAN_POINT('Ctrl Pts',(0.594585006052823,-1.,-2.09510876220501));
#39802=CARTESIAN_POINT('Ctrl Pts',(0.599241616422144,-1.,-2.09954930865331));
#39803=CARTESIAN_POINT('Ctrl Pts',(0.603932030738212,-1.,-2.10397049887709));
#39804=CARTESIAN_POINT('Ctrl Pts',(0.607711315456826,-1.,-2.10749199615859));
#39805=CARTESIAN_POINT('Ctrl Pts',(0.610560911691113,-1.,-2.11012443807661));
#39806=CARTESIAN_POINT('Ctrl Pts',(0.61246736556225,-1.,-2.11187554260142));
#39807=CARTESIAN_POINT('Ctrl Pts',(0.61342227326009,-1.,-2.11275013067528));
#39808=CARTESIAN_POINT('',(0.745574324794401,-1.,-2.0698113262342));
#39809=CARTESIAN_POINT('',(0.61342227326009,-1.,-2.11275013067528));
#39810=CARTESIAN_POINT('',(0.693717979106306,-1.,-1.60662857109684));
#39811=CARTESIAN_POINT('Ctrl Pts',(0.745574324794401,-1.,-2.0698113262342));
#39812=CARTESIAN_POINT('Ctrl Pts',(0.74583279137781,-1.,-2.06854248895575));
#39813=CARTESIAN_POINT('Ctrl Pts',(0.746345871542695,-1.,-2.06600523016401));
#39814=CARTESIAN_POINT('Ctrl Pts',(0.747103932785504,-1.,-2.06220058927162));
#39815=CARTESIAN_POINT('Ctrl Pts',(0.748091554181101,-1.,-2.05713023030263));
#39816=CARTESIAN_POINT('Ctrl Pts',(0.749287468663053,-1.,-2.05079645591606));
#39817=CARTESIAN_POINT('Ctrl Pts',(0.750444657874758,-1.,-2.04446689147754));
#39818=CARTESIAN_POINT('Ctrl Pts',(0.751562963361383,-1.,-2.03814160092173));
#39819=CARTESIAN_POINT('Ctrl Pts',(0.752642180488104,-1.,-2.03182068456467));
#39820=CARTESIAN_POINT('Ctrl Pts',(0.753682061113765,-1.,-2.02550428623587));
#39821=CARTESIAN_POINT('Ctrl Pts',(0.75468233072352,-1.,-2.01919259406003));
#39822=CARTESIAN_POINT('Ctrl Pts',(0.7556427049581,-1.,-2.01288584328149));
#39823=CARTESIAN_POINT('Ctrl Pts',(0.756562904646496,-1.,-2.00658431587682));
#39824=CARTESIAN_POINT('Ctrl Pts',(0.757442676862341,-1.,-2.00028834739072));
#39825=CARTESIAN_POINT('Ctrl Pts',(0.758281796766377,-1.,-1.9939983109871));
#39826=CARTESIAN_POINT('Ctrl Pts',(0.759080037802242,-1.,-1.98771456680806));
#39827=CARTESIAN_POINT('Ctrl Pts',(0.759837147452135,-1.,-1.98143741418156));
#39828=CARTESIAN_POINT('Ctrl Pts',(0.760552825409855,-1.,-1.97516705321521));
#39829=CARTESIAN_POINT('Ctrl Pts',(0.761226690483986,-1.,-1.96890351582545));
#39830=CARTESIAN_POINT('Ctrl Pts',(0.761858300014575,-1.,-1.96264672744229));
#39831=CARTESIAN_POINT('Ctrl Pts',(0.762447203806263,-1.,-1.95639665309893));
#39832=CARTESIAN_POINT('Ctrl Pts',(0.762992990878774,-1.,-1.95015342590025));
#39833=CARTESIAN_POINT('Ctrl Pts',(0.76349533353858,-1.,-1.94391746617626));
#39834=CARTESIAN_POINT('Ctrl Pts',(0.763954049121393,-1.,-1.93768964875867));
#39835=CARTESIAN_POINT('Ctrl Pts',(0.764369010673889,-1.,-1.93147105496367));
#39836=CARTESIAN_POINT('Ctrl Pts',(0.764740025488189,-1.,-1.92526263537041));
#39837=CARTESIAN_POINT('Ctrl Pts',(0.765066729667095,-1.,-1.91906491634197));
#39838=CARTESIAN_POINT('Ctrl Pts',(0.765348465884739,-1.,-1.91287765805174));
#39839=CARTESIAN_POINT('Ctrl Pts',(0.765584196937936,-1.,-1.90669961402362));
#39840=CARTESIAN_POINT('Ctrl Pts',(0.765772772593395,-1.,-1.90052930393599));
#39841=CARTESIAN_POINT('Ctrl Pts',(0.765913193856979,-1.,-1.89436577771389));
#39842=CARTESIAN_POINT('Ctrl Pts',(0.76600483706209,-1.,-1.88820926433409));
#39843=CARTESIAN_POINT('Ctrl Pts',(0.766047794851868,-1.,-1.88206215302561));
#39844=CARTESIAN_POINT('Ctrl Pts',(0.766042837036759,-1.,-1.87592888967886));
#39845=CARTESIAN_POINT('Ctrl Pts',(0.765990708546111,-1.,-1.86981398314345));
#39846=CARTESIAN_POINT('Ctrl Pts',(0.765891519092557,-1.,-1.86372027063315));
#39847=CARTESIAN_POINT('Ctrl Pts',(0.765744212909305,-1.,-1.85764741390391));
#39848=CARTESIAN_POINT('Ctrl Pts',(0.765545710619023,-1.,-1.85158945130054));
#39849=CARTESIAN_POINT('Ctrl Pts',(0.765291664861971,-1.,-1.84553698875911));
#39850=CARTESIAN_POINT('Ctrl Pts',(0.764978057881687,-1.,-1.83948181064823));
#39851=CARTESIAN_POINT('Ctrl Pts',(0.764602549687845,-1.,-1.8334207722714));
#39852=CARTESIAN_POINT('Ctrl Pts',(0.764165902606055,-1.,-1.8273599120008));
#39853=CARTESIAN_POINT('Ctrl Pts',(0.763673465462854,-1.,-1.82131873145297));
#39854=CARTESIAN_POINT('Ctrl Pts',(0.763132003836783,-1.,-1.81532118405566));
#39855=CARTESIAN_POINT('Ctrl Pts',(0.762546129464036,-1.,-1.80938551463989));
#39856=CARTESIAN_POINT('Ctrl Pts',(0.761915336443515,-1.,-1.80351583877334));
#39857=CARTESIAN_POINT('Ctrl Pts',(0.761229695230359,-1.,-1.79768986997735));
#39858=CARTESIAN_POINT('Ctrl Pts',(0.760469555880425,-1.,-1.79185815610802));
#39859=CARTESIAN_POINT('Ctrl Pts',(0.759614401109868,-1.,-1.78596964884527));
#39860=CARTESIAN_POINT('Ctrl Pts',(0.75865062667738,-1.,-1.77999411220912));
#39861=CARTESIAN_POINT('Ctrl Pts',(0.757578264077238,-1.,-1.77394167108342));
#39862=CARTESIAN_POINT('Ctrl Pts',(0.756421896028403,-1.,-1.76789396003141));
#39863=CARTESIAN_POINT('Ctrl Pts',(0.755220979975262,-1.,-1.7619781724032));
#39864=CARTESIAN_POINT('Ctrl Pts',(0.75400925402848,-1.,-1.75631083600175));
#39865=CARTESIAN_POINT('Ctrl Pts',(0.752797683531377,-1.,-1.75095139468809));
#39866=CARTESIAN_POINT('Ctrl Pts',(0.751555614163629,-1.,-1.74585086852298));
#39867=CARTESIAN_POINT('Ctrl Pts',(0.75019343597954,-1.,-1.74080458266705));
#39868=CARTESIAN_POINT('Ctrl Pts',(0.748582462954854,-1.,-1.73550351679848));
#39869=CARTESIAN_POINT('Ctrl Pts',(0.746574710096436,-1.,-1.72958533647399));
#39870=CARTESIAN_POINT('Ctrl Pts',(0.744021445433764,-1.,-1.7226822991693));
#39871=CARTESIAN_POINT('Ctrl Pts',(0.740795162032087,-1.,-1.71447789751927));
#39872=CARTESIAN_POINT('Ctrl Pts',(0.736799665724771,-1.,-1.70473309006121));
#39873=CARTESIAN_POINT('Ctrl Pts',(0.731963238697195,-1.,-1.69326921975743));
#39874=CARTESIAN_POINT('Ctrl Pts',(0.726235967997433,-1.,-1.67996158455503));
#39875=CARTESIAN_POINT('Ctrl Pts',(0.719585433804282,-1.,-1.6647288055568));
#39876=CARTESIAN_POINT('Ctrl Pts',(0.711993139355394,-1.,-1.64752408832016));
#39877=CARTESIAN_POINT('Ctrl Pts',(0.705159151988319,-1.,-1.63216541664676));
#39878=CARTESIAN_POINT('Ctrl Pts',(0.699605146405088,-1.,-1.61974673472612));
#39879=CARTESIAN_POINT('Ctrl Pts',(0.695712097881194,-1.,-1.61106790958151));
#39880=CARTESIAN_POINT('Ctrl Pts',(0.693717979106306,-1.,-1.60662857109684));
#39881=CARTESIAN_POINT('',(0.892032620296855,-1.,-1.5055822144029));
#39882=CARTESIAN_POINT('Origin',(0.,-1.,0.));
#39883=CARTESIAN_POINT('',(1.23627494547115,-1.,-1.81978687191668));
#39884=CARTESIAN_POINT('Ctrl Pts',(0.892032620296855,-1.,-1.5055822144029));
#39885=CARTESIAN_POINT('Ctrl Pts',(0.894452006964543,-1.,-1.50980486806688));
#39886=CARTESIAN_POINT('Ctrl Pts',(0.89918504748351,-1.,-1.51805569590094));
#39887=CARTESIAN_POINT('Ctrl Pts',(0.905967409625651,-1.,-1.52984849887993));
#39888=CARTESIAN_POINT('Ctrl Pts',(0.914375919026456,-1.,-1.54440491149498));
#39889=CARTESIAN_POINT('Ctrl Pts',(0.923832188944341,-1.,-1.56065988578893));
#39890=CARTESIAN_POINT('Ctrl Pts',(0.932246680108685,-1.,-1.57499388382243));
#39891=CARTESIAN_POINT('Ctrl Pts',(0.939646377893399,-1.,-1.58744937487176));
#39892=CARTESIAN_POINT('Ctrl Pts',(0.946078063315257,-1.,-1.59810042043673));
#39893=CARTESIAN_POINT('Ctrl Pts',(0.951613284356035,-1.,-1.60706069896936));
#39894=CARTESIAN_POINT('Ctrl Pts',(0.95635442292067,-1.,-1.61449324337085));
#39895=CARTESIAN_POINT('Ctrl Pts',(0.960438326101728,-1.,-1.62061638140221));
#39896=CARTESIAN_POINT('Ctrl Pts',(0.964046107040535,-1.,-1.62571930670187));
#39897=CARTESIAN_POINT('Ctrl Pts',(0.967387853230345,-1.,-1.63013849959462));
#39898=CARTESIAN_POINT('Ctrl Pts',(0.970669715997509,-1.,-1.63420665729798));
#39899=CARTESIAN_POINT('Ctrl Pts',(0.974066058287418,-1.,-1.63820952658144));
#39900=CARTESIAN_POINT('Ctrl Pts',(0.977689794119416,-1.,-1.64233990826687));
#39901=CARTESIAN_POINT('Ctrl Pts',(0.981562530939489,-1.,-1.64665139190656));
#39902=CARTESIAN_POINT('Ctrl Pts',(0.98564262292082,-1.,-1.65110016612638));
#39903=CARTESIAN_POINT('Ctrl Pts',(0.989855627854164,-1.,-1.65559044289699));
#39904=CARTESIAN_POINT('Ctrl Pts',(0.994121836661305,-1.,-1.66001553809947));
#39905=CARTESIAN_POINT('Ctrl Pts',(0.998389654952757,-1.,-1.66430758030376));
#39906=CARTESIAN_POINT('Ctrl Pts',(1.00265091003727,-1.,-1.66846059277303));
#39907=CARTESIAN_POINT('Ctrl Pts',(1.00692206696414,-1.,-1.67250335383293));
#39908=CARTESIAN_POINT('Ctrl Pts',(1.01123236493511,-1.,-1.67648246776464));
#39909=CARTESIAN_POINT('Ctrl Pts',(1.01561026162773,-1.,-1.68044289894798));
#39910=CARTESIAN_POINT('Ctrl Pts',(1.02006795074201,-1.,-1.68440578021706));
#39911=CARTESIAN_POINT('Ctrl Pts',(1.02460180535255,-1.,-1.68836910178447));
#39912=CARTESIAN_POINT('Ctrl Pts',(1.02919977579147,-1.,-1.69231840863458));
#39913=CARTESIAN_POINT('Ctrl Pts',(1.03384646003588,-1.,-1.69623414782771));
#39914=CARTESIAN_POINT('Ctrl Pts',(1.03852922490789,-1.,-1.70010052930962));
#39915=CARTESIAN_POINT('Ctrl Pts',(1.04324363334554,-1.,-1.70391338707982));
#39916=CARTESIAN_POINT('Ctrl Pts',(1.04799085404995,-1.,-1.70767646263649));
#39917=CARTESIAN_POINT('Ctrl Pts',(1.05277517202855,-1.,-1.71139783543989));
#39918=CARTESIAN_POINT('Ctrl Pts',(1.05760163192479,-1.,-1.7150865442702));
#39919=CARTESIAN_POINT('Ctrl Pts',(1.06247324680647,-1.,-1.71874858456904));
#39920=CARTESIAN_POINT('Ctrl Pts',(1.06738966975462,-1.,-1.72238500928453));
#39921=CARTESIAN_POINT('Ctrl Pts',(1.07234866990252,-1.,-1.72599406198488));
#39922=CARTESIAN_POINT('Ctrl Pts',(1.0773470373727,-1.,-1.72957248977424));
#39923=CARTESIAN_POINT('Ctrl Pts',(1.08238162784749,-1.,-1.73311705663407));
#39924=CARTESIAN_POINT('Ctrl Pts',(1.08745056285427,-1.,-1.73662628326091));
#39925=CARTESIAN_POINT('Ctrl Pts',(1.09255329056493,-1.,-1.74010053962247));
#39926=CARTESIAN_POINT('Ctrl Pts',(1.09768999241225,-1.,-1.74354119236208));
#39927=CARTESIAN_POINT('Ctrl Pts',(1.10286118991143,-1.,-1.74695004214923));
#39928=CARTESIAN_POINT('Ctrl Pts',(1.10806728183007,-1.,-1.7503286607592));
#39929=CARTESIAN_POINT('Ctrl Pts',(1.11330807582551,-1.,-1.7536777209463));
#39930=CARTESIAN_POINT('Ctrl Pts',(1.11858293216763,-1.,-1.75699720772105));
#39931=CARTESIAN_POINT('Ctrl Pts',(1.12389096855086,-1.,-1.76028671825096));
#39932=CARTESIAN_POINT('Ctrl Pts',(1.12923123555075,-1.,-1.7635457196617));
#39933=CARTESIAN_POINT('Ctrl Pts',(1.1346029180462,-1.,-1.76677384551862));
#39934=CARTESIAN_POINT('Ctrl Pts',(1.14000548336975,-1.,-1.76997111386769));
#39935=CARTESIAN_POINT('Ctrl Pts',(1.1454385822692,-1.,-1.77313777896194));
#39936=CARTESIAN_POINT('Ctrl Pts',(1.15090197841514,-1.,-1.7762742255701));
#39937=CARTESIAN_POINT('Ctrl Pts',(1.15639547194698,-1.,-1.77938085564275));
#39938=CARTESIAN_POINT('Ctrl Pts',(1.16191881298499,-1.,-1.78245795881009));
#39939=CARTESIAN_POINT('Ctrl Pts',(1.16747166312303,-1.,-1.78550566040443));
#39940=CARTESIAN_POINT('Ctrl Pts',(1.17305363177328,-1.,-1.78852398877617));
#39941=CARTESIAN_POINT('Ctrl Pts',(1.17866429440809,-1.,-1.79151291552689));
#39942=CARTESIAN_POINT('Ctrl Pts',(1.18430321697432,-1.,-1.79447240321515));
#39943=CARTESIAN_POINT('Ctrl Pts',(1.18996997934445,-1.,-1.79740245923478));
#39944=CARTESIAN_POINT('Ctrl Pts',(1.19566418930242,-1.,-1.80030314369879));
#39945=CARTESIAN_POINT('Ctrl Pts',(1.20138548938974,-1.,-1.80317454838603));
#39946=CARTESIAN_POINT('Ctrl Pts',(1.20713356605475,-1.,-1.80601678480707));
#39947=CARTESIAN_POINT('Ctrl Pts',(1.21290815708314,-1.,-1.80882996917129));
#39948=CARTESIAN_POINT('Ctrl Pts',(1.21870906103557,-1.,-1.81161420806656));
#39949=CARTESIAN_POINT('Ctrl Pts',(1.2245361330495,-1.,-1.81436959210434));
#39950=CARTESIAN_POINT('Ctrl Pts',(1.2292186489137,-1.,-1.8165508718364));
#39951=CARTESIAN_POINT('Ctrl Pts',(1.2327422452705,-1.,-1.81817389921279));
#39952=CARTESIAN_POINT('Ctrl Pts',(1.23509651170476,-1.,-1.81925017193666));
#39953=CARTESIAN_POINT('Ctrl Pts',(1.23627494547115,-1.,-1.81978687191668));
#39954=CARTESIAN_POINT('',(1.34869019493419,-1.,-1.73811241238545));
#39955=CARTESIAN_POINT('',(1.23627494547115,-1.,-1.81978687191668));
#39956=CARTESIAN_POINT('',(1.15624053661742,-1.,-1.31362392696032));
#39957=CARTESIAN_POINT('Ctrl Pts',(1.34869019493419,-1.,-1.73811241238545));
#39958=CARTESIAN_POINT('Ctrl Pts',(1.34854391898045,-1.,-1.73682580585691));
#39959=CARTESIAN_POINT('Ctrl Pts',(1.34824783112887,-1.,-1.73425417885907));
#39960=CARTESIAN_POINT('Ctrl Pts',(1.34779309152035,-1.,-1.7304014965394));
#39961=CARTESIAN_POINT('Ctrl Pts',(1.34716554819527,-1.,-1.72527410680674));
#39962=CARTESIAN_POINT('Ctrl Pts',(1.34634568653227,-1.,-1.7188807715049));
#39963=CARTESIAN_POINT('Ctrl Pts',(1.34549029589416,-1.,-1.71250340686822));
#39964=CARTESIAN_POINT('Ctrl Pts',(1.34459924533831,-1.,-1.70614212266738));
#39965=CARTESIAN_POINT('Ctrl Pts',(1.34367237124483,-1.,-1.69979707754427));
#39966=CARTESIAN_POINT('Ctrl Pts',(1.34270948206319,-1.,-1.6934684849687));
#39967=CARTESIAN_POINT('Ctrl Pts',(1.341710374848,-1.,-1.68715660868764));
#39968=CARTESIAN_POINT('Ctrl Pts',(1.34067485185203,-1.,-1.68086176030362));
#39969=CARTESIAN_POINT('Ctrl Pts',(1.3396027347034,-1.,-1.67458429426086));
#39970=CARTESIAN_POINT('Ctrl Pts',(1.33849388654388,-1.,-1.66832460783989));
#39971=CARTESIAN_POINT('Ctrl Pts',(1.33734820885262,-1.,-1.66208312541983));
#39972=CARTESIAN_POINT('Ctrl Pts',(1.33616559745172,-1.,-1.65586025952593));
#39973=CARTESIAN_POINT('Ctrl Pts',(1.33494590467993,-1.,-1.6496563728683));
#39974=CARTESIAN_POINT('Ctrl Pts',(1.33368890676572,-1.,-1.6434717485603));
#39975=CARTESIAN_POINT('Ctrl Pts',(1.33239425103724,-1.,-1.63730653475089));
#39976=CARTESIAN_POINT('Ctrl Pts',(1.33106149345645,-1.,-1.63116079730923));
#39977=CARTESIAN_POINT('Ctrl Pts',(1.3296901950568,-1.,-1.62503464209797));
#39978=CARTESIAN_POINT('Ctrl Pts',(1.32828000610449,-1.,-1.61892832270724));
#39979=CARTESIAN_POINT('Ctrl Pts',(1.32683074483356,-1.,-1.6128423401575));
#39980=CARTESIAN_POINT('Ctrl Pts',(1.32534250785782,-1.,-1.60677758290954));
#39981=CARTESIAN_POINT('Ctrl Pts',(1.32381550858256,-1.,-1.60073511858687));
#39982=CARTESIAN_POINT('Ctrl Pts',(1.32224985747682,-1.,-1.59471591079403));
#39983=CARTESIAN_POINT('Ctrl Pts',(1.32064537110892,-1.,-1.58872057258245));
#39984=CARTESIAN_POINT('Ctrl Pts',(1.31900135021432,-1.,-1.58274907898834));
#39985=CARTESIAN_POINT('Ctrl Pts',(1.31731642317187,-1.,-1.5768005650559));
#39986=CARTESIAN_POINT('Ctrl Pts',(1.31558903860016,-1.,-1.57087397835723));
#39987=CARTESIAN_POINT('Ctrl Pts',(1.31381795281002,-1.,-1.56496872402353));
#39988=CARTESIAN_POINT('Ctrl Pts',(1.31200264341696,-1.,-1.55908521254821));
#39989=CARTESIAN_POINT('Ctrl Pts',(1.31014393684222,-1.,-1.55322568759481));
#39990=CARTESIAN_POINT('Ctrl Pts',(1.30824393907473,-1.,-1.54739413957185));
#39991=CARTESIAN_POINT('Ctrl Pts',(1.30630475189556,-1.,-1.54159462645432));
#39992=CARTESIAN_POINT('Ctrl Pts',(1.30432735639489,-1.,-1.53582981268977));
#39993=CARTESIAN_POINT('Ctrl Pts',(1.30231064395568,-1.,-1.53009970283891));
#39994=CARTESIAN_POINT('Ctrl Pts',(1.30024984366328,-1.,-1.52439957861062));
#39995=CARTESIAN_POINT('Ctrl Pts',(1.29813791800747,-1.,-1.51872184912724));
#39996=CARTESIAN_POINT('Ctrl Pts',(1.29596850710509,-1.,-1.51305994241402));
#39997=CARTESIAN_POINT('Ctrl Pts',(1.29373841372842,-1.,-1.50741159078365));
#39998=CARTESIAN_POINT('Ctrl Pts',(1.29145022885181,-1.,-1.50178230149776));
#39999=CARTESIAN_POINT('Ctrl Pts',(1.28911506584254,-1.,-1.49618896881754));
#40000=CARTESIAN_POINT('Ctrl Pts',(1.2867467611644,-1.,-1.4906522831278));
#40001=CARTESIAN_POINT('Ctrl Pts',(1.28435533880201,-1.,-1.4851881711891));
#40002=CARTESIAN_POINT('Ctrl Pts',(1.28194158939517,-1.,-1.47980070347096));
#40003=CARTESIAN_POINT('Ctrl Pts',(1.2794891824849,-1.,-1.4744717526707));
#40004=CARTESIAN_POINT('Ctrl Pts',(1.27696414831089,-1.,-1.46916035917133));
#40005=CARTESIAN_POINT('Ctrl Pts',(1.27433119897822,-1.,-1.46382431332476));
#40006=CARTESIAN_POINT('Ctrl Pts',(1.27156805265289,-1.,-1.45843906294697));
#40007=CARTESIAN_POINT('Ctrl Pts',(1.2686778680489,-1.,-1.45301422764247));
#40008=CARTESIAN_POINT('Ctrl Pts',(1.26570925118868,-1.,-1.44761985001662));
#40009=CARTESIAN_POINT('Ctrl Pts',(1.26273903323858,-1.,-1.44236470511303));
#40010=CARTESIAN_POINT('Ctrl Pts',(1.25983531012005,-1.,-1.43734919180848));
#40011=CARTESIAN_POINT('Ctrl Pts',(1.25702687965755,-1.,-1.43262645609691));
#40012=CARTESIAN_POINT('Ctrl Pts',(1.25426945222639,-1.,-1.42815938799387));
#40013=CARTESIAN_POINT('Ctrl Pts',(1.2514145557001,-1.,-1.42378102115575));
#40014=CARTESIAN_POINT('Ctrl Pts',(1.24824430986571,-1.,-1.41923722596025));
#40015=CARTESIAN_POINT('Ctrl Pts',(1.24450600513056,-1.,-1.41422913175179));
#40016=CARTESIAN_POINT('Ctrl Pts',(1.23994455029534,-1.,-1.40845295531283));
#40017=CARTESIAN_POINT('Ctrl Pts',(1.23434087290423,-1.,-1.40164708206106));
#40018=CARTESIAN_POINT('Ctrl Pts',(1.22752961899387,-1.,-1.39361389568796));
#40019=CARTESIAN_POINT('Ctrl Pts',(1.21938737280852,-1.,-1.38420564527715));
#40020=CARTESIAN_POINT('Ctrl Pts',(1.20982812925645,-1.,-1.37331915607905));
#40021=CARTESIAN_POINT('Ctrl Pts',(1.1987959077932,-1.,-1.36088705043885));
#40022=CARTESIAN_POINT('Ctrl Pts',(1.18625865667441,-1.,-1.34687054001093));
#40023=CARTESIAN_POINT('Ctrl Pts',(1.17501305789857,-1.,-1.33437539347008));
#40024=CARTESIAN_POINT('Ctrl Pts',(1.16589330093588,-1.,-1.32428080721772));
#40025=CARTESIAN_POINT('Ctrl Pts',(1.15950888730809,-1.,-1.31722977216397));
#40026=CARTESIAN_POINT('Ctrl Pts',(1.15624053661742,-1.,-1.31362392696032));
#40027=CARTESIAN_POINT('',(1.31362392696032,-1.,-1.15624053661742));
#40028=CARTESIAN_POINT('Origin',(0.,-1.,0.));
#40029=CARTESIAN_POINT('',(1.73811241238545,-1.,-1.34869019493419));
#40030=CARTESIAN_POINT('Ctrl Pts',(1.31362392696032,-1.,-1.15624053661742));
#40031=CARTESIAN_POINT('Ctrl Pts',(1.3172297721596,-1.,-1.15950888730433));
#40032=CARTESIAN_POINT('Ctrl Pts',(1.32428080720544,-1.,-1.16589330092532));
#40033=CARTESIAN_POINT('Ctrl Pts',(1.33437539344842,-1.,-1.17501305787994));
#40034=CARTESIAN_POINT('Ctrl Pts',(1.34687053998157,-1.,-1.18625865664915));
#40035=CARTESIAN_POINT('Ctrl Pts',(1.36088705040677,-1.,-1.1987959077656));
#40036=CARTESIAN_POINT('Ctrl Pts',(1.37331915604962,-1.,-1.20982812923113));
#40037=CARTESIAN_POINT('Ctrl Pts',(1.38420564525391,-1.,-1.21938737278853));
#40038=CARTESIAN_POINT('Ctrl Pts',(1.39361389567257,-1.,-1.22752961898063));
#40039=CARTESIAN_POINT('Ctrl Pts',(1.40164708205345,-1.,-1.23434087289768));
#40040=CARTESIAN_POINT('Ctrl Pts',(1.40845295531151,-1.,-1.23994455029421));
#40041=CARTESIAN_POINT('Ctrl Pts',(1.41422913175437,-1.,-1.24450600513278));
#40042=CARTESIAN_POINT('Ctrl Pts',(1.41923722596421,-1.,-1.24824430986911));
#40043=CARTESIAN_POINT('Ctrl Pts',(1.42378102115911,-1.,-1.25141455570299));
#40044=CARTESIAN_POINT('Ctrl Pts',(1.42815938799555,-1.,-1.25426945222783));
#40045=CARTESIAN_POINT('Ctrl Pts',(1.43262645609679,-1.,-1.25702687965744));
#40046=CARTESIAN_POINT('Ctrl Pts',(1.43734919180719,-1.,-1.25983531011894));
#40047=CARTESIAN_POINT('Ctrl Pts',(1.44236470511145,-1.,-1.26273903323723));
#40048=CARTESIAN_POINT('Ctrl Pts',(1.44761985001544,-1.,-1.26570925118767));
#40049=CARTESIAN_POINT('Ctrl Pts',(1.45301422764205,-1.,-1.26867786804854));
#40050=CARTESIAN_POINT('Ctrl Pts',(1.45843906294725,-1.,-1.27156805265312));
#40051=CARTESIAN_POINT('Ctrl Pts',(1.4638243133254,-1.,-1.27433119897877));
#40052=CARTESIAN_POINT('Ctrl Pts',(1.46916035917197,-1.,-1.27696414831144));
#40053=CARTESIAN_POINT('Ctrl Pts',(1.4744717526711,-1.,-1.27948918248524));
#40054=CARTESIAN_POINT('Ctrl Pts',(1.47980070347102,-1.,-1.28194158939522));
#40055=CARTESIAN_POINT('Ctrl Pts',(1.48518817118891,-1.,-1.28435533880184));
#40056=CARTESIAN_POINT('Ctrl Pts',(1.4906522831275,-1.,-1.28674676116415));
#40057=CARTESIAN_POINT('Ctrl Pts',(1.49618896881729,-1.,-1.28911506584232));
#40058=CARTESIAN_POINT('Ctrl Pts',(1.50178230149764,-1.,-1.29145022885171));
#40059=CARTESIAN_POINT('Ctrl Pts',(1.50741159078367,-1.,-1.29373841372843));
#40060=CARTESIAN_POINT('Ctrl Pts',(1.51305994241412,-1.,-1.29596850710518));
#40061=CARTESIAN_POINT('Ctrl Pts',(1.51872184912735,-1.,-1.29813791800757));
#40062=CARTESIAN_POINT('Ctrl Pts',(1.5243995786107,-1.,-1.30024984366334));
#40063=CARTESIAN_POINT('Ctrl Pts',(1.53009970283893,-1.,-1.3023106439557));
#40064=CARTESIAN_POINT('Ctrl Pts',(1.53582981268976,-1.,-1.30432735639487));
#40065=CARTESIAN_POINT('Ctrl Pts',(1.54159462645428,-1.,-1.30630475189553));
#40066=CARTESIAN_POINT('Ctrl Pts',(1.54739413957183,-1.,-1.30824393907471));
#40067=CARTESIAN_POINT('Ctrl Pts',(1.55322568759481,-1.,-1.31014393684221));
#40068=CARTESIAN_POINT('Ctrl Pts',(1.55908521254822,-1.,-1.31200264341696));
#40069=CARTESIAN_POINT('Ctrl Pts',(1.56496872402352,-1.,-1.31381795281002));
#40070=CARTESIAN_POINT('Ctrl Pts',(1.57087397835721,-1.,-1.31558903860015));
#40071=CARTESIAN_POINT('Ctrl Pts',(1.57680056505585,-1.,-1.31731642317183));
#40072=CARTESIAN_POINT('Ctrl Pts',(1.58274907898829,-1.,-1.31900135021428));
#40073=CARTESIAN_POINT('Ctrl Pts',(1.58872057258244,-1.,-1.32064537110891));
#40074=CARTESIAN_POINT('Ctrl Pts',(1.59471591079408,-1.,-1.32224985747686));
#40075=CARTESIAN_POINT('Ctrl Pts',(1.600735118587,-1.,-1.32381550858266));
#40076=CARTESIAN_POINT('Ctrl Pts',(1.6067775829097,-1.,-1.32534250785794));
#40077=CARTESIAN_POINT('Ctrl Pts',(1.61284234015762,-1.,-1.32683074483365));
#40078=CARTESIAN_POINT('Ctrl Pts',(1.61892832270723,-1.,-1.32828000610448));
#40079=CARTESIAN_POINT('Ctrl Pts',(1.62503464209777,-1.,-1.32969019505665));
#40080=CARTESIAN_POINT('Ctrl Pts',(1.63116079730887,-1.,-1.33106149345618));
#40081=CARTESIAN_POINT('Ctrl Pts',(1.63730653475049,-1.,-1.33239425103694));
#40082=CARTESIAN_POINT('Ctrl Pts',(1.64347174856007,-1.,-1.33368890676554));
#40083=CARTESIAN_POINT('Ctrl Pts',(1.64965637286843,-1.,-1.33494590468003));
#40084=CARTESIAN_POINT('Ctrl Pts',(1.65586025952651,-1.,-1.33616559745217));
#40085=CARTESIAN_POINT('Ctrl Pts',(1.66208312542073,-1.,-1.33734820885331));
#40086=CARTESIAN_POINT('Ctrl Pts',(1.66832460784078,-1.,-1.33849388654458));
#40087=CARTESIAN_POINT('Ctrl Pts',(1.67458429426126,-1.,-1.33960273470372));
#40088=CARTESIAN_POINT('Ctrl Pts',(1.68086176030308,-1.,-1.3406748518516));
#40089=CARTESIAN_POINT('Ctrl Pts',(1.68715660868602,-1.,-1.34171037484673));
#40090=CARTESIAN_POINT('Ctrl Pts',(1.6934684849664,-1.,-1.34270948206139));
#40091=CARTESIAN_POINT('Ctrl Pts',(1.69979707754221,-1.,-1.34367237124322));
#40092=CARTESIAN_POINT('Ctrl Pts',(1.70614212266676,-1.,-1.34459924533783));
#40093=CARTESIAN_POINT('Ctrl Pts',(1.71250340687011,-1.,-1.34549029589563));
#40094=CARTESIAN_POINT('Ctrl Pts',(1.7188807715095,-1.,-1.34634568653586));
#40095=CARTESIAN_POINT('Ctrl Pts',(1.72527410681298,-1.,-1.34716554820013));
#40096=CARTESIAN_POINT('Ctrl Pts',(1.73040149654497,-1.,-1.3477930915247));
#40097=CARTESIAN_POINT('Ctrl Pts',(1.73425417886254,-1.,-1.34824783113158));
#40098=CARTESIAN_POINT('Ctrl Pts',(1.73682580585819,-1.,-1.34854391898145));
#40099=CARTESIAN_POINT('Ctrl Pts',(1.73811241238545,-1.,-1.34869019493419));
#40100=CARTESIAN_POINT('',(1.81978687191668,-1.,-1.23627494547115));
#40101=CARTESIAN_POINT('',(1.73811241238545,-1.,-1.34869019493419));
#40102=CARTESIAN_POINT('',(1.5055822144029,-1.,-0.892032620296855));
#40103=CARTESIAN_POINT('Ctrl Pts',(1.81978687191668,-1.,-1.23627494547115));
#40104=CARTESIAN_POINT('Ctrl Pts',(1.81925017193531,-1.,-1.23509651170384));
#40105=CARTESIAN_POINT('Ctrl Pts',(1.81817389920914,-1.,-1.23274224526804));
#40106=CARTESIAN_POINT('Ctrl Pts',(1.81655087183054,-1.,-1.22921864890975));
#40107=CARTESIAN_POINT('Ctrl Pts',(1.81436959209778,-1.,-1.22453613304507));
#40108=CARTESIAN_POINT('Ctrl Pts',(1.81161420806172,-1.,-1.2187090610323));
#40109=CARTESIAN_POINT('Ctrl Pts',(1.80882996916931,-1.,-1.2129081570818));
#40110=CARTESIAN_POINT('Ctrl Pts',(1.80601678480772,-1.,-1.20713356605519));
#40111=CARTESIAN_POINT('Ctrl Pts',(1.8031745483882,-1.,-1.2013854893912));
#40112=CARTESIAN_POINT('Ctrl Pts',(1.80030314370121,-1.,-1.19566418930405));
#40113=CARTESIAN_POINT('Ctrl Pts',(1.79740245923649,-1.,-1.1899699793456));
#40114=CARTESIAN_POINT('Ctrl Pts',(1.79447240321572,-1.,-1.18430321697471));
#40115=CARTESIAN_POINT('Ctrl Pts',(1.79151291552646,-1.,-1.17866429440781));
#40116=CARTESIAN_POINT('Ctrl Pts',(1.78852398877523,-1.,-1.17305363177265));
#40117=CARTESIAN_POINT('Ctrl Pts',(1.78550566040349,-1.,-1.16747166312239));
#40118=CARTESIAN_POINT('Ctrl Pts',(1.78245795880949,-1.,-1.16191881298458));
#40119=CARTESIAN_POINT('Ctrl Pts',(1.77938085564261,-1.,-1.15639547194689));
#40120=CARTESIAN_POINT('Ctrl Pts',(1.77627422557034,-1.,-1.15090197841531));
#40121=CARTESIAN_POINT('Ctrl Pts',(1.77313777896234,-1.,-1.14543858226948));
#40122=CARTESIAN_POINT('Ctrl Pts',(1.76997111386806,-1.,-1.14000548337));
#40123=CARTESIAN_POINT('Ctrl Pts',(1.76677384551883,-1.,-1.13460291804635));
#40124=CARTESIAN_POINT('Ctrl Pts',(1.76354571966171,-1.,-1.12923123555076));
#40125=CARTESIAN_POINT('Ctrl Pts',(1.76028671825084,-1.,-1.12389096855078));
#40126=CARTESIAN_POINT('Ctrl Pts',(1.75699720772089,-1.,-1.11858293216752));
#40127=CARTESIAN_POINT('Ctrl Pts',(1.75367772094617,-1.,-1.11330807582542));
#40128=CARTESIAN_POINT('Ctrl Pts',(1.75032866075914,-1.,-1.10806728183003));
#40129=CARTESIAN_POINT('Ctrl Pts',(1.74695004214924,-1.,-1.10286118991144));
#40130=CARTESIAN_POINT('Ctrl Pts',(1.74354119236212,-1.,-1.09768999241229));
#40131=CARTESIAN_POINT('Ctrl Pts',(1.74010053962252,-1.,-1.09255329056496));
#40132=CARTESIAN_POINT('Ctrl Pts',(1.73662628326093,-1.,-1.08745056285429));
#40133=CARTESIAN_POINT('Ctrl Pts',(1.73311705663407,-1.,-1.08238162784749));
#40134=CARTESIAN_POINT('Ctrl Pts',(1.72957248977424,-1.,-1.0773470373727));
#40135=CARTESIAN_POINT('Ctrl Pts',(1.72599406198489,-1.,-1.07234866990252));
#40136=CARTESIAN_POINT('Ctrl Pts',(1.72238500928456,-1.,-1.06738966975463));
#40137=CARTESIAN_POINT('Ctrl Pts',(1.71874858456908,-1.,-1.0624732468065));
#40138=CARTESIAN_POINT('Ctrl Pts',(1.71508654427022,-1.,-1.05760163192481));
#40139=CARTESIAN_POINT('Ctrl Pts',(1.71139783543986,-1.,-1.05277517202854));
#40140=CARTESIAN_POINT('Ctrl Pts',(1.70767646263641,-1.,-1.0479908540499));
#40141=CARTESIAN_POINT('Ctrl Pts',(1.70391338707969,-1.,-1.04324363334546));
#40142=CARTESIAN_POINT('Ctrl Pts',(1.70010052930951,-1.,-1.03852922490782));
#40143=CARTESIAN_POINT('Ctrl Pts',(1.69623414782769,-1.,-1.03384646003587));
#40144=CARTESIAN_POINT('Ctrl Pts',(1.69231840863471,-1.,-1.02919977579155));
#40145=CARTESIAN_POINT('Ctrl Pts',(1.68836910178475,-1.,-1.02460180535272));
#40146=CARTESIAN_POINT('Ctrl Pts',(1.68440578021739,-1.,-1.02006795074222));
#40147=CARTESIAN_POINT('Ctrl Pts',(1.6804428989482,-1.,-1.01561026162787));
#40148=CARTESIAN_POINT('Ctrl Pts',(1.67648246776457,-1.,-1.01123236493507));
#40149=CARTESIAN_POINT('Ctrl Pts',(1.67250335383248,-1.,-1.00692206696387));
#40150=CARTESIAN_POINT('Ctrl Pts',(1.66846059277231,-1.,-1.00265091003682));
#40151=CARTESIAN_POINT('Ctrl Pts',(1.66430758030304,-1.,-0.998389654952317));
#40152=CARTESIAN_POINT('Ctrl Pts',(1.66001553809916,-1.,-0.994121836661116));
#40153=CARTESIAN_POINT('Ctrl Pts',(1.65559044289746,-1.,-0.98985562785445));
#40154=CARTESIAN_POINT('Ctrl Pts',(1.6511001661277,-1.,-0.985642622921626));
#40155=CARTESIAN_POINT('Ctrl Pts',(1.64665139190834,-1.,-0.981562530940574));
#40156=CARTESIAN_POINT('Ctrl Pts',(1.64233990826831,-1.,-0.977689794120297));
#40157=CARTESIAN_POINT('Ctrl Pts',(1.63820952658157,-1.,-0.974066058287501));
#40158=CARTESIAN_POINT('Ctrl Pts',(1.63420665729609,-1.,-0.970669715996356));
#40159=CARTESIAN_POINT('Ctrl Pts',(1.63013849959083,-1.,-0.967387853228041));
#40160=CARTESIAN_POINT('Ctrl Pts',(1.6257193066974,-1.,-0.964046107037821));
#40161=CARTESIAN_POINT('Ctrl Pts',(1.62061638139929,-1.,-0.960438326099958));
#40162=CARTESIAN_POINT('Ctrl Pts',(1.61449324337233,-1.,-0.956354422921573));
#40163=CARTESIAN_POINT('Ctrl Pts',(1.60706069897794,-1.,-0.951613284361248));
#40164=CARTESIAN_POINT('Ctrl Pts',(1.59810042045408,-1.,-0.946078063325796));
#40165=CARTESIAN_POINT('Ctrl Pts',(1.58744937489796,-1.,-0.939646377909319));
#40166=CARTESIAN_POINT('Ctrl Pts',(1.57499388385561,-1.,-0.932246680128849));
#40167=CARTESIAN_POINT('Ctrl Pts',(1.56065988582509,-1.,-0.923832188966322));
#40168=CARTESIAN_POINT('Ctrl Pts',(1.54440491152807,-1.,-0.91437591904658));
#40169=CARTESIAN_POINT('Ctrl Pts',(1.52984849890434,-1.,-0.905967409640499));
#40170=CARTESIAN_POINT('Ctrl Pts',(1.51805569591479,-1.,-0.89918504749193));
#40171=CARTESIAN_POINT('Ctrl Pts',(1.50980486807181,-1.,-0.894452006967538));
#40172=CARTESIAN_POINT('Ctrl Pts',(1.5055822144029,-1.,-0.892032620296855));
#40173=CARTESIAN_POINT('',(1.60662857109684,-1.,-0.693717979106306));
#40174=CARTESIAN_POINT('Origin',(0.,-1.,0.));
#40175=CARTESIAN_POINT('',(2.0698113262342,-1.,-0.745574324794401));
#40176=CARTESIAN_POINT('Ctrl Pts',(1.60662857109684,-1.,-0.693717979106306));
#40177=CARTESIAN_POINT('Ctrl Pts',(1.61106790957619,-1.,-0.69571209787897));
#40178=CARTESIAN_POINT('Ctrl Pts',(1.61974673471117,-1.,-0.699605146398837));
#40179=CARTESIAN_POINT('Ctrl Pts',(1.6321654166204,-1.,-0.705159151977294));
#40180=CARTESIAN_POINT('Ctrl Pts',(1.64752408828442,-1.,-0.711993139340448));
#40181=CARTESIAN_POINT('Ctrl Pts',(1.66472880551777,-1.,-0.71958543378795));
#40182=CARTESIAN_POINT('Ctrl Pts',(1.67996158451922,-1.,-0.726235967982445));
#40183=CARTESIAN_POINT('Ctrl Pts',(1.69326921972915,-1.,-0.731963238685357));
#40184=CARTESIAN_POINT('Ctrl Pts',(1.70473309004249,-1.,-0.736799665716932));
#40185=CARTESIAN_POINT('Ctrl Pts',(1.71447789751001,-1.,-0.74079516202821));
#40186=CARTESIAN_POINT('Ctrl Pts',(1.72268229916769,-1.,-0.744021445433094));
#40187=CARTESIAN_POINT('Ctrl Pts',(1.72958533647714,-1.,-0.746574710097752));
#40188=CARTESIAN_POINT('Ctrl Pts',(1.7355035168033,-1.,-0.74858246295687));
#40189=CARTESIAN_POINT('Ctrl Pts',(1.74080458267114,-1.,-0.75019343598125));
#40190=CARTESIAN_POINT('Ctrl Pts',(1.74585086852502,-1.,-0.751555614164483));
#40191=CARTESIAN_POINT('Ctrl Pts',(1.75095139468794,-1.,-0.752797683531314));
#40192=CARTESIAN_POINT('Ctrl Pts',(1.75631083600019,-1.,-0.754009254027829));
#40193=CARTESIAN_POINT('Ctrl Pts',(1.76197817240128,-1.,-0.755220979974462));
#40194=CARTESIAN_POINT('Ctrl Pts',(1.76789396002998,-1.,-0.75642189602781));
#40195=CARTESIAN_POINT('Ctrl Pts',(1.77394167108292,-1.,-0.757578264077029));
#40196=CARTESIAN_POINT('Ctrl Pts',(1.77999411220945,-1.,-0.758650626677519));
#40197=CARTESIAN_POINT('Ctrl Pts',(1.78596964884604,-1.,-0.75961440111019));
#40198=CARTESIAN_POINT('Ctrl Pts',(1.7918581561088,-1.,-0.760469555880749));
#40199=CARTESIAN_POINT('Ctrl Pts',(1.79768986997783,-1.,-0.761229695230558));
#40200=CARTESIAN_POINT('Ctrl Pts',(1.80351583877342,-1.,-0.761915336443547));
#40201=CARTESIAN_POINT('Ctrl Pts',(1.80938551463965,-1.,-0.762546129463938));
#40202=CARTESIAN_POINT('Ctrl Pts',(1.8153211840553,-1.,-0.763132003836634));
#40203=CARTESIAN_POINT('Ctrl Pts',(1.82131873145266,-1.,-0.763673465462727));
#40204=CARTESIAN_POINT('Ctrl Pts',(1.82735991200065,-1.,-0.764165902605995));
#40205=CARTESIAN_POINT('Ctrl Pts',(1.83342077227142,-1.,-0.764602549687853));
#40206=CARTESIAN_POINT('Ctrl Pts',(1.83948181064835,-1.,-0.764978057881738));
#40207=CARTESIAN_POINT('Ctrl Pts',(1.84553698875924,-1.,-0.765291664862029));
#40208=CARTESIAN_POINT('Ctrl Pts',(1.85158945130063,-1.,-0.765545710619063));
#40209=CARTESIAN_POINT('Ctrl Pts',(1.85764741390394,-1.,-0.765744212909319));
#40210=CARTESIAN_POINT('Ctrl Pts',(1.86372027063312,-1.,-0.765891519092547));
#40211=CARTESIAN_POINT('Ctrl Pts',(1.86981398314341,-1.,-0.765990708546091));
#40212=CARTESIAN_POINT('Ctrl Pts',(1.87592888967883,-1.,-0.766042837036744));
#40213=CARTESIAN_POINT('Ctrl Pts',(1.88206215302561,-1.,-0.766047794851865));
#40214=CARTESIAN_POINT('Ctrl Pts',(1.88820926433409,-1.,-0.766004837062091));
#40215=CARTESIAN_POINT('Ctrl Pts',(1.89436577771388,-1.,-0.765913193856978));
#40216=CARTESIAN_POINT('Ctrl Pts',(1.90052930393596,-1.,-0.765772772593386));
#40217=CARTESIAN_POINT('Ctrl Pts',(1.90669961402356,-1.,-0.765584196937919));
#40218=CARTESIAN_POINT('Ctrl Pts',(1.91287765805169,-1.,-0.765348465884722));
#40219=CARTESIAN_POINT('Ctrl Pts',(1.91906491634196,-1.,-0.765066729667089));
#40220=CARTESIAN_POINT('Ctrl Pts',(1.92526263537048,-1.,-0.764740025488212));
#40221=CARTESIAN_POINT('Ctrl Pts',(1.93147105496382,-1.,-0.764369010673941));
#40222=CARTESIAN_POINT('Ctrl Pts',(1.93768964875886,-1.,-0.763954049121459));
#40223=CARTESIAN_POINT('Ctrl Pts',(1.9439174661764,-1.,-0.763495333538629));
#40224=CARTESIAN_POINT('Ctrl Pts',(1.95015342590024,-1.,-0.762992990878769));
#40225=CARTESIAN_POINT('Ctrl Pts',(1.95639665309869,-1.,-0.762447203806179));
#40226=CARTESIAN_POINT('Ctrl Pts',(1.96264672744186,-1.,-0.761858300014424));
#40227=CARTESIAN_POINT('Ctrl Pts',(1.96890351582499,-1.,-0.761226690483821));
#40228=CARTESIAN_POINT('Ctrl Pts',(1.97516705321494,-1.,-0.760552825409757));
#40229=CARTESIAN_POINT('Ctrl Pts',(1.98143741418172,-1.,-0.75983714745219));
#40230=CARTESIAN_POINT('Ctrl Pts',(1.98771456680874,-1.,-0.759080037802488));
#40231=CARTESIAN_POINT('Ctrl Pts',(1.99399831098817,-1.,-0.758281796766761));
#40232=CARTESIAN_POINT('Ctrl Pts',(2.00028834739178,-1.,-0.757442676862724));
#40233=CARTESIAN_POINT('Ctrl Pts',(2.0065843158773,-1.,-0.756562904646671));
#40234=CARTESIAN_POINT('Ctrl Pts',(2.01288584328084,-1.,-0.755642704957865));
#40235=CARTESIAN_POINT('Ctrl Pts',(2.01919259405809,-1.,-0.754682330722816));
#40236=CARTESIAN_POINT('Ctrl Pts',(2.02550428623313,-1.,-0.753682061112768));
#40237=CARTESIAN_POINT('Ctrl Pts',(2.03182068456221,-1.,-0.752642180487211));
#40238=CARTESIAN_POINT('Ctrl Pts',(2.03814160092099,-1.,-0.751562963361115));
#40239=CARTESIAN_POINT('Ctrl Pts',(2.04446689147979,-1.,-0.750444657875576));
#40240=CARTESIAN_POINT('Ctrl Pts',(2.05079645592154,-1.,-0.749287468665046));
#40241=CARTESIAN_POINT('Ctrl Pts',(2.05713023031006,-1.,-0.748091554183803));
#40242=CARTESIAN_POINT('Ctrl Pts',(2.06220058927826,-1.,-0.74710393278792));
#40243=CARTESIAN_POINT('Ctrl Pts',(2.06600523016815,-1.,-0.746345871544201));
#40244=CARTESIAN_POINT('Ctrl Pts',(2.06854248895728,-1.,-0.745832791378367));
#40245=CARTESIAN_POINT('Ctrl Pts',(2.0698113262342,-1.,-0.745574324794401));
#40246=CARTESIAN_POINT('',(2.11275013067528,-1.,-0.61342227326009));
#40247=CARTESIAN_POINT('',(2.0698113262342,-1.,-0.745574324794401));
#40248=CARTESIAN_POINT('',(1.7075470150345,-1.,-0.383122945602004));
#40249=CARTESIAN_POINT('Ctrl Pts',(2.11275013067528,-1.,-0.61342227326009));
#40250=CARTESIAN_POINT('Ctrl Pts',(2.11187554259986,-1.,-0.6124673655618));
#40251=CARTESIAN_POINT('Ctrl Pts',(2.11012443807238,-1.,-0.610560911689899));
#40252=CARTESIAN_POINT('Ctrl Pts',(2.1074919961518,-1.,-0.607711315454876));
#40253=CARTESIAN_POINT('Ctrl Pts',(2.10397049886949,-1.,-0.60393203073603));
#40254=CARTESIAN_POINT('Ctrl Pts',(2.0995493086477,-1.,-0.599241616420534));
#40255=CARTESIAN_POINT('Ctrl Pts',(2.0951087622027,-1.,-0.594585006052162));
#40256=CARTESIAN_POINT('Ctrl Pts',(2.09064881812129,-1.,-0.589962365403406));
#40257=CARTESIAN_POINT('Ctrl Pts',(2.08616943727951,-1.,-0.585373918991617));
#40258=CARTESIAN_POINT('Ctrl Pts',(2.08167059018418,-1.,-0.580819952108064));
#40259=CARTESIAN_POINT('Ctrl Pts',(2.07715226767559,-1.,-0.576300797416845));
#40260=CARTESIAN_POINT('Ctrl Pts',(2.07261449292824,-1.,-0.571816823242603));
#40261=CARTESIAN_POINT('Ctrl Pts',(2.06805732997334,-1.,-0.567368421181087));
#40262=CARTESIAN_POINT('Ctrl Pts',(2.06348090160589,-1.,-0.562955993082262));
#40263=CARTESIAN_POINT('Ctrl Pts',(2.05888537756462,-1.,-0.558579940185152));
#40264=CARTESIAN_POINT('Ctrl Pts',(2.05427091604413,-1.,-0.554240657463906));
#40265=CARTESIAN_POINT('Ctrl Pts',(2.04963761077958,-1.,-0.549938525150295));
#40266=CARTESIAN_POINT('Ctrl Pts',(2.04498544714588,-1.,-0.54567390381743));
#40267=CARTESIAN_POINT('Ctrl Pts',(2.04031422690527,-1.,-0.541447120615659));
#40268=CARTESIAN_POINT('Ctrl Pts',(2.03562362954037,-1.,-0.537258489833262));
#40269=CARTESIAN_POINT('Ctrl Pts',(2.03091336214426,-1.,-0.533108355132977));
#40270=CARTESIAN_POINT('Ctrl Pts',(2.0261832908329,-1.,-0.528997127241914));
#40271=CARTESIAN_POINT('Ctrl Pts',(2.02143356304698,-1.,-0.524925318333476));
#40272=CARTESIAN_POINT('Ctrl Pts',(2.01666477917286,-1.,-0.520893590399371));
#40273=CARTESIAN_POINT('Ctrl Pts',(2.01187773939242,-1.,-0.516902681728687));
#40274=CARTESIAN_POINT('Ctrl Pts',(2.00707309946949,-1.,-0.512953306961793));
#40275=CARTESIAN_POINT('Ctrl Pts',(2.00225107134734,-1.,-0.509046069886157));
#40276=CARTESIAN_POINT('Ctrl Pts',(1.99741107463572,-1.,-0.505181361323026));
#40277=CARTESIAN_POINT('Ctrl Pts',(1.99255149126155,-1.,-0.501359287727146));
#40278=CARTESIAN_POINT('Ctrl Pts',(1.98767044752932,-1.,-0.497579909545574));
#40279=CARTESIAN_POINT('Ctrl Pts',(1.98276658761821,-1.,-0.493843476541495));
#40280=CARTESIAN_POINT('Ctrl Pts',(1.97783973019229,-1.,-0.490150627860953));
#40281=CARTESIAN_POINT('Ctrl Pts',(1.97289186263272,-1.,-0.486502692907659));
#40282=CARTESIAN_POINT('Ctrl Pts',(1.96792703422362,-1.,-0.482901662120691));
#40283=CARTESIAN_POINT('Ctrl Pts',(1.96294933055943,-1.,-0.479349583074855));
#40284=CARTESIAN_POINT('Ctrl Pts',(1.95796111148177,-1.,-0.475848034683176));
#40285=CARTESIAN_POINT('Ctrl Pts',(1.95296148278133,-1.,-0.472397672264072));
#40286=CARTESIAN_POINT('Ctrl Pts',(1.94794381136514,-1.,-0.468997482913135));
#40287=CARTESIAN_POINT('Ctrl Pts',(1.9428979419619,-1.,-0.46564546202603));
#40288=CARTESIAN_POINT('Ctrl Pts',(1.93781486640821,-1.,-0.462340031009057));
#40289=CARTESIAN_POINT('Ctrl Pts',(1.93269066517934,-1.,-0.459081234547926));
#40290=CARTESIAN_POINT('Ctrl Pts',(1.92753067150476,-1.,-0.455872005174371));
#40291=CARTESIAN_POINT('Ctrl Pts',(1.92235380648502,-1.,-0.452719478359433));
#40292=CARTESIAN_POINT('Ctrl Pts',(1.91718342555755,-1.,-0.449632260106662));
#40293=CARTESIAN_POINT('Ctrl Pts',(1.9120369998112,-1.,-0.446617343485711));
#40294=CARTESIAN_POINT('Ctrl Pts',(1.90691756144898,-1.,-0.443677556849151));
#40295=CARTESIAN_POINT('Ctrl Pts',(1.90180124389086,-1.,-0.440807833704038));
#40296=CARTESIAN_POINT('Ctrl Pts',(1.89663648956466,-1.,-0.437995003948244));
#40297=CARTESIAN_POINT('Ctrl Pts',(1.89136993975504,-1.,-0.435225660963383));
#40298=CARTESIAN_POINT('Ctrl Pts',(1.88596913666793,-1.,-0.432493038548748));
#40299=CARTESIAN_POINT('Ctrl Pts',(1.88044229001832,-1.,-0.429803062482345));
#40300=CARTESIAN_POINT('Ctrl Pts',(1.87486989291484,-1.,-0.427183828519102));
#40301=CARTESIAN_POINT('Ctrl Pts',(1.86937803944323,-1.,-0.424678177291359));
#40302=CARTESIAN_POINT('Ctrl Pts',(1.86408083334028,-1.,-0.422327307418275));
#40303=CARTESIAN_POINT('Ctrl Pts',(1.85903281096686,-1.,-0.42015728797562));
#40304=CARTESIAN_POINT('Ctrl Pts',(1.85417632856234,-1.,-0.418164129143534));
#40305=CARTESIAN_POINT('Ctrl Pts',(1.84929312929882,-1.,-0.416300022038864));
#40306=CARTESIAN_POINT('Ctrl Pts',(1.8440575707371,-1.,-0.41448743825434));
#40307=CARTESIAN_POINT('Ctrl Pts',(1.83808953475839,-1.,-0.412633125322162));
#40308=CARTESIAN_POINT('Ctrl Pts',(1.83100408895216,-1.,-0.410641256301675));
#40309=CARTESIAN_POINT('Ctrl Pts',(1.8224702267854,-1.,-0.408428948108534));
#40310=CARTESIAN_POINT('Ctrl Pts',(1.81223801813988,-1.,-0.405933518411838));
#40311=CARTESIAN_POINT('Ctrl Pts',(1.80012077176221,-1.,-0.403107976170441));
#40312=CARTESIAN_POINT('Ctrl Pts',(1.78598826347533,-1.,-0.399919403783081));
#40313=CARTESIAN_POINT('Ctrl Pts',(1.7697556004756,-1.,-0.39634619612042));
#40314=CARTESIAN_POINT('Ctrl Pts',(1.75137405313962,-1.,-0.392375812294307));
#40315=CARTESIAN_POINT('Ctrl Pts',(1.7349317097561,-1.,-0.388877023509192));
#40316=CARTESIAN_POINT('Ctrl Pts',(1.72162022246158,-1.,-0.38607079032701));
#40317=CARTESIAN_POINT('Ctrl Pts',(1.71231062891958,-1.,-0.384119047315542));
#40318=CARTESIAN_POINT('Ctrl Pts',(1.7075470150345,-1.,-0.383122945602004));
#40319=CARTESIAN_POINT('',(1.74236521665491,-1.,-0.163289472382896));
#40320=CARTESIAN_POINT('Origin',(0.,-1.,0.));
#40321=CARTESIAN_POINT('',(2.19890268624765,-1.,-0.0694764450219582));
#40322=CARTESIAN_POINT('Ctrl Pts',(1.74236521665491,-1.,-0.163289472382896));
#40323=CARTESIAN_POINT('Ctrl Pts',(1.7472034950333,-1.,-0.163814161002002));
#40324=CARTESIAN_POINT('Ctrl Pts',(1.75666056638427,-1.,-0.164834765707159));
#40325=CARTESIAN_POINT('Ctrl Pts',(1.77018771684844,-1.,-0.1662793551464));
#40326=CARTESIAN_POINT('Ctrl Pts',(1.7869064998507,-1.,-0.168032772805197));
#40327=CARTESIAN_POINT('Ctrl Pts',(1.80561530629706,-1.,-0.169936923904608));
#40328=CARTESIAN_POINT('Ctrl Pts',(1.82215766811545,-1.,-0.171554770204119));
#40329=CARTESIAN_POINT('Ctrl Pts',(1.83658380527692,-1.,-0.1728894428919));
#40330=CARTESIAN_POINT('Ctrl Pts',(1.8489811319852,-1.,-0.173946627587732));
#40331=CARTESIAN_POINT('Ctrl Pts',(1.85948367088837,-1.,-0.17473525927603));
#40332=CARTESIAN_POINT('Ctrl Pts',(1.86828349694799,-1.,-0.175268337590758));
#40333=CARTESIAN_POINT('Ctrl Pts',(1.87563767773588,-1.,-0.175563480746485));
#40334=CARTESIAN_POINT('Ctrl Pts',(1.88188663145367,-1.,-0.175644148889699));
#40335=CARTESIAN_POINT('Ctrl Pts',(1.88742606273259,-1.,-0.175538155840648));
#40336=CARTESIAN_POINT('Ctrl Pts',(1.892646301985,-1.,-0.175274276190844));
#40337=CARTESIAN_POINT('Ctrl Pts',(1.89788101117132,-1.,-0.174879405091263));
#40338=CARTESIAN_POINT('Ctrl Pts',(1.90335253862834,-1.,-0.174375518661085));
#40339=CARTESIAN_POINT('Ctrl Pts',(1.90911693975267,-1.,-0.173776635257817));
#40340=CARTESIAN_POINT('Ctrl Pts',(1.91511429159527,-1.,-0.173090695383496));
#40341=CARTESIAN_POINT('Ctrl Pts',(1.9212233439798,-1.,-0.172321621259514));
#40342=CARTESIAN_POINT('Ctrl Pts',(1.92731093582036,-1.,-0.171471191532988));
#40343=CARTESIAN_POINT('Ctrl Pts',(1.93329183155539,-1.,-0.170541253116202));
#40344=CARTESIAN_POINT('Ctrl Pts',(1.93915639211581,-1.,-0.169534904817491));
#40345=CARTESIAN_POINT('Ctrl Pts',(1.94493757756931,-1.,-0.168455741607556));
#40346=CARTESIAN_POINT('Ctrl Pts',(1.95069027794294,-1.,-0.167307501784476));
#40347=CARTESIAN_POINT('Ctrl Pts',(1.9564675971873,-1.,-0.166093592002813));
#40348=CARTESIAN_POINT('Ctrl Pts',(1.96229379940136,-1.,-0.164816568920269));
#40349=CARTESIAN_POINT('Ctrl Pts',(1.96816512677967,-1.,-0.163478185457734));
#40350=CARTESIAN_POINT('Ctrl Pts',(1.97406280235188,-1.,-0.162079693556289));
#40351=CARTESIAN_POINT('Ctrl Pts',(1.97996195437559,-1.,-0.160622060784611));
#40352=CARTESIAN_POINT('Ctrl Pts',(1.98584238283292,-1.,-0.159106226437299));
#40353=CARTESIAN_POINT('Ctrl Pts',(1.99169810931908,-1.,-0.157533331459227));
#40354=CARTESIAN_POINT('Ctrl Pts',(1.99753284771497,-1.,-0.155904629548784));
#40355=CARTESIAN_POINT('Ctrl Pts',(2.00335565310543,-1.,-0.154221403049722));
#40356=CARTESIAN_POINT('Ctrl Pts',(2.00917680318424,-1.,-0.15248488362145));
#40357=CARTESIAN_POINT('Ctrl Pts',(2.01500291940238,-1.,-0.150696157673078));
#40358=CARTESIAN_POINT('Ctrl Pts',(2.02083464969894,-1.,-0.148856124775337));
#40359=CARTESIAN_POINT('Ctrl Pts',(2.02666926182017,-1.,-0.146965557332583));
#40360=CARTESIAN_POINT('Ctrl Pts',(2.03250223739942,-1.,-0.145025140186058));
#40361=CARTESIAN_POINT('Ctrl Pts',(2.03832911025912,-1.,-0.143035515058209));
#40362=CARTESIAN_POINT('Ctrl Pts',(2.04414757947916,-1.,-0.140997332152546));
#40363=CARTESIAN_POINT('Ctrl Pts',(2.04995762001328,-1.,-0.138911255368966));
#40364=CARTESIAN_POINT('Ctrl Pts',(2.05576044414264,-1.,-0.136777941218044));
#40365=CARTESIAN_POINT('Ctrl Pts',(2.06155781517842,-1.,-0.134598026192106));
#40366=CARTESIAN_POINT('Ctrl Pts',(2.06735123910326,-1.,-0.132372111547711));
#40367=CARTESIAN_POINT('Ctrl Pts',(2.07314114713063,-1.,-0.130100748328404));
#40368=CARTESIAN_POINT('Ctrl Pts',(2.07892715110987,-1.,-0.12778444527612));
#40369=CARTESIAN_POINT('Ctrl Pts',(2.08470840653643,-1.,-0.125423679412062));
#40370=CARTESIAN_POINT('Ctrl Pts',(2.09048392424825,-1.,-0.123018905621083));
#40371=CARTESIAN_POINT('Ctrl Pts',(2.0962529286773,-1.,-0.120570567965122));
#40372=CARTESIAN_POINT('Ctrl Pts',(2.102015121329,-1.,-0.118079107988356));
#40373=CARTESIAN_POINT('Ctrl Pts',(2.10777050261309,-1.,-0.115544957687927));
#40374=CARTESIAN_POINT('Ctrl Pts',(2.11351924490306,-1.,-0.112968534419737));
#40375=CARTESIAN_POINT('Ctrl Pts',(2.11926155590865,-1.,-0.110350236135025));
#40376=CARTESIAN_POINT('Ctrl Pts',(2.12499752307,-1.,-0.10769043523109));
#40377=CARTESIAN_POINT('Ctrl Pts',(2.13072704887293,-1.,-0.10498947915274));
#40378=CARTESIAN_POINT('Ctrl Pts',(2.13644992667165,-1.,-0.102247700556101));
#40379=CARTESIAN_POINT('Ctrl Pts',(2.14216588396025,-1.,-0.0994654261990917));
#40380=CARTESIAN_POINT('Ctrl Pts',(2.14787463531795,-1.,-0.096642985230546));
#40381=CARTESIAN_POINT('Ctrl Pts',(2.1535759397817,-1.,-0.0937807218867645));
#40382=CARTESIAN_POINT('Ctrl Pts',(2.15926961544516,-1.,-0.0908789888107267));
#40383=CARTESIAN_POINT('Ctrl Pts',(2.16495552645014,-1.,-0.0879381291386924));
#40384=CARTESIAN_POINT('Ctrl Pts',(2.17063357870952,-1.,-0.0849584620835374));
#40385=CARTESIAN_POINT('Ctrl Pts',(2.176303712113,-1.,-0.0819402680872767));
#40386=CARTESIAN_POINT('Ctrl Pts',(2.18196589448887,-1.,-0.0788837727685244));
#40387=CARTESIAN_POINT('Ctrl Pts',(2.1876201139953,-1.,-0.0757891465836149));
#40388=CARTESIAN_POINT('Ctrl Pts',(2.19213712013662,-1.,-0.0732830357306726));
#40389=CARTESIAN_POINT('Ctrl Pts',(2.19552129484002,-1.,-0.0713863779526155));
#40390=CARTESIAN_POINT('Ctrl Pts',(2.19777582085423,-1.,-0.0701143536325491));
#40391=CARTESIAN_POINT('Ctrl Pts',(2.19890268624765,-1.,-0.0694764450219582));
#40392=CARTESIAN_POINT('',(2.19890268624765,-1.,0.0694764450219582));
#40393=CARTESIAN_POINT('',(2.19890268624765,-1.,-0.0694764450219582));
#40394=CARTESIAN_POINT('',(1.74236521665491,-1.,0.163289472382896));
#40395=CARTESIAN_POINT('Ctrl Pts',(2.19890268624765,-1.,0.0694764450219582));
#40396=CARTESIAN_POINT('Ctrl Pts',(2.19777582085261,-1.,0.0701143536324925));
#40397=CARTESIAN_POINT('Ctrl Pts',(2.19552129483562,-1.,0.0713863779524626));
#40398=CARTESIAN_POINT('Ctrl Pts',(2.19213712012956,-1.,0.0732830357304275));
#40399=CARTESIAN_POINT('Ctrl Pts',(2.1876201139874,-1.,0.075789146583341));
#40400=CARTESIAN_POINT('Ctrl Pts',(2.18196589448304,-1.,0.0788837727683226));
#40401=CARTESIAN_POINT('Ctrl Pts',(2.1763037121106,-1.,0.0819402680871938));
#40402=CARTESIAN_POINT('Ctrl Pts',(2.17063357871031,-1.,0.0849584620835642));
#40403=CARTESIAN_POINT('Ctrl Pts',(2.16495552645275,-1.,0.0879381291387821));
#40404=CARTESIAN_POINT('Ctrl Pts',(2.15926961544808,-1.,0.0908789888108265));
#40405=CARTESIAN_POINT('Ctrl Pts',(2.15357593978377,-1.,0.0937807218868344));
#40406=CARTESIAN_POINT('Ctrl Pts',(2.14787463531864,-1.,0.0966429852305688));
#40407=CARTESIAN_POINT('Ctrl Pts',(2.14216588395974,-1.,0.0994654261990741));
#40408=CARTESIAN_POINT('Ctrl Pts',(2.13644992667052,-1.,0.102247700556063));
#40409=CARTESIAN_POINT('Ctrl Pts',(2.1307270488718,-1.,0.104989479152703));
#40410=CARTESIAN_POINT('Ctrl Pts',(2.12499752306927,-1.,0.107690435231068));
#40411=CARTESIAN_POINT('Ctrl Pts',(2.11926155590849,-1.,0.11035023613502));
#40412=CARTESIAN_POINT('Ctrl Pts',(2.11351924490335,-1.,0.112968534419746));
#40413=CARTESIAN_POINT('Ctrl Pts',(2.10777050261359,-1.,0.11554495768794));
#40414=CARTESIAN_POINT('Ctrl Pts',(2.10201512132945,-1.,0.118079107988368));
#40415=CARTESIAN_POINT('Ctrl Pts',(2.09625292867756,-1.,0.120570567965129));
#40416=CARTESIAN_POINT('Ctrl Pts',(2.09048392424826,-1.,0.123018905621083));
#40417=CARTESIAN_POINT('Ctrl Pts',(2.08470840653628,-1.,0.125423679412058));
#40418=CARTESIAN_POINT('Ctrl Pts',(2.07892715110967,-1.,0.127784445276116));
#40419=CARTESIAN_POINT('Ctrl Pts',(2.07314114713047,-1.,0.1301007483284));
#40420=CARTESIAN_POINT('Ctrl Pts',(2.06735123910319,-1.,0.132372111547709));
#40421=CARTESIAN_POINT('Ctrl Pts',(2.06155781517844,-1.,0.134598026192107));
#40422=CARTESIAN_POINT('Ctrl Pts',(2.0557604441427,-1.,0.136777941218044));
#40423=CARTESIAN_POINT('Ctrl Pts',(2.04995762001333,-1.,0.138911255368966));
#40424=CARTESIAN_POINT('Ctrl Pts',(2.04414757947919,-1.,0.140997332152545));
#40425=CARTESIAN_POINT('Ctrl Pts',(2.03832911025913,-1.,0.143035515058208));
#40426=CARTESIAN_POINT('Ctrl Pts',(2.03250223739941,-1.,0.145025140186058));
#40427=CARTESIAN_POINT('Ctrl Pts',(2.02666926182017,-1.,0.146965557332586));
#40428=CARTESIAN_POINT('Ctrl Pts',(2.02083464969897,-1.,0.148856124775342));
#40429=CARTESIAN_POINT('Ctrl Pts',(2.01500291940243,-1.,0.150696157673084));
#40430=CARTESIAN_POINT('Ctrl Pts',(2.00917680318426,-1.,0.152484883621452));
#40431=CARTESIAN_POINT('Ctrl Pts',(2.00335565310539,-1.,0.154221403049719));
#40432=CARTESIAN_POINT('Ctrl Pts',(1.99753284771487,-1.,0.155904629548774));
#40433=CARTESIAN_POINT('Ctrl Pts',(1.99169810931893,-1.,0.157533331459215));
#40434=CARTESIAN_POINT('Ctrl Pts',(1.98584238283279,-1.,0.159106226437288));
#40435=CARTESIAN_POINT('Ctrl Pts',(1.97996195437557,-1.,0.16062206078461));
#40436=CARTESIAN_POINT('Ctrl Pts',(1.97406280235204,-1.,0.162079693556302));
#40437=CARTESIAN_POINT('Ctrl Pts',(1.96816512678,-1.,0.16347818545776));
#40438=CARTESIAN_POINT('Ctrl Pts',(1.96229379940174,-1.,0.1648165689203));
#40439=CARTESIAN_POINT('Ctrl Pts',(1.95646759718755,-1.,0.166093592002832));
#40440=CARTESIAN_POINT('Ctrl Pts',(1.95069027794286,-1.,0.167307501784469));
#40441=CARTESIAN_POINT('Ctrl Pts',(1.94493757756879,-1.,0.168455741607515));
#40442=CARTESIAN_POINT('Ctrl Pts',(1.93915639211497,-1.,0.169534904817425));
#40443=CARTESIAN_POINT('Ctrl Pts',(1.93329183155455,-1.,0.170541253116136));
#40444=CARTESIAN_POINT('Ctrl Pts',(1.92731093582,-1.,0.17147119153296));
#40445=CARTESIAN_POINT('Ctrl Pts',(1.92122334398034,-1.,0.172321621259556));
#40446=CARTESIAN_POINT('Ctrl Pts',(1.91511429159681,-1.,0.173090695383619));
#40447=CARTESIAN_POINT('Ctrl Pts',(1.90911693975475,-1.,0.173776635257983));
#40448=CARTESIAN_POINT('Ctrl Pts',(1.90335253863003,-1.,0.174375518661222));
#40449=CARTESIAN_POINT('Ctrl Pts',(1.89788101117148,-1.,0.174879405091277));
#40450=CARTESIAN_POINT('Ctrl Pts',(1.89264630198279,-1.,0.175274276190664));
#40451=CARTESIAN_POINT('Ctrl Pts',(1.88742606272818,-1.,0.175538155840286));
#40452=CARTESIAN_POINT('Ctrl Pts',(1.88188663144846,-1.,0.175644148889271));
#40453=CARTESIAN_POINT('Ctrl Pts',(1.87563767773249,-1.,0.175563480746205));
#40454=CARTESIAN_POINT('Ctrl Pts',(1.86828349694972,-1.,0.1752683375909));
#40455=CARTESIAN_POINT('Ctrl Pts',(1.85948367089838,-1.,0.174735259276856));
#40456=CARTESIAN_POINT('Ctrl Pts',(1.84898113200543,-1.,0.173946627589401));
#40457=CARTESIAN_POINT('Ctrl Pts',(1.83658380530747,-1.,0.17288944289442));
#40458=CARTESIAN_POINT('Ctrl Pts',(1.82215766815414,-1.,0.171554770207306));
#40459=CARTESIAN_POINT('Ctrl Pts',(1.80561530633924,-1.,0.169936923908078));
#40460=CARTESIAN_POINT('Ctrl Pts',(1.78690649988931,-1.,0.16803277280837));
#40461=CARTESIAN_POINT('Ctrl Pts',(1.77018771687692,-1.,0.166279355148738));
#40462=CARTESIAN_POINT('Ctrl Pts',(1.75666056640041,-1.,0.164834765708484));
#40463=CARTESIAN_POINT('Ctrl Pts',(1.74720349503904,-1.,0.163814161002474));
#40464=CARTESIAN_POINT('Ctrl Pts',(1.74236521665491,-1.,0.163289472382896));
#40465=CARTESIAN_POINT('',(1.7075470150345,-1.,0.383122945602004));
#40466=CARTESIAN_POINT('Origin',(0.,-1.,0.));
#40467=CARTESIAN_POINT('',(2.11275013067528,-1.,0.613422273260091));
#40468=CARTESIAN_POINT('Ctrl Pts',(1.7075470150345,-1.,0.383122945602004));
#40469=CARTESIAN_POINT('Ctrl Pts',(1.71231062891398,-1.,0.384119047314215));
#40470=CARTESIAN_POINT('Ctrl Pts',(1.72162022244582,-1.,0.386070790323281));
#40471=CARTESIAN_POINT('Ctrl Pts',(1.73493170972829,-1.,0.388877023502615));
#40472=CARTESIAN_POINT('Ctrl Pts',(1.75137405310193,-1.,0.392375812285396));
#40473=CARTESIAN_POINT('Ctrl Pts',(1.76975560043442,-1.,0.396346196110688));
#40474=CARTESIAN_POINT('Ctrl Pts',(1.78598826343754,-1.,0.399919403774156));
#40475=CARTESIAN_POINT('Ctrl Pts',(1.80012077173238,-1.,0.403107976163396));
#40476=CARTESIAN_POINT('Ctrl Pts',(1.81223801812013,-1.,0.405933518407176));
#40477=CARTESIAN_POINT('Ctrl Pts',(1.82247022677562,-1.,0.408428948106228));
#40478=CARTESIAN_POINT('Ctrl Pts',(1.83100408895047,-1.,0.410641256301276));
#40479=CARTESIAN_POINT('Ctrl Pts',(1.8380895347617,-1.,0.412633125322945));
#40480=CARTESIAN_POINT('Ctrl Pts',(1.84405757074218,-1.,0.414487438255542));
#40481=CARTESIAN_POINT('Ctrl Pts',(1.84929312930314,-1.,0.416300022039885));
#40482=CARTESIAN_POINT('Ctrl Pts',(1.8541763285645,-1.,0.418164129144046));
#40483=CARTESIAN_POINT('Ctrl Pts',(1.8590328109667,-1.,0.420157287975583));
#40484=CARTESIAN_POINT('Ctrl Pts',(1.86408083333863,-1.,0.422327307417885));
#40485=CARTESIAN_POINT('Ctrl Pts',(1.8693780394412,-1.,0.424678177290876));
#40486=CARTESIAN_POINT('Ctrl Pts',(1.87486989291333,-1.,0.427183828518743));
#40487=CARTESIAN_POINT('Ctrl Pts',(1.88044229001778,-1.,0.429803062482217));
#40488=CARTESIAN_POINT('Ctrl Pts',(1.88596913666828,-1.,0.432493038548833));
#40489=CARTESIAN_POINT('Ctrl Pts',(1.89136993975585,-1.,0.43522566096358));
#40490=CARTESIAN_POINT('Ctrl Pts',(1.89663648956549,-1.,0.437995003948443));
#40491=CARTESIAN_POINT('Ctrl Pts',(1.90180124389137,-1.,0.440807833704161));
#40492=CARTESIAN_POINT('Ctrl Pts',(1.90691756144906,-1.,0.443677556849171));
#40493=CARTESIAN_POINT('Ctrl Pts',(1.91203699981095,-1.,0.446617343485651));
#40494=CARTESIAN_POINT('Ctrl Pts',(1.91718342555717,-1.,0.449632260106572));
#40495=CARTESIAN_POINT('Ctrl Pts',(1.9223538064847,-1.,0.452719478359356));
#40496=CARTESIAN_POINT('Ctrl Pts',(1.92753067150461,-1.,0.455872005174336));
#40497=CARTESIAN_POINT('Ctrl Pts',(1.93269066517936,-1.,0.459081234547932));
#40498=CARTESIAN_POINT('Ctrl Pts',(1.93781486640834,-1.,0.462340031009087));
#40499=CARTESIAN_POINT('Ctrl Pts',(1.94289794196205,-1.,0.465645462026065));
#40500=CARTESIAN_POINT('Ctrl Pts',(1.94794381136524,-1.,0.468997482913158));
#40501=CARTESIAN_POINT('Ctrl Pts',(1.95296148278136,-1.,0.47239767226408));
#40502=CARTESIAN_POINT('Ctrl Pts',(1.95796111148175,-1.,0.475848034683172));
#40503=CARTESIAN_POINT('Ctrl Pts',(1.96294933055938,-1.,0.479349583074846));
#40504=CARTESIAN_POINT('Ctrl Pts',(1.96792703422358,-1.,0.482901662120687));
#40505=CARTESIAN_POINT('Ctrl Pts',(1.97289186263272,-1.,0.486502692907661));
#40506=CARTESIAN_POINT('Ctrl Pts',(1.97783973019229,-1.,0.490150627860955));
#40507=CARTESIAN_POINT('Ctrl Pts',(1.9827665876182,-1.,0.493843476541493));
#40508=CARTESIAN_POINT('Ctrl Pts',(1.98767044752929,-1.,0.497579909545564));
#40509=CARTESIAN_POINT('Ctrl Pts',(1.9925514912615,-1.,0.501359287727129));
#40510=CARTESIAN_POINT('Ctrl Pts',(1.99741107463567,-1.,0.505181361323011));
#40511=CARTESIAN_POINT('Ctrl Pts',(2.00225107134733,-1.,0.509046069886152));
#40512=CARTESIAN_POINT('Ctrl Pts',(2.00707309946955,-1.,0.512953306961814));
#40513=CARTESIAN_POINT('Ctrl Pts',(2.01187773939257,-1.,0.516902681728733));
#40514=CARTESIAN_POINT('Ctrl Pts',(2.01666477917305,-1.,0.520893590399429));
#40515=CARTESIAN_POINT('Ctrl Pts',(2.02143356304712,-1.,0.524925318333519));
#40516=CARTESIAN_POINT('Ctrl Pts',(2.02618329083289,-1.,0.528997127241911));
#40517=CARTESIAN_POINT('Ctrl Pts',(2.03091336214401,-1.,0.533108355132905));
#40518=CARTESIAN_POINT('Ctrl Pts',(2.03562362953993,-1.,0.537258489833135));
#40519=CARTESIAN_POINT('Ctrl Pts',(2.0403142269048,-1.,0.54144712061552));
#40520=CARTESIAN_POINT('Ctrl Pts',(2.0449854471456,-1.,0.545673903817349));
#40521=CARTESIAN_POINT('Ctrl Pts',(2.04963761077974,-1.,0.549938525150342));
#40522=CARTESIAN_POINT('Ctrl Pts',(2.05427091604482,-1.,0.55424065746411));
#40523=CARTESIAN_POINT('Ctrl Pts',(2.05888537756571,-1.,0.558579940185468));
#40524=CARTESIAN_POINT('Ctrl Pts',(2.06348090160697,-1.,0.562955993082574));
#40525=CARTESIAN_POINT('Ctrl Pts',(2.06805732997383,-1.,0.56736842118123));
#40526=CARTESIAN_POINT('Ctrl Pts',(2.07261449292757,-1.,0.571816823242411));
#40527=CARTESIAN_POINT('Ctrl Pts',(2.07715226767361,-1.,0.576300797416275));
#40528=CARTESIAN_POINT('Ctrl Pts',(2.08167059018138,-1.,0.580819952107257));
#40529=CARTESIAN_POINT('Ctrl Pts',(2.086169437277,-1.,0.585373918990895));
#40530=CARTESIAN_POINT('Ctrl Pts',(2.09064881812053,-1.,0.58996236540319));
#40531=CARTESIAN_POINT('Ctrl Pts',(2.09510876220501,-1.,0.594585006052824));
#40532=CARTESIAN_POINT('Ctrl Pts',(2.09954930865331,-1.,0.599241616422144));
#40533=CARTESIAN_POINT('Ctrl Pts',(2.10397049887709,-1.,0.603932030738212));
#40534=CARTESIAN_POINT('Ctrl Pts',(2.10749199615859,-1.,0.607711315456826));
#40535=CARTESIAN_POINT('Ctrl Pts',(2.11012443807661,-1.,0.610560911691114));
#40536=CARTESIAN_POINT('Ctrl Pts',(2.11187554260142,-1.,0.61246736556225));
#40537=CARTESIAN_POINT('Ctrl Pts',(2.11275013067528,-1.,0.613422273260091));
#40538=CARTESIAN_POINT('',(2.0698113262342,-1.,0.745574324794401));
#40539=CARTESIAN_POINT('',(2.11275013067528,-1.,0.613422273260091));
#40540=CARTESIAN_POINT('Ctrl Pts',(2.0698113262342,-1.,0.745574324794401));
#40541=CARTESIAN_POINT('Ctrl Pts',(2.06854248895575,-1.,0.74583279137781));
#40542=CARTESIAN_POINT('Ctrl Pts',(2.06600523016401,-1.,0.746345871542696));
#40543=CARTESIAN_POINT('Ctrl Pts',(2.06220058927162,-1.,0.747103932785504));
#40544=CARTESIAN_POINT('Ctrl Pts',(2.05713023030263,-1.,0.748091554181101));
#40545=CARTESIAN_POINT('Ctrl Pts',(2.05079645591606,-1.,0.749287468663053));
#40546=CARTESIAN_POINT('Ctrl Pts',(2.04446689147754,-1.,0.750444657874758));
#40547=CARTESIAN_POINT('Ctrl Pts',(2.03814160092173,-1.,0.751562963361384));
#40548=CARTESIAN_POINT('Ctrl Pts',(2.03182068456467,-1.,0.752642180488104));
#40549=CARTESIAN_POINT('Ctrl Pts',(2.02550428623587,-1.,0.753682061113766));
#40550=CARTESIAN_POINT('Ctrl Pts',(2.01919259406003,-1.,0.75468233072352));
#40551=CARTESIAN_POINT('Ctrl Pts',(2.01288584328149,-1.,0.755642704958101));
#40552=CARTESIAN_POINT('Ctrl Pts',(2.00658431587682,-1.,0.756562904646496));
#40553=CARTESIAN_POINT('Ctrl Pts',(2.00028834739072,-1.,0.757442676862342));
#40554=CARTESIAN_POINT('Ctrl Pts',(1.9939983109871,-1.,0.758281796766377));
#40555=CARTESIAN_POINT('Ctrl Pts',(1.98771456680806,-1.,0.759080037802243));
#40556=CARTESIAN_POINT('Ctrl Pts',(1.98143741418156,-1.,0.759837147452135));
#40557=CARTESIAN_POINT('Ctrl Pts',(1.97516705321521,-1.,0.760552825409856));
#40558=CARTESIAN_POINT('Ctrl Pts',(1.96890351582545,-1.,0.761226690483986));
#40559=CARTESIAN_POINT('Ctrl Pts',(1.96264672744229,-1.,0.761858300014575));
#40560=CARTESIAN_POINT('Ctrl Pts',(1.95639665309893,-1.,0.762447203806264));
#40561=CARTESIAN_POINT('Ctrl Pts',(1.95015342590025,-1.,0.762992990878774));
#40562=CARTESIAN_POINT('Ctrl Pts',(1.94391746617626,-1.,0.763495333538581));
#40563=CARTESIAN_POINT('Ctrl Pts',(1.93768964875867,-1.,0.763954049121394));
#40564=CARTESIAN_POINT('Ctrl Pts',(1.93147105496367,-1.,0.76436901067389));
#40565=CARTESIAN_POINT('Ctrl Pts',(1.92526263537041,-1.,0.764740025488189));
#40566=CARTESIAN_POINT('Ctrl Pts',(1.91906491634197,-1.,0.765066729667095));
#40567=CARTESIAN_POINT('Ctrl Pts',(1.91287765805174,-1.,0.765348465884739));
#40568=CARTESIAN_POINT('Ctrl Pts',(1.90669961402362,-1.,0.765584196937937));
#40569=CARTESIAN_POINT('Ctrl Pts',(1.90052930393599,-1.,0.765772772593395));
#40570=CARTESIAN_POINT('Ctrl Pts',(1.89436577771389,-1.,0.765913193856979));
#40571=CARTESIAN_POINT('Ctrl Pts',(1.88820926433409,-1.,0.76600483706209));
#40572=CARTESIAN_POINT('Ctrl Pts',(1.88206215302561,-1.,0.766047794851869));
#40573=CARTESIAN_POINT('Ctrl Pts',(1.87592888967886,-1.,0.766042837036759));
#40574=CARTESIAN_POINT('Ctrl Pts',(1.86981398314345,-1.,0.765990708546112));
#40575=CARTESIAN_POINT('Ctrl Pts',(1.86372027063314,-1.,0.765891519092557));
#40576=CARTESIAN_POINT('Ctrl Pts',(1.85764741390391,-1.,0.765744212909305));
#40577=CARTESIAN_POINT('Ctrl Pts',(1.85158945130054,-1.,0.765545710619023));
#40578=CARTESIAN_POINT('Ctrl Pts',(1.8455369887591,-1.,0.765291664861972));
#40579=CARTESIAN_POINT('Ctrl Pts',(1.83948181064823,-1.,0.764978057881688));
#40580=CARTESIAN_POINT('Ctrl Pts',(1.8334207722714,-1.,0.764602549687846));
#40581=CARTESIAN_POINT('Ctrl Pts',(1.8273599120008,-1.,0.764165902606056));
#40582=CARTESIAN_POINT('Ctrl Pts',(1.82131873145297,-1.,0.763673465462854));
#40583=CARTESIAN_POINT('Ctrl Pts',(1.81532118405566,-1.,0.763132003836783));
#40584=CARTESIAN_POINT('Ctrl Pts',(1.80938551463989,-1.,0.762546129464036));
#40585=CARTESIAN_POINT('Ctrl Pts',(1.80351583877334,-1.,0.761915336443516));
#40586=CARTESIAN_POINT('Ctrl Pts',(1.79768986997735,-1.,0.761229695230359));
#40587=CARTESIAN_POINT('Ctrl Pts',(1.79185815610802,-1.,0.760469555880425));
#40588=CARTESIAN_POINT('Ctrl Pts',(1.78596964884526,-1.,0.759614401109868));
#40589=CARTESIAN_POINT('Ctrl Pts',(1.77999411220912,-1.,0.75865062667738));
#40590=CARTESIAN_POINT('Ctrl Pts',(1.77394167108342,-1.,0.757578264077238));
#40591=CARTESIAN_POINT('Ctrl Pts',(1.76789396003141,-1.,0.756421896028403));
#40592=CARTESIAN_POINT('Ctrl Pts',(1.7619781724032,-1.,0.755220979975262));
#40593=CARTESIAN_POINT('Ctrl Pts',(1.75631083600175,-1.,0.75400925402848));
#40594=CARTESIAN_POINT('Ctrl Pts',(1.75095139468809,-1.,0.752797683531377));
#40595=CARTESIAN_POINT('Ctrl Pts',(1.74585086852298,-1.,0.751555614163629));
#40596=CARTESIAN_POINT('Ctrl Pts',(1.74080458266705,-1.,0.750193435979541));
#40597=CARTESIAN_POINT('Ctrl Pts',(1.73550351679848,-1.,0.748582462954855));
#40598=CARTESIAN_POINT('Ctrl Pts',(1.72958533647399,-1.,0.746574710096437));
#40599=CARTESIAN_POINT('Ctrl Pts',(1.7226822991693,-1.,0.744021445433765));
#40600=CARTESIAN_POINT('Ctrl Pts',(1.71447789751927,-1.,0.740795162032088));
#40601=CARTESIAN_POINT('Ctrl Pts',(1.70473309006121,-1.,0.736799665724771));
#40602=CARTESIAN_POINT('Ctrl Pts',(1.69326921975743,-1.,0.731963238697195));
#40603=CARTESIAN_POINT('Ctrl Pts',(1.67996158455503,-1.,0.726235967997433));
#40604=CARTESIAN_POINT('Ctrl Pts',(1.6647288055568,-1.,0.719585433804282));
#40605=CARTESIAN_POINT('Ctrl Pts',(1.64752408832016,-1.,0.711993139355394));
#40606=CARTESIAN_POINT('Ctrl Pts',(1.63216541664676,-1.,0.705159151988319));
#40607=CARTESIAN_POINT('Ctrl Pts',(1.61974673472612,-1.,0.699605146405088));
#40608=CARTESIAN_POINT('Ctrl Pts',(1.61106790958151,-1.,0.695712097881194));
#40609=CARTESIAN_POINT('Ctrl Pts',(1.60662857109684,-1.,0.693717979106306));
#40610=CARTESIAN_POINT('Origin',(0.,1.,0.));
#40611=CARTESIAN_POINT('',(-1.4,1.,1.71450551880629E-16));
#40612=CARTESIAN_POINT('',(-1.4,1.,1.71450551880629E-16));
#40613=CARTESIAN_POINT('Origin',(0.,1.,0.));
#40614=CARTESIAN_POINT('Ctrl Pts',(2.11275013067528,-1.,0.613422273260091));
#40615=CARTESIAN_POINT('Ctrl Pts',(2.11275013067528,1.,0.613422273260091));
#40616=CARTESIAN_POINT('Ctrl Pts',(2.11187554260142,-1.,0.61246736556225));
#40617=CARTESIAN_POINT('Ctrl Pts',(2.11187554260142,1.,0.61246736556225));
#40618=CARTESIAN_POINT('Ctrl Pts',(2.11012443807661,-1.,0.610560911691114));
#40619=CARTESIAN_POINT('Ctrl Pts',(2.11012443807661,1.,0.610560911691114));
#40620=CARTESIAN_POINT('Ctrl Pts',(2.10749199615859,-1.,0.607711315456826));
#40621=CARTESIAN_POINT('Ctrl Pts',(2.10749199615859,1.,0.607711315456826));
#40622=CARTESIAN_POINT('Ctrl Pts',(2.10397049887709,-1.,0.603932030738212));
#40623=CARTESIAN_POINT('Ctrl Pts',(2.10397049887709,1.,0.603932030738212));
#40624=CARTESIAN_POINT('Ctrl Pts',(2.09954930865331,-1.,0.599241616422144));
#40625=CARTESIAN_POINT('Ctrl Pts',(2.09954930865331,1.,0.599241616422144));
#40626=CARTESIAN_POINT('Ctrl Pts',(2.09510876220501,-1.,0.594585006052824));
#40627=CARTESIAN_POINT('Ctrl Pts',(2.09510876220501,1.,0.594585006052824));
#40628=CARTESIAN_POINT('Ctrl Pts',(2.09064881812053,-1.,0.58996236540319));
#40629=CARTESIAN_POINT('Ctrl Pts',(2.09064881812053,1.,0.58996236540319));
#40630=CARTESIAN_POINT('Ctrl Pts',(2.086169437277,-1.,0.585373918990895));
#40631=CARTESIAN_POINT('Ctrl Pts',(2.086169437277,1.,0.585373918990895));
#40632=CARTESIAN_POINT('Ctrl Pts',(2.08167059018138,-1.,0.580819952107257));
#40633=CARTESIAN_POINT('Ctrl Pts',(2.08167059018138,1.,0.580819952107257));
#40634=CARTESIAN_POINT('Ctrl Pts',(2.07715226767361,-1.,0.576300797416275));
#40635=CARTESIAN_POINT('Ctrl Pts',(2.07715226767361,1.,0.576300797416275));
#40636=CARTESIAN_POINT('Ctrl Pts',(2.07261449292757,-1.,0.571816823242411));
#40637=CARTESIAN_POINT('Ctrl Pts',(2.07261449292757,1.,0.571816823242411));
#40638=CARTESIAN_POINT('Ctrl Pts',(2.06805732997383,-1.,0.56736842118123));
#40639=CARTESIAN_POINT('Ctrl Pts',(2.06805732997383,1.,0.56736842118123));
#40640=CARTESIAN_POINT('Ctrl Pts',(2.06348090160697,-1.,0.562955993082574));
#40641=CARTESIAN_POINT('Ctrl Pts',(2.06348090160697,1.,0.562955993082574));
#40642=CARTESIAN_POINT('Ctrl Pts',(2.05888537756571,-1.,0.558579940185468));
#40643=CARTESIAN_POINT('Ctrl Pts',(2.05888537756571,1.,0.558579940185468));
#40644=CARTESIAN_POINT('Ctrl Pts',(2.05427091604482,-1.,0.55424065746411));
#40645=CARTESIAN_POINT('Ctrl Pts',(2.05427091604482,1.,0.55424065746411));
#40646=CARTESIAN_POINT('Ctrl Pts',(2.04963761077974,-1.,0.549938525150342));
#40647=CARTESIAN_POINT('Ctrl Pts',(2.04963761077974,1.,0.549938525150342));
#40648=CARTESIAN_POINT('Ctrl Pts',(2.0449854471456,-1.,0.545673903817349));
#40649=CARTESIAN_POINT('Ctrl Pts',(2.0449854471456,1.,0.545673903817349));
#40650=CARTESIAN_POINT('Ctrl Pts',(2.0403142269048,-1.,0.54144712061552));
#40651=CARTESIAN_POINT('Ctrl Pts',(2.0403142269048,1.,0.54144712061552));
#40652=CARTESIAN_POINT('Ctrl Pts',(2.03562362953993,-1.,0.537258489833135));
#40653=CARTESIAN_POINT('Ctrl Pts',(2.03562362953993,1.,0.537258489833135));
#40654=CARTESIAN_POINT('Ctrl Pts',(2.03091336214401,-1.,0.533108355132905));
#40655=CARTESIAN_POINT('Ctrl Pts',(2.03091336214401,1.,0.533108355132905));
#40656=CARTESIAN_POINT('Ctrl Pts',(2.02618329083289,-1.,0.528997127241911));
#40657=CARTESIAN_POINT('Ctrl Pts',(2.02618329083289,1.,0.528997127241911));
#40658=CARTESIAN_POINT('Ctrl Pts',(2.02143356304712,-1.,0.524925318333519));
#40659=CARTESIAN_POINT('Ctrl Pts',(2.02143356304712,1.,0.524925318333519));
#40660=CARTESIAN_POINT('Ctrl Pts',(2.01666477917305,-1.,0.520893590399429));
#40661=CARTESIAN_POINT('Ctrl Pts',(2.01666477917305,1.,0.520893590399429));
#40662=CARTESIAN_POINT('Ctrl Pts',(2.01187773939257,-1.,0.516902681728733));
#40663=CARTESIAN_POINT('Ctrl Pts',(2.01187773939257,1.,0.516902681728733));
#40664=CARTESIAN_POINT('Ctrl Pts',(2.00707309946955,-1.,0.512953306961814));
#40665=CARTESIAN_POINT('Ctrl Pts',(2.00707309946955,1.,0.512953306961814));
#40666=CARTESIAN_POINT('Ctrl Pts',(2.00225107134733,-1.,0.509046069886152));
#40667=CARTESIAN_POINT('Ctrl Pts',(2.00225107134733,1.,0.509046069886152));
#40668=CARTESIAN_POINT('Ctrl Pts',(1.99741107463567,-1.,0.505181361323011));
#40669=CARTESIAN_POINT('Ctrl Pts',(1.99741107463567,1.,0.505181361323011));
#40670=CARTESIAN_POINT('Ctrl Pts',(1.9925514912615,-1.,0.501359287727129));
#40671=CARTESIAN_POINT('Ctrl Pts',(1.9925514912615,1.,0.501359287727129));
#40672=CARTESIAN_POINT('Ctrl Pts',(1.98767044752929,-1.,0.497579909545564));
#40673=CARTESIAN_POINT('Ctrl Pts',(1.98767044752929,1.,0.497579909545564));
#40674=CARTESIAN_POINT('Ctrl Pts',(1.9827665876182,-1.,0.493843476541493));
#40675=CARTESIAN_POINT('Ctrl Pts',(1.9827665876182,1.,0.493843476541493));
#40676=CARTESIAN_POINT('Ctrl Pts',(1.97783973019229,-1.,0.490150627860955));
#40677=CARTESIAN_POINT('Ctrl Pts',(1.97783973019229,1.,0.490150627860955));
#40678=CARTESIAN_POINT('Ctrl Pts',(1.97289186263272,-1.,0.486502692907661));
#40679=CARTESIAN_POINT('Ctrl Pts',(1.97289186263272,1.,0.486502692907661));
#40680=CARTESIAN_POINT('Ctrl Pts',(1.96792703422358,-1.,0.482901662120687));
#40681=CARTESIAN_POINT('Ctrl Pts',(1.96792703422358,1.,0.482901662120687));
#40682=CARTESIAN_POINT('Ctrl Pts',(1.96294933055938,-1.,0.479349583074846));
#40683=CARTESIAN_POINT('Ctrl Pts',(1.96294933055938,1.,0.479349583074846));
#40684=CARTESIAN_POINT('Ctrl Pts',(1.95796111148175,-1.,0.475848034683172));
#40685=CARTESIAN_POINT('Ctrl Pts',(1.95796111148175,1.,0.475848034683172));
#40686=CARTESIAN_POINT('Ctrl Pts',(1.95296148278136,-1.,0.47239767226408));
#40687=CARTESIAN_POINT('Ctrl Pts',(1.95296148278136,1.,0.47239767226408));
#40688=CARTESIAN_POINT('Ctrl Pts',(1.94794381136524,-1.,0.468997482913158));
#40689=CARTESIAN_POINT('Ctrl Pts',(1.94794381136524,1.,0.468997482913158));
#40690=CARTESIAN_POINT('Ctrl Pts',(1.94289794196205,-1.,0.465645462026065));
#40691=CARTESIAN_POINT('Ctrl Pts',(1.94289794196205,1.,0.465645462026065));
#40692=CARTESIAN_POINT('Ctrl Pts',(1.93781486640834,-1.,0.462340031009087));
#40693=CARTESIAN_POINT('Ctrl Pts',(1.93781486640834,1.,0.462340031009087));
#40694=CARTESIAN_POINT('Ctrl Pts',(1.93269066517936,-1.,0.459081234547932));
#40695=CARTESIAN_POINT('Ctrl Pts',(1.93269066517936,1.,0.459081234547932));
#40696=CARTESIAN_POINT('Ctrl Pts',(1.92753067150461,-1.,0.455872005174336));
#40697=CARTESIAN_POINT('Ctrl Pts',(1.92753067150461,1.,0.455872005174336));
#40698=CARTESIAN_POINT('Ctrl Pts',(1.9223538064847,-1.,0.452719478359356));
#40699=CARTESIAN_POINT('Ctrl Pts',(1.9223538064847,1.,0.452719478359356));
#40700=CARTESIAN_POINT('Ctrl Pts',(1.91718342555717,-1.,0.449632260106572));
#40701=CARTESIAN_POINT('Ctrl Pts',(1.91718342555717,1.,0.449632260106572));
#40702=CARTESIAN_POINT('Ctrl Pts',(1.91203699981095,-1.,0.446617343485651));
#40703=CARTESIAN_POINT('Ctrl Pts',(1.91203699981095,1.,0.446617343485651));
#40704=CARTESIAN_POINT('Ctrl Pts',(1.90691756144906,-1.,0.443677556849171));
#40705=CARTESIAN_POINT('Ctrl Pts',(1.90691756144906,1.,0.443677556849171));
#40706=CARTESIAN_POINT('Ctrl Pts',(1.90180124389137,-1.,0.440807833704161));
#40707=CARTESIAN_POINT('Ctrl Pts',(1.90180124389137,1.,0.440807833704161));
#40708=CARTESIAN_POINT('Ctrl Pts',(1.89663648956549,-1.,0.437995003948443));
#40709=CARTESIAN_POINT('Ctrl Pts',(1.89663648956549,1.,0.437995003948443));
#40710=CARTESIAN_POINT('Ctrl Pts',(1.89136993975585,-1.,0.43522566096358));
#40711=CARTESIAN_POINT('Ctrl Pts',(1.89136993975585,1.,0.43522566096358));
#40712=CARTESIAN_POINT('Ctrl Pts',(1.88596913666828,-1.,0.432493038548833));
#40713=CARTESIAN_POINT('Ctrl Pts',(1.88596913666828,1.,0.432493038548833));
#40714=CARTESIAN_POINT('Ctrl Pts',(1.88044229001778,-1.,0.429803062482217));
#40715=CARTESIAN_POINT('Ctrl Pts',(1.88044229001778,1.,0.429803062482217));
#40716=CARTESIAN_POINT('Ctrl Pts',(1.87486989291333,-1.,0.427183828518743));
#40717=CARTESIAN_POINT('Ctrl Pts',(1.87486989291333,1.,0.427183828518743));
#40718=CARTESIAN_POINT('Ctrl Pts',(1.8693780394412,-1.,0.424678177290876));
#40719=CARTESIAN_POINT('Ctrl Pts',(1.8693780394412,1.,0.424678177290876));
#40720=CARTESIAN_POINT('Ctrl Pts',(1.86408083333863,-1.,0.422327307417885));
#40721=CARTESIAN_POINT('Ctrl Pts',(1.86408083333863,1.,0.422327307417885));
#40722=CARTESIAN_POINT('Ctrl Pts',(1.8590328109667,-1.,0.420157287975583));
#40723=CARTESIAN_POINT('Ctrl Pts',(1.8590328109667,1.,0.420157287975583));
#40724=CARTESIAN_POINT('Ctrl Pts',(1.8541763285645,-1.,0.418164129144046));
#40725=CARTESIAN_POINT('Ctrl Pts',(1.8541763285645,1.,0.418164129144046));
#40726=CARTESIAN_POINT('Ctrl Pts',(1.84929312930314,-1.,0.416300022039885));
#40727=CARTESIAN_POINT('Ctrl Pts',(1.84929312930314,1.,0.416300022039885));
#40728=CARTESIAN_POINT('Ctrl Pts',(1.84405757074218,-1.,0.414487438255542));
#40729=CARTESIAN_POINT('Ctrl Pts',(1.84405757074218,1.,0.414487438255542));
#40730=CARTESIAN_POINT('Ctrl Pts',(1.8380895347617,-1.,0.412633125322945));
#40731=CARTESIAN_POINT('Ctrl Pts',(1.8380895347617,1.,0.412633125322945));
#40732=CARTESIAN_POINT('Ctrl Pts',(1.83100408895047,-1.,0.410641256301276));
#40733=CARTESIAN_POINT('Ctrl Pts',(1.83100408895047,1.,0.410641256301276));
#40734=CARTESIAN_POINT('Ctrl Pts',(1.82247022677562,-1.,0.408428948106228));
#40735=CARTESIAN_POINT('Ctrl Pts',(1.82247022677562,1.,0.408428948106228));
#40736=CARTESIAN_POINT('Ctrl Pts',(1.81223801812013,-1.,0.405933518407176));
#40737=CARTESIAN_POINT('Ctrl Pts',(1.81223801812013,1.,0.405933518407176));
#40738=CARTESIAN_POINT('Ctrl Pts',(1.80012077173238,-1.,0.403107976163396));
#40739=CARTESIAN_POINT('Ctrl Pts',(1.80012077173238,1.,0.403107976163396));
#40740=CARTESIAN_POINT('Ctrl Pts',(1.78598826343754,-1.,0.399919403774156));
#40741=CARTESIAN_POINT('Ctrl Pts',(1.78598826343754,1.,0.399919403774156));
#40742=CARTESIAN_POINT('Ctrl Pts',(1.76975560043442,-1.,0.396346196110688));
#40743=CARTESIAN_POINT('Ctrl Pts',(1.76975560043442,1.,0.396346196110688));
#40744=CARTESIAN_POINT('Ctrl Pts',(1.75137405310193,-1.,0.392375812285396));
#40745=CARTESIAN_POINT('Ctrl Pts',(1.75137405310193,1.,0.392375812285396));
#40746=CARTESIAN_POINT('Ctrl Pts',(1.73493170972829,-1.,0.388877023502615));
#40747=CARTESIAN_POINT('Ctrl Pts',(1.73493170972829,1.,0.388877023502615));
#40748=CARTESIAN_POINT('Ctrl Pts',(1.72162022244582,-1.,0.386070790323281));
#40749=CARTESIAN_POINT('Ctrl Pts',(1.72162022244582,1.,0.386070790323281));
#40750=CARTESIAN_POINT('Ctrl Pts',(1.71231062891398,-1.,0.384119047314215));
#40751=CARTESIAN_POINT('Ctrl Pts',(1.71231062891398,1.,0.384119047314215));
#40752=CARTESIAN_POINT('Ctrl Pts',(1.7075470150345,-1.,0.383122945602004));
#40753=CARTESIAN_POINT('Ctrl Pts',(1.7075470150345,1.,0.383122945602004));
#40754=CARTESIAN_POINT('',(1.7075470150345,1.,0.383122945602004));
#40755=CARTESIAN_POINT('',(1.7075470150345,0.,0.383122945602005));
#40756=CARTESIAN_POINT('',(2.11275013067528,1.,0.613422273260091));
#40757=CARTESIAN_POINT('Ctrl Pts',(2.11275013067528,1.,0.613422273260091));
#40758=CARTESIAN_POINT('Ctrl Pts',(2.11187554260142,1.,0.61246736556225));
#40759=CARTESIAN_POINT('Ctrl Pts',(2.11012443807661,1.,0.610560911691114));
#40760=CARTESIAN_POINT('Ctrl Pts',(2.10749199615859,1.,0.607711315456826));
#40761=CARTESIAN_POINT('Ctrl Pts',(2.10397049887709,1.,0.603932030738212));
#40762=CARTESIAN_POINT('Ctrl Pts',(2.09954930865331,1.,0.599241616422144));
#40763=CARTESIAN_POINT('Ctrl Pts',(2.09510876220501,1.,0.594585006052824));
#40764=CARTESIAN_POINT('Ctrl Pts',(2.09064881812053,1.,0.58996236540319));
#40765=CARTESIAN_POINT('Ctrl Pts',(2.086169437277,1.,0.585373918990895));
#40766=CARTESIAN_POINT('Ctrl Pts',(2.08167059018138,1.,0.580819952107257));
#40767=CARTESIAN_POINT('Ctrl Pts',(2.07715226767361,1.,0.576300797416275));
#40768=CARTESIAN_POINT('Ctrl Pts',(2.07261449292757,1.,0.571816823242411));
#40769=CARTESIAN_POINT('Ctrl Pts',(2.06805732997383,1.,0.56736842118123));
#40770=CARTESIAN_POINT('Ctrl Pts',(2.06348090160697,1.,0.562955993082574));
#40771=CARTESIAN_POINT('Ctrl Pts',(2.05888537756571,1.,0.558579940185468));
#40772=CARTESIAN_POINT('Ctrl Pts',(2.05427091604482,1.,0.55424065746411));
#40773=CARTESIAN_POINT('Ctrl Pts',(2.04963761077974,1.,0.549938525150342));
#40774=CARTESIAN_POINT('Ctrl Pts',(2.0449854471456,1.,0.545673903817349));
#40775=CARTESIAN_POINT('Ctrl Pts',(2.0403142269048,1.,0.54144712061552));
#40776=CARTESIAN_POINT('Ctrl Pts',(2.03562362953993,1.,0.537258489833135));
#40777=CARTESIAN_POINT('Ctrl Pts',(2.03091336214401,1.,0.533108355132905));
#40778=CARTESIAN_POINT('Ctrl Pts',(2.02618329083289,1.,0.528997127241911));
#40779=CARTESIAN_POINT('Ctrl Pts',(2.02143356304712,1.,0.524925318333519));
#40780=CARTESIAN_POINT('Ctrl Pts',(2.01666477917305,1.,0.520893590399429));
#40781=CARTESIAN_POINT('Ctrl Pts',(2.01187773939257,1.,0.516902681728733));
#40782=CARTESIAN_POINT('Ctrl Pts',(2.00707309946955,1.,0.512953306961814));
#40783=CARTESIAN_POINT('Ctrl Pts',(2.00225107134733,1.,0.509046069886152));
#40784=CARTESIAN_POINT('Ctrl Pts',(1.99741107463567,1.,0.505181361323011));
#40785=CARTESIAN_POINT('Ctrl Pts',(1.9925514912615,1.,0.501359287727129));
#40786=CARTESIAN_POINT('Ctrl Pts',(1.98767044752929,1.,0.497579909545564));
#40787=CARTESIAN_POINT('Ctrl Pts',(1.9827665876182,1.,0.493843476541493));
#40788=CARTESIAN_POINT('Ctrl Pts',(1.97783973019229,1.,0.490150627860955));
#40789=CARTESIAN_POINT('Ctrl Pts',(1.97289186263272,1.,0.486502692907661));
#40790=CARTESIAN_POINT('Ctrl Pts',(1.96792703422358,1.,0.482901662120687));
#40791=CARTESIAN_POINT('Ctrl Pts',(1.96294933055938,1.,0.479349583074846));
#40792=CARTESIAN_POINT('Ctrl Pts',(1.95796111148175,1.,0.475848034683172));
#40793=CARTESIAN_POINT('Ctrl Pts',(1.95296148278136,1.,0.47239767226408));
#40794=CARTESIAN_POINT('Ctrl Pts',(1.94794381136524,1.,0.468997482913158));
#40795=CARTESIAN_POINT('Ctrl Pts',(1.94289794196205,1.,0.465645462026065));
#40796=CARTESIAN_POINT('Ctrl Pts',(1.93781486640834,1.,0.462340031009087));
#40797=CARTESIAN_POINT('Ctrl Pts',(1.93269066517936,1.,0.459081234547932));
#40798=CARTESIAN_POINT('Ctrl Pts',(1.92753067150461,1.,0.455872005174336));
#40799=CARTESIAN_POINT('Ctrl Pts',(1.9223538064847,1.,0.452719478359356));
#40800=CARTESIAN_POINT('Ctrl Pts',(1.91718342555717,1.,0.449632260106572));
#40801=CARTESIAN_POINT('Ctrl Pts',(1.91203699981095,1.,0.446617343485651));
#40802=CARTESIAN_POINT('Ctrl Pts',(1.90691756144906,1.,0.443677556849171));
#40803=CARTESIAN_POINT('Ctrl Pts',(1.90180124389137,1.,0.440807833704161));
#40804=CARTESIAN_POINT('Ctrl Pts',(1.89663648956549,1.,0.437995003948443));
#40805=CARTESIAN_POINT('Ctrl Pts',(1.89136993975585,1.,0.43522566096358));
#40806=CARTESIAN_POINT('Ctrl Pts',(1.88596913666828,1.,0.432493038548833));
#40807=CARTESIAN_POINT('Ctrl Pts',(1.88044229001778,1.,0.429803062482217));
#40808=CARTESIAN_POINT('Ctrl Pts',(1.87486989291333,1.,0.427183828518743));
#40809=CARTESIAN_POINT('Ctrl Pts',(1.8693780394412,1.,0.424678177290876));
#40810=CARTESIAN_POINT('Ctrl Pts',(1.86408083333863,1.,0.422327307417885));
#40811=CARTESIAN_POINT('Ctrl Pts',(1.8590328109667,1.,0.420157287975583));
#40812=CARTESIAN_POINT('Ctrl Pts',(1.8541763285645,1.,0.418164129144046));
#40813=CARTESIAN_POINT('Ctrl Pts',(1.84929312930314,1.,0.416300022039885));
#40814=CARTESIAN_POINT('Ctrl Pts',(1.84405757074218,1.,0.414487438255542));
#40815=CARTESIAN_POINT('Ctrl Pts',(1.8380895347617,1.,0.412633125322945));
#40816=CARTESIAN_POINT('Ctrl Pts',(1.83100408895047,1.,0.410641256301276));
#40817=CARTESIAN_POINT('Ctrl Pts',(1.82247022677562,1.,0.408428948106228));
#40818=CARTESIAN_POINT('Ctrl Pts',(1.81223801812013,1.,0.405933518407176));
#40819=CARTESIAN_POINT('Ctrl Pts',(1.80012077173238,1.,0.403107976163396));
#40820=CARTESIAN_POINT('Ctrl Pts',(1.78598826343754,1.,0.399919403774156));
#40821=CARTESIAN_POINT('Ctrl Pts',(1.76975560043442,1.,0.396346196110688));
#40822=CARTESIAN_POINT('Ctrl Pts',(1.75137405310193,1.,0.392375812285396));
#40823=CARTESIAN_POINT('Ctrl Pts',(1.73493170972829,1.,0.388877023502615));
#40824=CARTESIAN_POINT('Ctrl Pts',(1.72162022244582,1.,0.386070790323281));
#40825=CARTESIAN_POINT('Ctrl Pts',(1.71231062891398,1.,0.384119047314215));
#40826=CARTESIAN_POINT('Ctrl Pts',(1.7075470150345,1.,0.383122945602004));
#40827=CARTESIAN_POINT('',(2.11275013067528,0.,0.613422273260091));
#40828=CARTESIAN_POINT('Origin',(2.0698113262342,0.,0.745574324794401));
#40829=CARTESIAN_POINT('',(2.0698113262342,1.,0.745574324794401));
#40830=CARTESIAN_POINT('',(2.11275013067528,1.,0.613422273260091));
#40831=CARTESIAN_POINT('',(2.0698113262342,0.,0.745574324794401));
#40832=CARTESIAN_POINT('Ctrl Pts',(1.60662857109684,-1.,0.693717979106306));
#40833=CARTESIAN_POINT('Ctrl Pts',(1.60662857109684,1.,0.693717979106306));
#40834=CARTESIAN_POINT('Ctrl Pts',(1.61106790958151,-1.,0.695712097881194));
#40835=CARTESIAN_POINT('Ctrl Pts',(1.61106790958151,1.,0.695712097881194));
#40836=CARTESIAN_POINT('Ctrl Pts',(1.61974673472612,-1.,0.699605146405088));
#40837=CARTESIAN_POINT('Ctrl Pts',(1.61974673472612,1.,0.699605146405088));
#40838=CARTESIAN_POINT('Ctrl Pts',(1.63216541664676,-1.,0.705159151988319));
#40839=CARTESIAN_POINT('Ctrl Pts',(1.63216541664676,1.,0.705159151988319));
#40840=CARTESIAN_POINT('Ctrl Pts',(1.64752408832016,-1.,0.711993139355394));
#40841=CARTESIAN_POINT('Ctrl Pts',(1.64752408832016,1.,0.711993139355394));
#40842=CARTESIAN_POINT('Ctrl Pts',(1.6647288055568,-1.,0.719585433804282));
#40843=CARTESIAN_POINT('Ctrl Pts',(1.6647288055568,1.,0.719585433804282));
#40844=CARTESIAN_POINT('Ctrl Pts',(1.67996158455503,-1.,0.726235967997433));
#40845=CARTESIAN_POINT('Ctrl Pts',(1.67996158455503,1.,0.726235967997433));
#40846=CARTESIAN_POINT('Ctrl Pts',(1.69326921975743,-1.,0.731963238697195));
#40847=CARTESIAN_POINT('Ctrl Pts',(1.69326921975743,1.,0.731963238697195));
#40848=CARTESIAN_POINT('Ctrl Pts',(1.70473309006121,-1.,0.736799665724771));
#40849=CARTESIAN_POINT('Ctrl Pts',(1.70473309006121,1.,0.736799665724771));
#40850=CARTESIAN_POINT('Ctrl Pts',(1.71447789751927,-1.,0.740795162032088));
#40851=CARTESIAN_POINT('Ctrl Pts',(1.71447789751927,1.,0.740795162032088));
#40852=CARTESIAN_POINT('Ctrl Pts',(1.7226822991693,-1.,0.744021445433765));
#40853=CARTESIAN_POINT('Ctrl Pts',(1.7226822991693,1.,0.744021445433765));
#40854=CARTESIAN_POINT('Ctrl Pts',(1.72958533647399,-1.,0.746574710096437));
#40855=CARTESIAN_POINT('Ctrl Pts',(1.72958533647399,1.,0.746574710096437));
#40856=CARTESIAN_POINT('Ctrl Pts',(1.73550351679848,-1.,0.748582462954855));
#40857=CARTESIAN_POINT('Ctrl Pts',(1.73550351679848,1.,0.748582462954855));
#40858=CARTESIAN_POINT('Ctrl Pts',(1.74080458266705,-1.,0.750193435979541));
#40859=CARTESIAN_POINT('Ctrl Pts',(1.74080458266705,1.,0.750193435979541));
#40860=CARTESIAN_POINT('Ctrl Pts',(1.74585086852298,-1.,0.751555614163629));
#40861=CARTESIAN_POINT('Ctrl Pts',(1.74585086852298,1.,0.751555614163629));
#40862=CARTESIAN_POINT('Ctrl Pts',(1.75095139468809,-1.,0.752797683531377));
#40863=CARTESIAN_POINT('Ctrl Pts',(1.75095139468809,1.,0.752797683531377));
#40864=CARTESIAN_POINT('Ctrl Pts',(1.75631083600175,-1.,0.75400925402848));
#40865=CARTESIAN_POINT('Ctrl Pts',(1.75631083600175,1.,0.75400925402848));
#40866=CARTESIAN_POINT('Ctrl Pts',(1.7619781724032,-1.,0.755220979975262));
#40867=CARTESIAN_POINT('Ctrl Pts',(1.7619781724032,1.,0.755220979975262));
#40868=CARTESIAN_POINT('Ctrl Pts',(1.76789396003141,-1.,0.756421896028403));
#40869=CARTESIAN_POINT('Ctrl Pts',(1.76789396003141,1.,0.756421896028403));
#40870=CARTESIAN_POINT('Ctrl Pts',(1.77394167108342,-1.,0.757578264077238));
#40871=CARTESIAN_POINT('Ctrl Pts',(1.77394167108342,1.,0.757578264077238));
#40872=CARTESIAN_POINT('Ctrl Pts',(1.77999411220912,-1.,0.75865062667738));
#40873=CARTESIAN_POINT('Ctrl Pts',(1.77999411220912,1.,0.75865062667738));
#40874=CARTESIAN_POINT('Ctrl Pts',(1.78596964884526,-1.,0.759614401109868));
#40875=CARTESIAN_POINT('Ctrl Pts',(1.78596964884526,1.,0.759614401109868));
#40876=CARTESIAN_POINT('Ctrl Pts',(1.79185815610802,-1.,0.760469555880425));
#40877=CARTESIAN_POINT('Ctrl Pts',(1.79185815610802,1.,0.760469555880425));
#40878=CARTESIAN_POINT('Ctrl Pts',(1.79768986997735,-1.,0.761229695230359));
#40879=CARTESIAN_POINT('Ctrl Pts',(1.79768986997735,1.,0.761229695230359));
#40880=CARTESIAN_POINT('Ctrl Pts',(1.80351583877334,-1.,0.761915336443516));
#40881=CARTESIAN_POINT('Ctrl Pts',(1.80351583877334,1.,0.761915336443516));
#40882=CARTESIAN_POINT('Ctrl Pts',(1.80938551463989,-1.,0.762546129464036));
#40883=CARTESIAN_POINT('Ctrl Pts',(1.80938551463989,1.,0.762546129464036));
#40884=CARTESIAN_POINT('Ctrl Pts',(1.81532118405566,-1.,0.763132003836783));
#40885=CARTESIAN_POINT('Ctrl Pts',(1.81532118405566,1.,0.763132003836783));
#40886=CARTESIAN_POINT('Ctrl Pts',(1.82131873145297,-1.,0.763673465462854));
#40887=CARTESIAN_POINT('Ctrl Pts',(1.82131873145297,1.,0.763673465462854));
#40888=CARTESIAN_POINT('Ctrl Pts',(1.8273599120008,-1.,0.764165902606056));
#40889=CARTESIAN_POINT('Ctrl Pts',(1.8273599120008,1.,0.764165902606056));
#40890=CARTESIAN_POINT('Ctrl Pts',(1.8334207722714,-1.,0.764602549687846));
#40891=CARTESIAN_POINT('Ctrl Pts',(1.8334207722714,1.,0.764602549687846));
#40892=CARTESIAN_POINT('Ctrl Pts',(1.83948181064823,-1.,0.764978057881688));
#40893=CARTESIAN_POINT('Ctrl Pts',(1.83948181064823,1.,0.764978057881688));
#40894=CARTESIAN_POINT('Ctrl Pts',(1.8455369887591,-1.,0.765291664861972));
#40895=CARTESIAN_POINT('Ctrl Pts',(1.8455369887591,1.,0.765291664861972));
#40896=CARTESIAN_POINT('Ctrl Pts',(1.85158945130054,-1.,0.765545710619023));
#40897=CARTESIAN_POINT('Ctrl Pts',(1.85158945130054,1.,0.765545710619023));
#40898=CARTESIAN_POINT('Ctrl Pts',(1.85764741390391,-1.,0.765744212909305));
#40899=CARTESIAN_POINT('Ctrl Pts',(1.85764741390391,1.,0.765744212909305));
#40900=CARTESIAN_POINT('Ctrl Pts',(1.86372027063314,-1.,0.765891519092557));
#40901=CARTESIAN_POINT('Ctrl Pts',(1.86372027063314,1.,0.765891519092557));
#40902=CARTESIAN_POINT('Ctrl Pts',(1.86981398314345,-1.,0.765990708546112));
#40903=CARTESIAN_POINT('Ctrl Pts',(1.86981398314345,1.,0.765990708546112));
#40904=CARTESIAN_POINT('Ctrl Pts',(1.87592888967886,-1.,0.766042837036759));
#40905=CARTESIAN_POINT('Ctrl Pts',(1.87592888967886,1.,0.766042837036759));
#40906=CARTESIAN_POINT('Ctrl Pts',(1.88206215302561,-1.,0.766047794851869));
#40907=CARTESIAN_POINT('Ctrl Pts',(1.88206215302561,1.,0.766047794851869));
#40908=CARTESIAN_POINT('Ctrl Pts',(1.88820926433409,-1.,0.76600483706209));
#40909=CARTESIAN_POINT('Ctrl Pts',(1.88820926433409,1.,0.76600483706209));
#40910=CARTESIAN_POINT('Ctrl Pts',(1.89436577771389,-1.,0.765913193856979));
#40911=CARTESIAN_POINT('Ctrl Pts',(1.89436577771389,1.,0.765913193856979));
#40912=CARTESIAN_POINT('Ctrl Pts',(1.90052930393599,-1.,0.765772772593395));
#40913=CARTESIAN_POINT('Ctrl Pts',(1.90052930393599,1.,0.765772772593395));
#40914=CARTESIAN_POINT('Ctrl Pts',(1.90669961402362,-1.,0.765584196937937));
#40915=CARTESIAN_POINT('Ctrl Pts',(1.90669961402362,1.,0.765584196937937));
#40916=CARTESIAN_POINT('Ctrl Pts',(1.91287765805174,-1.,0.765348465884739));
#40917=CARTESIAN_POINT('Ctrl Pts',(1.91287765805174,1.,0.765348465884739));
#40918=CARTESIAN_POINT('Ctrl Pts',(1.91906491634197,-1.,0.765066729667095));
#40919=CARTESIAN_POINT('Ctrl Pts',(1.91906491634197,1.,0.765066729667095));
#40920=CARTESIAN_POINT('Ctrl Pts',(1.92526263537041,-1.,0.764740025488189));
#40921=CARTESIAN_POINT('Ctrl Pts',(1.92526263537041,1.,0.764740025488189));
#40922=CARTESIAN_POINT('Ctrl Pts',(1.93147105496367,-1.,0.76436901067389));
#40923=CARTESIAN_POINT('Ctrl Pts',(1.93147105496367,1.,0.76436901067389));
#40924=CARTESIAN_POINT('Ctrl Pts',(1.93768964875867,-1.,0.763954049121394));
#40925=CARTESIAN_POINT('Ctrl Pts',(1.93768964875867,1.,0.763954049121394));
#40926=CARTESIAN_POINT('Ctrl Pts',(1.94391746617626,-1.,0.763495333538581));
#40927=CARTESIAN_POINT('Ctrl Pts',(1.94391746617626,1.,0.763495333538581));
#40928=CARTESIAN_POINT('Ctrl Pts',(1.95015342590025,-1.,0.762992990878774));
#40929=CARTESIAN_POINT('Ctrl Pts',(1.95015342590025,1.,0.762992990878774));
#40930=CARTESIAN_POINT('Ctrl Pts',(1.95639665309893,-1.,0.762447203806264));
#40931=CARTESIAN_POINT('Ctrl Pts',(1.95639665309893,1.,0.762447203806264));
#40932=CARTESIAN_POINT('Ctrl Pts',(1.96264672744229,-1.,0.761858300014575));
#40933=CARTESIAN_POINT('Ctrl Pts',(1.96264672744229,1.,0.761858300014575));
#40934=CARTESIAN_POINT('Ctrl Pts',(1.96890351582545,-1.,0.761226690483986));
#40935=CARTESIAN_POINT('Ctrl Pts',(1.96890351582545,1.,0.761226690483986));
#40936=CARTESIAN_POINT('Ctrl Pts',(1.97516705321521,-1.,0.760552825409856));
#40937=CARTESIAN_POINT('Ctrl Pts',(1.97516705321521,1.,0.760552825409856));
#40938=CARTESIAN_POINT('Ctrl Pts',(1.98143741418156,-1.,0.759837147452135));
#40939=CARTESIAN_POINT('Ctrl Pts',(1.98143741418156,1.,0.759837147452135));
#40940=CARTESIAN_POINT('Ctrl Pts',(1.98771456680806,-1.,0.759080037802243));
#40941=CARTESIAN_POINT('Ctrl Pts',(1.98771456680806,1.,0.759080037802243));
#40942=CARTESIAN_POINT('Ctrl Pts',(1.9939983109871,-1.,0.758281796766377));
#40943=CARTESIAN_POINT('Ctrl Pts',(1.9939983109871,1.,0.758281796766377));
#40944=CARTESIAN_POINT('Ctrl Pts',(2.00028834739072,-1.,0.757442676862342));
#40945=CARTESIAN_POINT('Ctrl Pts',(2.00028834739072,1.,0.757442676862342));
#40946=CARTESIAN_POINT('Ctrl Pts',(2.00658431587682,-1.,0.756562904646496));
#40947=CARTESIAN_POINT('Ctrl Pts',(2.00658431587682,1.,0.756562904646496));
#40948=CARTESIAN_POINT('Ctrl Pts',(2.01288584328149,-1.,0.755642704958101));
#40949=CARTESIAN_POINT('Ctrl Pts',(2.01288584328149,1.,0.755642704958101));
#40950=CARTESIAN_POINT('Ctrl Pts',(2.01919259406003,-1.,0.75468233072352));
#40951=CARTESIAN_POINT('Ctrl Pts',(2.01919259406003,1.,0.75468233072352));
#40952=CARTESIAN_POINT('Ctrl Pts',(2.02550428623587,-1.,0.753682061113766));
#40953=CARTESIAN_POINT('Ctrl Pts',(2.02550428623587,1.,0.753682061113766));
#40954=CARTESIAN_POINT('Ctrl Pts',(2.03182068456467,-1.,0.752642180488104));
#40955=CARTESIAN_POINT('Ctrl Pts',(2.03182068456467,1.,0.752642180488104));
#40956=CARTESIAN_POINT('Ctrl Pts',(2.03814160092173,-1.,0.751562963361384));
#40957=CARTESIAN_POINT('Ctrl Pts',(2.03814160092173,1.,0.751562963361384));
#40958=CARTESIAN_POINT('Ctrl Pts',(2.04446689147754,-1.,0.750444657874758));
#40959=CARTESIAN_POINT('Ctrl Pts',(2.04446689147754,1.,0.750444657874758));
#40960=CARTESIAN_POINT('Ctrl Pts',(2.05079645591606,-1.,0.749287468663053));
#40961=CARTESIAN_POINT('Ctrl Pts',(2.05079645591606,1.,0.749287468663053));
#40962=CARTESIAN_POINT('Ctrl Pts',(2.05713023030263,-1.,0.748091554181101));
#40963=CARTESIAN_POINT('Ctrl Pts',(2.05713023030263,1.,0.748091554181101));
#40964=CARTESIAN_POINT('Ctrl Pts',(2.06220058927162,-1.,0.747103932785504));
#40965=CARTESIAN_POINT('Ctrl Pts',(2.06220058927162,1.,0.747103932785504));
#40966=CARTESIAN_POINT('Ctrl Pts',(2.06600523016401,-1.,0.746345871542696));
#40967=CARTESIAN_POINT('Ctrl Pts',(2.06600523016401,1.,0.746345871542696));
#40968=CARTESIAN_POINT('Ctrl Pts',(2.06854248895575,-1.,0.74583279137781));
#40969=CARTESIAN_POINT('Ctrl Pts',(2.06854248895575,1.,0.74583279137781));
#40970=CARTESIAN_POINT('Ctrl Pts',(2.0698113262342,-1.,0.745574324794401));
#40971=CARTESIAN_POINT('Ctrl Pts',(2.0698113262342,1.,0.745574324794401));
#40972=CARTESIAN_POINT('',(1.60662857109684,1.,0.693717979106306));
#40973=CARTESIAN_POINT('Ctrl Pts',(1.60662857109684,1.,0.693717979106306));
#40974=CARTESIAN_POINT('Ctrl Pts',(1.61106790958151,1.,0.695712097881194));
#40975=CARTESIAN_POINT('Ctrl Pts',(1.61974673472612,1.,0.699605146405088));
#40976=CARTESIAN_POINT('Ctrl Pts',(1.63216541664676,1.,0.705159151988319));
#40977=CARTESIAN_POINT('Ctrl Pts',(1.64752408832016,1.,0.711993139355394));
#40978=CARTESIAN_POINT('Ctrl Pts',(1.6647288055568,1.,0.719585433804282));
#40979=CARTESIAN_POINT('Ctrl Pts',(1.67996158455503,1.,0.726235967997433));
#40980=CARTESIAN_POINT('Ctrl Pts',(1.69326921975743,1.,0.731963238697195));
#40981=CARTESIAN_POINT('Ctrl Pts',(1.70473309006121,1.,0.736799665724771));
#40982=CARTESIAN_POINT('Ctrl Pts',(1.71447789751927,1.,0.740795162032088));
#40983=CARTESIAN_POINT('Ctrl Pts',(1.7226822991693,1.,0.744021445433765));
#40984=CARTESIAN_POINT('Ctrl Pts',(1.72958533647399,1.,0.746574710096437));
#40985=CARTESIAN_POINT('Ctrl Pts',(1.73550351679848,1.,0.748582462954855));
#40986=CARTESIAN_POINT('Ctrl Pts',(1.74080458266705,1.,0.750193435979541));
#40987=CARTESIAN_POINT('Ctrl Pts',(1.74585086852298,1.,0.751555614163629));
#40988=CARTESIAN_POINT('Ctrl Pts',(1.75095139468809,1.,0.752797683531377));
#40989=CARTESIAN_POINT('Ctrl Pts',(1.75631083600175,1.,0.75400925402848));
#40990=CARTESIAN_POINT('Ctrl Pts',(1.7619781724032,1.,0.755220979975262));
#40991=CARTESIAN_POINT('Ctrl Pts',(1.76789396003141,1.,0.756421896028403));
#40992=CARTESIAN_POINT('Ctrl Pts',(1.77394167108342,1.,0.757578264077238));
#40993=CARTESIAN_POINT('Ctrl Pts',(1.77999411220912,1.,0.75865062667738));
#40994=CARTESIAN_POINT('Ctrl Pts',(1.78596964884526,1.,0.759614401109868));
#40995=CARTESIAN_POINT('Ctrl Pts',(1.79185815610802,1.,0.760469555880425));
#40996=CARTESIAN_POINT('Ctrl Pts',(1.79768986997735,1.,0.761229695230359));
#40997=CARTESIAN_POINT('Ctrl Pts',(1.80351583877334,1.,0.761915336443516));
#40998=CARTESIAN_POINT('Ctrl Pts',(1.80938551463989,1.,0.762546129464036));
#40999=CARTESIAN_POINT('Ctrl Pts',(1.81532118405566,1.,0.763132003836783));
#41000=CARTESIAN_POINT('Ctrl Pts',(1.82131873145297,1.,0.763673465462854));
#41001=CARTESIAN_POINT('Ctrl Pts',(1.8273599120008,1.,0.764165902606056));
#41002=CARTESIAN_POINT('Ctrl Pts',(1.8334207722714,1.,0.764602549687846));
#41003=CARTESIAN_POINT('Ctrl Pts',(1.83948181064823,1.,0.764978057881688));
#41004=CARTESIAN_POINT('Ctrl Pts',(1.8455369887591,1.,0.765291664861972));
#41005=CARTESIAN_POINT('Ctrl Pts',(1.85158945130054,1.,0.765545710619023));
#41006=CARTESIAN_POINT('Ctrl Pts',(1.85764741390391,1.,0.765744212909305));
#41007=CARTESIAN_POINT('Ctrl Pts',(1.86372027063314,1.,0.765891519092557));
#41008=CARTESIAN_POINT('Ctrl Pts',(1.86981398314345,1.,0.765990708546112));
#41009=CARTESIAN_POINT('Ctrl Pts',(1.87592888967886,1.,0.766042837036759));
#41010=CARTESIAN_POINT('Ctrl Pts',(1.88206215302561,1.,0.766047794851869));
#41011=CARTESIAN_POINT('Ctrl Pts',(1.88820926433409,1.,0.76600483706209));
#41012=CARTESIAN_POINT('Ctrl Pts',(1.89436577771389,1.,0.765913193856979));
#41013=CARTESIAN_POINT('Ctrl Pts',(1.90052930393599,1.,0.765772772593395));
#41014=CARTESIAN_POINT('Ctrl Pts',(1.90669961402362,1.,0.765584196937937));
#41015=CARTESIAN_POINT('Ctrl Pts',(1.91287765805174,1.,0.765348465884739));
#41016=CARTESIAN_POINT('Ctrl Pts',(1.91906491634197,1.,0.765066729667095));
#41017=CARTESIAN_POINT('Ctrl Pts',(1.92526263537041,1.,0.764740025488189));
#41018=CARTESIAN_POINT('Ctrl Pts',(1.93147105496367,1.,0.76436901067389));
#41019=CARTESIAN_POINT('Ctrl Pts',(1.93768964875867,1.,0.763954049121394));
#41020=CARTESIAN_POINT('Ctrl Pts',(1.94391746617626,1.,0.763495333538581));
#41021=CARTESIAN_POINT('Ctrl Pts',(1.95015342590025,1.,0.762992990878774));
#41022=CARTESIAN_POINT('Ctrl Pts',(1.95639665309893,1.,0.762447203806264));
#41023=CARTESIAN_POINT('Ctrl Pts',(1.96264672744229,1.,0.761858300014575));
#41024=CARTESIAN_POINT('Ctrl Pts',(1.96890351582545,1.,0.761226690483986));
#41025=CARTESIAN_POINT('Ctrl Pts',(1.97516705321521,1.,0.760552825409856));
#41026=CARTESIAN_POINT('Ctrl Pts',(1.98143741418156,1.,0.759837147452135));
#41027=CARTESIAN_POINT('Ctrl Pts',(1.98771456680806,1.,0.759080037802243));
#41028=CARTESIAN_POINT('Ctrl Pts',(1.9939983109871,1.,0.758281796766377));
#41029=CARTESIAN_POINT('Ctrl Pts',(2.00028834739072,1.,0.757442676862342));
#41030=CARTESIAN_POINT('Ctrl Pts',(2.00658431587682,1.,0.756562904646496));
#41031=CARTESIAN_POINT('Ctrl Pts',(2.01288584328149,1.,0.755642704958101));
#41032=CARTESIAN_POINT('Ctrl Pts',(2.01919259406003,1.,0.75468233072352));
#41033=CARTESIAN_POINT('Ctrl Pts',(2.02550428623587,1.,0.753682061113766));
#41034=CARTESIAN_POINT('Ctrl Pts',(2.03182068456467,1.,0.752642180488104));
#41035=CARTESIAN_POINT('Ctrl Pts',(2.03814160092173,1.,0.751562963361384));
#41036=CARTESIAN_POINT('Ctrl Pts',(2.04446689147754,1.,0.750444657874758));
#41037=CARTESIAN_POINT('Ctrl Pts',(2.05079645591606,1.,0.749287468663053));
#41038=CARTESIAN_POINT('Ctrl Pts',(2.05713023030263,1.,0.748091554181101));
#41039=CARTESIAN_POINT('Ctrl Pts',(2.06220058927162,1.,0.747103932785504));
#41040=CARTESIAN_POINT('Ctrl Pts',(2.06600523016401,1.,0.746345871542696));
#41041=CARTESIAN_POINT('Ctrl Pts',(2.06854248895575,1.,0.74583279137781));
#41042=CARTESIAN_POINT('Ctrl Pts',(2.0698113262342,1.,0.745574324794401));
#41043=CARTESIAN_POINT('',(1.60662857109684,0.,0.693717979106305));
#41044=CARTESIAN_POINT('Origin',(0.,0.,0.));
#41045=CARTESIAN_POINT('',(1.5055822144029,1.,0.892032620296856));
#41046=CARTESIAN_POINT('Origin',(0.,1.,0.));
#41047=CARTESIAN_POINT('',(1.5055822144029,0.,0.892032620296855));
#41048=CARTESIAN_POINT('Ctrl Pts',(1.81978687191668,-1.,1.23627494547115));
#41049=CARTESIAN_POINT('Ctrl Pts',(1.81978687191668,1.,1.23627494547115));
#41050=CARTESIAN_POINT('Ctrl Pts',(1.81925017193666,-1.,1.23509651170476));
#41051=CARTESIAN_POINT('Ctrl Pts',(1.81925017193666,1.,1.23509651170476));
#41052=CARTESIAN_POINT('Ctrl Pts',(1.81817389921279,-1.,1.2327422452705));
#41053=CARTESIAN_POINT('Ctrl Pts',(1.81817389921279,1.,1.2327422452705));
#41054=CARTESIAN_POINT('Ctrl Pts',(1.8165508718364,-1.,1.2292186489137));
#41055=CARTESIAN_POINT('Ctrl Pts',(1.8165508718364,1.,1.2292186489137));
#41056=CARTESIAN_POINT('Ctrl Pts',(1.81436959210434,-1.,1.2245361330495));
#41057=CARTESIAN_POINT('Ctrl Pts',(1.81436959210434,1.,1.2245361330495));
#41058=CARTESIAN_POINT('Ctrl Pts',(1.81161420806656,-1.,1.21870906103557));
#41059=CARTESIAN_POINT('Ctrl Pts',(1.81161420806656,1.,1.21870906103557));
#41060=CARTESIAN_POINT('Ctrl Pts',(1.80882996917129,-1.,1.21290815708314));
#41061=CARTESIAN_POINT('Ctrl Pts',(1.80882996917129,1.,1.21290815708314));
#41062=CARTESIAN_POINT('Ctrl Pts',(1.80601678480707,-1.,1.20713356605475));
#41063=CARTESIAN_POINT('Ctrl Pts',(1.80601678480707,1.,1.20713356605475));
#41064=CARTESIAN_POINT('Ctrl Pts',(1.80317454838603,-1.,1.20138548938974));
#41065=CARTESIAN_POINT('Ctrl Pts',(1.80317454838603,1.,1.20138548938974));
#41066=CARTESIAN_POINT('Ctrl Pts',(1.80030314369879,-1.,1.19566418930242));
#41067=CARTESIAN_POINT('Ctrl Pts',(1.80030314369879,1.,1.19566418930242));
#41068=CARTESIAN_POINT('Ctrl Pts',(1.79740245923478,-1.,1.18996997934445));
#41069=CARTESIAN_POINT('Ctrl Pts',(1.79740245923478,1.,1.18996997934445));
#41070=CARTESIAN_POINT('Ctrl Pts',(1.79447240321515,-1.,1.18430321697432));
#41071=CARTESIAN_POINT('Ctrl Pts',(1.79447240321515,1.,1.18430321697432));
#41072=CARTESIAN_POINT('Ctrl Pts',(1.79151291552689,-1.,1.17866429440809));
#41073=CARTESIAN_POINT('Ctrl Pts',(1.79151291552689,1.,1.17866429440809));
#41074=CARTESIAN_POINT('Ctrl Pts',(1.78852398877616,-1.,1.17305363177328));
#41075=CARTESIAN_POINT('Ctrl Pts',(1.78852398877616,1.,1.17305363177328));
#41076=CARTESIAN_POINT('Ctrl Pts',(1.78550566040443,-1.,1.16747166312303));
#41077=CARTESIAN_POINT('Ctrl Pts',(1.78550566040443,1.,1.16747166312303));
#41078=CARTESIAN_POINT('Ctrl Pts',(1.78245795881009,-1.,1.16191881298499));
#41079=CARTESIAN_POINT('Ctrl Pts',(1.78245795881009,1.,1.16191881298499));
#41080=CARTESIAN_POINT('Ctrl Pts',(1.77938085564275,-1.,1.15639547194698));
#41081=CARTESIAN_POINT('Ctrl Pts',(1.77938085564275,1.,1.15639547194698));
#41082=CARTESIAN_POINT('Ctrl Pts',(1.7762742255701,-1.,1.15090197841515));
#41083=CARTESIAN_POINT('Ctrl Pts',(1.7762742255701,1.,1.15090197841515));
#41084=CARTESIAN_POINT('Ctrl Pts',(1.77313777896194,-1.,1.1454385822692));
#41085=CARTESIAN_POINT('Ctrl Pts',(1.77313777896194,1.,1.1454385822692));
#41086=CARTESIAN_POINT('Ctrl Pts',(1.76997111386769,-1.,1.14000548336975));
#41087=CARTESIAN_POINT('Ctrl Pts',(1.76997111386769,1.,1.14000548336975));
#41088=CARTESIAN_POINT('Ctrl Pts',(1.76677384551862,-1.,1.1346029180462));
#41089=CARTESIAN_POINT('Ctrl Pts',(1.76677384551862,1.,1.1346029180462));
#41090=CARTESIAN_POINT('Ctrl Pts',(1.7635457196617,-1.,1.12923123555075));
#41091=CARTESIAN_POINT('Ctrl Pts',(1.7635457196617,1.,1.12923123555075));
#41092=CARTESIAN_POINT('Ctrl Pts',(1.76028671825096,-1.,1.12389096855086));
#41093=CARTESIAN_POINT('Ctrl Pts',(1.76028671825096,1.,1.12389096855086));
#41094=CARTESIAN_POINT('Ctrl Pts',(1.75699720772105,-1.,1.11858293216763));
#41095=CARTESIAN_POINT('Ctrl Pts',(1.75699720772105,1.,1.11858293216763));
#41096=CARTESIAN_POINT('Ctrl Pts',(1.7536777209463,-1.,1.11330807582551));
#41097=CARTESIAN_POINT('Ctrl Pts',(1.7536777209463,1.,1.11330807582551));
#41098=CARTESIAN_POINT('Ctrl Pts',(1.7503286607592,-1.,1.10806728183007));
#41099=CARTESIAN_POINT('Ctrl Pts',(1.7503286607592,1.,1.10806728183007));
#41100=CARTESIAN_POINT('Ctrl Pts',(1.74695004214923,-1.,1.10286118991143));
#41101=CARTESIAN_POINT('Ctrl Pts',(1.74695004214923,1.,1.10286118991143));
#41102=CARTESIAN_POINT('Ctrl Pts',(1.74354119236208,-1.,1.09768999241226));
#41103=CARTESIAN_POINT('Ctrl Pts',(1.74354119236208,1.,1.09768999241226));
#41104=CARTESIAN_POINT('Ctrl Pts',(1.74010053962247,-1.,1.09255329056493));
#41105=CARTESIAN_POINT('Ctrl Pts',(1.74010053962247,1.,1.09255329056493));
#41106=CARTESIAN_POINT('Ctrl Pts',(1.73662628326091,-1.,1.08745056285427));
#41107=CARTESIAN_POINT('Ctrl Pts',(1.73662628326091,1.,1.08745056285427));
#41108=CARTESIAN_POINT('Ctrl Pts',(1.73311705663407,-1.,1.08238162784749));
#41109=CARTESIAN_POINT('Ctrl Pts',(1.73311705663407,1.,1.08238162784749));
#41110=CARTESIAN_POINT('Ctrl Pts',(1.72957248977424,-1.,1.0773470373727));
#41111=CARTESIAN_POINT('Ctrl Pts',(1.72957248977424,1.,1.0773470373727));
#41112=CARTESIAN_POINT('Ctrl Pts',(1.72599406198488,-1.,1.07234866990252));
#41113=CARTESIAN_POINT('Ctrl Pts',(1.72599406198488,1.,1.07234866990252));
#41114=CARTESIAN_POINT('Ctrl Pts',(1.72238500928453,-1.,1.06738966975462));
#41115=CARTESIAN_POINT('Ctrl Pts',(1.72238500928453,1.,1.06738966975462));
#41116=CARTESIAN_POINT('Ctrl Pts',(1.71874858456904,-1.,1.06247324680647));
#41117=CARTESIAN_POINT('Ctrl Pts',(1.71874858456904,1.,1.06247324680647));
#41118=CARTESIAN_POINT('Ctrl Pts',(1.7150865442702,-1.,1.05760163192479));
#41119=CARTESIAN_POINT('Ctrl Pts',(1.7150865442702,1.,1.05760163192479));
#41120=CARTESIAN_POINT('Ctrl Pts',(1.71139783543989,-1.,1.05277517202855));
#41121=CARTESIAN_POINT('Ctrl Pts',(1.71139783543989,1.,1.05277517202855));
#41122=CARTESIAN_POINT('Ctrl Pts',(1.70767646263649,-1.,1.04799085404995));
#41123=CARTESIAN_POINT('Ctrl Pts',(1.70767646263649,1.,1.04799085404995));
#41124=CARTESIAN_POINT('Ctrl Pts',(1.70391338707982,-1.,1.04324363334554));
#41125=CARTESIAN_POINT('Ctrl Pts',(1.70391338707982,1.,1.04324363334554));
#41126=CARTESIAN_POINT('Ctrl Pts',(1.70010052930962,-1.,1.03852922490789));
#41127=CARTESIAN_POINT('Ctrl Pts',(1.70010052930962,1.,1.03852922490789));
#41128=CARTESIAN_POINT('Ctrl Pts',(1.69623414782771,-1.,1.03384646003588));
#41129=CARTESIAN_POINT('Ctrl Pts',(1.69623414782771,1.,1.03384646003588));
#41130=CARTESIAN_POINT('Ctrl Pts',(1.69231840863458,-1.,1.02919977579147));
#41131=CARTESIAN_POINT('Ctrl Pts',(1.69231840863458,1.,1.02919977579147));
#41132=CARTESIAN_POINT('Ctrl Pts',(1.68836910178447,-1.,1.02460180535255));
#41133=CARTESIAN_POINT('Ctrl Pts',(1.68836910178447,1.,1.02460180535255));
#41134=CARTESIAN_POINT('Ctrl Pts',(1.68440578021706,-1.,1.02006795074201));
#41135=CARTESIAN_POINT('Ctrl Pts',(1.68440578021706,1.,1.02006795074201));
#41136=CARTESIAN_POINT('Ctrl Pts',(1.68044289894798,-1.,1.01561026162773));
#41137=CARTESIAN_POINT('Ctrl Pts',(1.68044289894798,1.,1.01561026162773));
#41138=CARTESIAN_POINT('Ctrl Pts',(1.67648246776464,-1.,1.01123236493511));
#41139=CARTESIAN_POINT('Ctrl Pts',(1.67648246776464,1.,1.01123236493511));
#41140=CARTESIAN_POINT('Ctrl Pts',(1.67250335383293,-1.,1.00692206696414));
#41141=CARTESIAN_POINT('Ctrl Pts',(1.67250335383293,1.,1.00692206696414));
#41142=CARTESIAN_POINT('Ctrl Pts',(1.66846059277303,-1.,1.00265091003727));
#41143=CARTESIAN_POINT('Ctrl Pts',(1.66846059277303,1.,1.00265091003727));
#41144=CARTESIAN_POINT('Ctrl Pts',(1.66430758030376,-1.,0.998389654952758));
#41145=CARTESIAN_POINT('Ctrl Pts',(1.66430758030376,1.,0.998389654952758));
#41146=CARTESIAN_POINT('Ctrl Pts',(1.66001553809947,-1.,0.994121836661306));
#41147=CARTESIAN_POINT('Ctrl Pts',(1.66001553809947,1.,0.994121836661306));
#41148=CARTESIAN_POINT('Ctrl Pts',(1.65559044289699,-1.,0.989855627854165));
#41149=CARTESIAN_POINT('Ctrl Pts',(1.65559044289699,1.,0.989855627854165));
#41150=CARTESIAN_POINT('Ctrl Pts',(1.65110016612638,-1.,0.985642622920821));
#41151=CARTESIAN_POINT('Ctrl Pts',(1.65110016612638,1.,0.985642622920821));
#41152=CARTESIAN_POINT('Ctrl Pts',(1.64665139190656,-1.,0.981562530939489));
#41153=CARTESIAN_POINT('Ctrl Pts',(1.64665139190656,1.,0.981562530939489));
#41154=CARTESIAN_POINT('Ctrl Pts',(1.64233990826687,-1.,0.977689794119417));
#41155=CARTESIAN_POINT('Ctrl Pts',(1.64233990826687,1.,0.977689794119417));
#41156=CARTESIAN_POINT('Ctrl Pts',(1.63820952658144,-1.,0.974066058287419));
#41157=CARTESIAN_POINT('Ctrl Pts',(1.63820952658144,1.,0.974066058287419));
#41158=CARTESIAN_POINT('Ctrl Pts',(1.63420665729798,-1.,0.970669715997509));
#41159=CARTESIAN_POINT('Ctrl Pts',(1.63420665729798,1.,0.970669715997509));
#41160=CARTESIAN_POINT('Ctrl Pts',(1.63013849959461,-1.,0.967387853230345));
#41161=CARTESIAN_POINT('Ctrl Pts',(1.63013849959461,1.,0.967387853230345));
#41162=CARTESIAN_POINT('Ctrl Pts',(1.62571930670187,-1.,0.964046107040536));
#41163=CARTESIAN_POINT('Ctrl Pts',(1.62571930670187,1.,0.964046107040536));
#41164=CARTESIAN_POINT('Ctrl Pts',(1.62061638140221,-1.,0.960438326101729));
#41165=CARTESIAN_POINT('Ctrl Pts',(1.62061638140221,1.,0.960438326101729));
#41166=CARTESIAN_POINT('Ctrl Pts',(1.61449324337085,-1.,0.956354422920671));
#41167=CARTESIAN_POINT('Ctrl Pts',(1.61449324337085,1.,0.956354422920671));
#41168=CARTESIAN_POINT('Ctrl Pts',(1.60706069896936,-1.,0.951613284356035));
#41169=CARTESIAN_POINT('Ctrl Pts',(1.60706069896936,1.,0.951613284356035));
#41170=CARTESIAN_POINT('Ctrl Pts',(1.59810042043673,-1.,0.946078063315257));
#41171=CARTESIAN_POINT('Ctrl Pts',(1.59810042043673,1.,0.946078063315257));
#41172=CARTESIAN_POINT('Ctrl Pts',(1.58744937487176,-1.,0.939646377893399));
#41173=CARTESIAN_POINT('Ctrl Pts',(1.58744937487176,1.,0.939646377893399));
#41174=CARTESIAN_POINT('Ctrl Pts',(1.57499388382243,-1.,0.932246680108685));
#41175=CARTESIAN_POINT('Ctrl Pts',(1.57499388382243,1.,0.932246680108685));
#41176=CARTESIAN_POINT('Ctrl Pts',(1.56065988578893,-1.,0.923832188944341));
#41177=CARTESIAN_POINT('Ctrl Pts',(1.56065988578893,1.,0.923832188944341));
#41178=CARTESIAN_POINT('Ctrl Pts',(1.54440491149498,-1.,0.914375919026456));
#41179=CARTESIAN_POINT('Ctrl Pts',(1.54440491149498,1.,0.914375919026456));
#41180=CARTESIAN_POINT('Ctrl Pts',(1.52984849887993,-1.,0.905967409625651));
#41181=CARTESIAN_POINT('Ctrl Pts',(1.52984849887993,1.,0.905967409625651));
#41182=CARTESIAN_POINT('Ctrl Pts',(1.51805569590094,-1.,0.899185047483511));
#41183=CARTESIAN_POINT('Ctrl Pts',(1.51805569590094,1.,0.899185047483511));
#41184=CARTESIAN_POINT('Ctrl Pts',(1.50980486806688,-1.,0.894452006964544));
#41185=CARTESIAN_POINT('Ctrl Pts',(1.50980486806688,1.,0.894452006964544));
#41186=CARTESIAN_POINT('Ctrl Pts',(1.5055822144029,-1.,0.892032620296856));
#41187=CARTESIAN_POINT('Ctrl Pts',(1.5055822144029,1.,0.892032620296856));
#41188=CARTESIAN_POINT('',(1.81978687191668,1.,1.23627494547115));
#41189=CARTESIAN_POINT('Ctrl Pts',(1.81978687191668,1.,1.23627494547115));
#41190=CARTESIAN_POINT('Ctrl Pts',(1.81925017193666,1.,1.23509651170476));
#41191=CARTESIAN_POINT('Ctrl Pts',(1.81817389921279,1.,1.2327422452705));
#41192=CARTESIAN_POINT('Ctrl Pts',(1.8165508718364,1.,1.2292186489137));
#41193=CARTESIAN_POINT('Ctrl Pts',(1.81436959210434,1.,1.2245361330495));
#41194=CARTESIAN_POINT('Ctrl Pts',(1.81161420806656,1.,1.21870906103557));
#41195=CARTESIAN_POINT('Ctrl Pts',(1.80882996917129,1.,1.21290815708314));
#41196=CARTESIAN_POINT('Ctrl Pts',(1.80601678480707,1.,1.20713356605475));
#41197=CARTESIAN_POINT('Ctrl Pts',(1.80317454838603,1.,1.20138548938974));
#41198=CARTESIAN_POINT('Ctrl Pts',(1.80030314369879,1.,1.19566418930242));
#41199=CARTESIAN_POINT('Ctrl Pts',(1.79740245923478,1.,1.18996997934445));
#41200=CARTESIAN_POINT('Ctrl Pts',(1.79447240321515,1.,1.18430321697432));
#41201=CARTESIAN_POINT('Ctrl Pts',(1.79151291552689,1.,1.17866429440809));
#41202=CARTESIAN_POINT('Ctrl Pts',(1.78852398877616,1.,1.17305363177328));
#41203=CARTESIAN_POINT('Ctrl Pts',(1.78550566040443,1.,1.16747166312303));
#41204=CARTESIAN_POINT('Ctrl Pts',(1.78245795881009,1.,1.16191881298499));
#41205=CARTESIAN_POINT('Ctrl Pts',(1.77938085564275,1.,1.15639547194698));
#41206=CARTESIAN_POINT('Ctrl Pts',(1.7762742255701,1.,1.15090197841515));
#41207=CARTESIAN_POINT('Ctrl Pts',(1.77313777896194,1.,1.1454385822692));
#41208=CARTESIAN_POINT('Ctrl Pts',(1.76997111386769,1.,1.14000548336975));
#41209=CARTESIAN_POINT('Ctrl Pts',(1.76677384551862,1.,1.1346029180462));
#41210=CARTESIAN_POINT('Ctrl Pts',(1.7635457196617,1.,1.12923123555075));
#41211=CARTESIAN_POINT('Ctrl Pts',(1.76028671825096,1.,1.12389096855086));
#41212=CARTESIAN_POINT('Ctrl Pts',(1.75699720772105,1.,1.11858293216763));
#41213=CARTESIAN_POINT('Ctrl Pts',(1.7536777209463,1.,1.11330807582551));
#41214=CARTESIAN_POINT('Ctrl Pts',(1.7503286607592,1.,1.10806728183007));
#41215=CARTESIAN_POINT('Ctrl Pts',(1.74695004214923,1.,1.10286118991143));
#41216=CARTESIAN_POINT('Ctrl Pts',(1.74354119236208,1.,1.09768999241226));
#41217=CARTESIAN_POINT('Ctrl Pts',(1.74010053962247,1.,1.09255329056493));
#41218=CARTESIAN_POINT('Ctrl Pts',(1.73662628326091,1.,1.08745056285427));
#41219=CARTESIAN_POINT('Ctrl Pts',(1.73311705663407,1.,1.08238162784749));
#41220=CARTESIAN_POINT('Ctrl Pts',(1.72957248977424,1.,1.0773470373727));
#41221=CARTESIAN_POINT('Ctrl Pts',(1.72599406198488,1.,1.07234866990252));
#41222=CARTESIAN_POINT('Ctrl Pts',(1.72238500928453,1.,1.06738966975462));
#41223=CARTESIAN_POINT('Ctrl Pts',(1.71874858456904,1.,1.06247324680647));
#41224=CARTESIAN_POINT('Ctrl Pts',(1.7150865442702,1.,1.05760163192479));
#41225=CARTESIAN_POINT('Ctrl Pts',(1.71139783543989,1.,1.05277517202855));
#41226=CARTESIAN_POINT('Ctrl Pts',(1.70767646263649,1.,1.04799085404995));
#41227=CARTESIAN_POINT('Ctrl Pts',(1.70391338707982,1.,1.04324363334554));
#41228=CARTESIAN_POINT('Ctrl Pts',(1.70010052930962,1.,1.03852922490789));
#41229=CARTESIAN_POINT('Ctrl Pts',(1.69623414782771,1.,1.03384646003588));
#41230=CARTESIAN_POINT('Ctrl Pts',(1.69231840863458,1.,1.02919977579147));
#41231=CARTESIAN_POINT('Ctrl Pts',(1.68836910178447,1.,1.02460180535255));
#41232=CARTESIAN_POINT('Ctrl Pts',(1.68440578021706,1.,1.02006795074201));
#41233=CARTESIAN_POINT('Ctrl Pts',(1.68044289894798,1.,1.01561026162773));
#41234=CARTESIAN_POINT('Ctrl Pts',(1.67648246776464,1.,1.01123236493511));
#41235=CARTESIAN_POINT('Ctrl Pts',(1.67250335383293,1.,1.00692206696414));
#41236=CARTESIAN_POINT('Ctrl Pts',(1.66846059277303,1.,1.00265091003727));
#41237=CARTESIAN_POINT('Ctrl Pts',(1.66430758030376,1.,0.998389654952758));
#41238=CARTESIAN_POINT('Ctrl Pts',(1.66001553809947,1.,0.994121836661306));
#41239=CARTESIAN_POINT('Ctrl Pts',(1.65559044289699,1.,0.989855627854165));
#41240=CARTESIAN_POINT('Ctrl Pts',(1.65110016612638,1.,0.985642622920821));
#41241=CARTESIAN_POINT('Ctrl Pts',(1.64665139190656,1.,0.981562530939489));
#41242=CARTESIAN_POINT('Ctrl Pts',(1.64233990826687,1.,0.977689794119417));
#41243=CARTESIAN_POINT('Ctrl Pts',(1.63820952658144,1.,0.974066058287419));
#41244=CARTESIAN_POINT('Ctrl Pts',(1.63420665729798,1.,0.970669715997509));
#41245=CARTESIAN_POINT('Ctrl Pts',(1.63013849959461,1.,0.967387853230345));
#41246=CARTESIAN_POINT('Ctrl Pts',(1.62571930670187,1.,0.964046107040536));
#41247=CARTESIAN_POINT('Ctrl Pts',(1.62061638140221,1.,0.960438326101729));
#41248=CARTESIAN_POINT('Ctrl Pts',(1.61449324337085,1.,0.956354422920671));
#41249=CARTESIAN_POINT('Ctrl Pts',(1.60706069896936,1.,0.951613284356035));
#41250=CARTESIAN_POINT('Ctrl Pts',(1.59810042043673,1.,0.946078063315257));
#41251=CARTESIAN_POINT('Ctrl Pts',(1.58744937487176,1.,0.939646377893399));
#41252=CARTESIAN_POINT('Ctrl Pts',(1.57499388382243,1.,0.932246680108685));
#41253=CARTESIAN_POINT('Ctrl Pts',(1.56065988578893,1.,0.923832188944341));
#41254=CARTESIAN_POINT('Ctrl Pts',(1.54440491149498,1.,0.914375919026456));
#41255=CARTESIAN_POINT('Ctrl Pts',(1.52984849887993,1.,0.905967409625651));
#41256=CARTESIAN_POINT('Ctrl Pts',(1.51805569590094,1.,0.899185047483511));
#41257=CARTESIAN_POINT('Ctrl Pts',(1.50980486806688,1.,0.894452006964544));
#41258=CARTESIAN_POINT('Ctrl Pts',(1.5055822144029,1.,0.892032620296856));
#41259=CARTESIAN_POINT('',(1.81978687191668,0.,1.23627494547115));
#41260=CARTESIAN_POINT('Origin',(1.73811241238545,0.,1.34869019493419));
#41261=CARTESIAN_POINT('',(1.73811241238545,1.,1.34869019493419));
#41262=CARTESIAN_POINT('',(1.81978687191668,1.,1.23627494547115));
#41263=CARTESIAN_POINT('',(1.73811241238545,0.,1.34869019493419));
#41264=CARTESIAN_POINT('Ctrl Pts',(1.31362392696032,-1.,1.15624053661742));
#41265=CARTESIAN_POINT('Ctrl Pts',(1.31362392696032,1.,1.15624053661742));
#41266=CARTESIAN_POINT('Ctrl Pts',(1.31722977216397,-1.,1.15950888730809));
#41267=CARTESIAN_POINT('Ctrl Pts',(1.31722977216397,1.,1.15950888730809));
#41268=CARTESIAN_POINT('Ctrl Pts',(1.32428080721772,-1.,1.16589330093588));
#41269=CARTESIAN_POINT('Ctrl Pts',(1.32428080721772,1.,1.16589330093588));
#41270=CARTESIAN_POINT('Ctrl Pts',(1.33437539347008,-1.,1.17501305789857));
#41271=CARTESIAN_POINT('Ctrl Pts',(1.33437539347008,1.,1.17501305789857));
#41272=CARTESIAN_POINT('Ctrl Pts',(1.34687054001093,-1.,1.18625865667441));
#41273=CARTESIAN_POINT('Ctrl Pts',(1.34687054001093,1.,1.18625865667441));
#41274=CARTESIAN_POINT('Ctrl Pts',(1.36088705043885,-1.,1.1987959077932));
#41275=CARTESIAN_POINT('Ctrl Pts',(1.36088705043885,1.,1.1987959077932));
#41276=CARTESIAN_POINT('Ctrl Pts',(1.37331915607905,-1.,1.20982812925645));
#41277=CARTESIAN_POINT('Ctrl Pts',(1.37331915607905,1.,1.20982812925645));
#41278=CARTESIAN_POINT('Ctrl Pts',(1.38420564527715,-1.,1.21938737280852));
#41279=CARTESIAN_POINT('Ctrl Pts',(1.38420564527715,1.,1.21938737280852));
#41280=CARTESIAN_POINT('Ctrl Pts',(1.39361389568796,-1.,1.22752961899387));
#41281=CARTESIAN_POINT('Ctrl Pts',(1.39361389568796,1.,1.22752961899387));
#41282=CARTESIAN_POINT('Ctrl Pts',(1.40164708206106,-1.,1.23434087290423));
#41283=CARTESIAN_POINT('Ctrl Pts',(1.40164708206106,1.,1.23434087290423));
#41284=CARTESIAN_POINT('Ctrl Pts',(1.40845295531283,-1.,1.23994455029534));
#41285=CARTESIAN_POINT('Ctrl Pts',(1.40845295531283,1.,1.23994455029534));
#41286=CARTESIAN_POINT('Ctrl Pts',(1.41422913175179,-1.,1.24450600513056));
#41287=CARTESIAN_POINT('Ctrl Pts',(1.41422913175179,1.,1.24450600513056));
#41288=CARTESIAN_POINT('Ctrl Pts',(1.41923722596025,-1.,1.24824430986571));
#41289=CARTESIAN_POINT('Ctrl Pts',(1.41923722596025,1.,1.24824430986571));
#41290=CARTESIAN_POINT('Ctrl Pts',(1.42378102115575,-1.,1.2514145557001));
#41291=CARTESIAN_POINT('Ctrl Pts',(1.42378102115575,1.,1.2514145557001));
#41292=CARTESIAN_POINT('Ctrl Pts',(1.42815938799387,-1.,1.25426945222639));
#41293=CARTESIAN_POINT('Ctrl Pts',(1.42815938799387,1.,1.25426945222639));
#41294=CARTESIAN_POINT('Ctrl Pts',(1.43262645609691,-1.,1.25702687965755));
#41295=CARTESIAN_POINT('Ctrl Pts',(1.43262645609691,1.,1.25702687965755));
#41296=CARTESIAN_POINT('Ctrl Pts',(1.43734919180847,-1.,1.25983531012005));
#41297=CARTESIAN_POINT('Ctrl Pts',(1.43734919180847,1.,1.25983531012005));
#41298=CARTESIAN_POINT('Ctrl Pts',(1.44236470511303,-1.,1.26273903323859));
#41299=CARTESIAN_POINT('Ctrl Pts',(1.44236470511303,1.,1.26273903323859));
#41300=CARTESIAN_POINT('Ctrl Pts',(1.44761985001662,-1.,1.26570925118868));
#41301=CARTESIAN_POINT('Ctrl Pts',(1.44761985001662,1.,1.26570925118868));
#41302=CARTESIAN_POINT('Ctrl Pts',(1.45301422764247,-1.,1.2686778680489));
#41303=CARTESIAN_POINT('Ctrl Pts',(1.45301422764247,1.,1.2686778680489));
#41304=CARTESIAN_POINT('Ctrl Pts',(1.45843906294697,-1.,1.27156805265289));
#41305=CARTESIAN_POINT('Ctrl Pts',(1.45843906294697,1.,1.27156805265289));
#41306=CARTESIAN_POINT('Ctrl Pts',(1.46382431332476,-1.,1.27433119897822));
#41307=CARTESIAN_POINT('Ctrl Pts',(1.46382431332476,1.,1.27433119897822));
#41308=CARTESIAN_POINT('Ctrl Pts',(1.46916035917133,-1.,1.2769641483109));
#41309=CARTESIAN_POINT('Ctrl Pts',(1.46916035917133,1.,1.2769641483109));
#41310=CARTESIAN_POINT('Ctrl Pts',(1.4744717526707,-1.,1.2794891824849));
#41311=CARTESIAN_POINT('Ctrl Pts',(1.4744717526707,1.,1.2794891824849));
#41312=CARTESIAN_POINT('Ctrl Pts',(1.47980070347095,-1.,1.28194158939517));
#41313=CARTESIAN_POINT('Ctrl Pts',(1.47980070347095,1.,1.28194158939517));
#41314=CARTESIAN_POINT('Ctrl Pts',(1.4851881711891,-1.,1.28435533880201));
#41315=CARTESIAN_POINT('Ctrl Pts',(1.4851881711891,1.,1.28435533880201));
#41316=CARTESIAN_POINT('Ctrl Pts',(1.4906522831278,-1.,1.2867467611644));
#41317=CARTESIAN_POINT('Ctrl Pts',(1.4906522831278,1.,1.2867467611644));
#41318=CARTESIAN_POINT('Ctrl Pts',(1.49618896881754,-1.,1.28911506584254));
#41319=CARTESIAN_POINT('Ctrl Pts',(1.49618896881754,1.,1.28911506584254));
#41320=CARTESIAN_POINT('Ctrl Pts',(1.50178230149776,-1.,1.29145022885181));
#41321=CARTESIAN_POINT('Ctrl Pts',(1.50178230149776,1.,1.29145022885181));
#41322=CARTESIAN_POINT('Ctrl Pts',(1.50741159078365,-1.,1.29373841372842));
#41323=CARTESIAN_POINT('Ctrl Pts',(1.50741159078365,1.,1.29373841372842));
#41324=CARTESIAN_POINT('Ctrl Pts',(1.51305994241402,-1.,1.29596850710509));
#41325=CARTESIAN_POINT('Ctrl Pts',(1.51305994241402,1.,1.29596850710509));
#41326=CARTESIAN_POINT('Ctrl Pts',(1.51872184912724,-1.,1.29813791800747));
#41327=CARTESIAN_POINT('Ctrl Pts',(1.51872184912724,1.,1.29813791800747));
#41328=CARTESIAN_POINT('Ctrl Pts',(1.52439957861062,-1.,1.30024984366328));
#41329=CARTESIAN_POINT('Ctrl Pts',(1.52439957861062,1.,1.30024984366328));
#41330=CARTESIAN_POINT('Ctrl Pts',(1.53009970283891,-1.,1.30231064395568));
#41331=CARTESIAN_POINT('Ctrl Pts',(1.53009970283891,1.,1.30231064395568));
#41332=CARTESIAN_POINT('Ctrl Pts',(1.53582981268977,-1.,1.30432735639489));
#41333=CARTESIAN_POINT('Ctrl Pts',(1.53582981268977,1.,1.30432735639489));
#41334=CARTESIAN_POINT('Ctrl Pts',(1.54159462645432,-1.,1.30630475189556));
#41335=CARTESIAN_POINT('Ctrl Pts',(1.54159462645432,1.,1.30630475189556));
#41336=CARTESIAN_POINT('Ctrl Pts',(1.54739413957185,-1.,1.30824393907473));
#41337=CARTESIAN_POINT('Ctrl Pts',(1.54739413957185,1.,1.30824393907473));
#41338=CARTESIAN_POINT('Ctrl Pts',(1.55322568759481,-1.,1.31014393684222));
#41339=CARTESIAN_POINT('Ctrl Pts',(1.55322568759481,1.,1.31014393684222));
#41340=CARTESIAN_POINT('Ctrl Pts',(1.55908521254821,-1.,1.31200264341696));
#41341=CARTESIAN_POINT('Ctrl Pts',(1.55908521254821,1.,1.31200264341696));
#41342=CARTESIAN_POINT('Ctrl Pts',(1.56496872402353,-1.,1.31381795281002));
#41343=CARTESIAN_POINT('Ctrl Pts',(1.56496872402353,1.,1.31381795281002));
#41344=CARTESIAN_POINT('Ctrl Pts',(1.57087397835723,-1.,1.31558903860016));
#41345=CARTESIAN_POINT('Ctrl Pts',(1.57087397835723,1.,1.31558903860016));
#41346=CARTESIAN_POINT('Ctrl Pts',(1.5768005650559,-1.,1.31731642317187));
#41347=CARTESIAN_POINT('Ctrl Pts',(1.5768005650559,1.,1.31731642317187));
#41348=CARTESIAN_POINT('Ctrl Pts',(1.58274907898834,-1.,1.31900135021432));
#41349=CARTESIAN_POINT('Ctrl Pts',(1.58274907898834,1.,1.31900135021432));
#41350=CARTESIAN_POINT('Ctrl Pts',(1.58872057258245,-1.,1.32064537110892));
#41351=CARTESIAN_POINT('Ctrl Pts',(1.58872057258245,1.,1.32064537110892));
#41352=CARTESIAN_POINT('Ctrl Pts',(1.59471591079403,-1.,1.32224985747682));
#41353=CARTESIAN_POINT('Ctrl Pts',(1.59471591079403,1.,1.32224985747682));
#41354=CARTESIAN_POINT('Ctrl Pts',(1.60073511858687,-1.,1.32381550858256));
#41355=CARTESIAN_POINT('Ctrl Pts',(1.60073511858687,1.,1.32381550858256));
#41356=CARTESIAN_POINT('Ctrl Pts',(1.60677758290954,-1.,1.32534250785782));
#41357=CARTESIAN_POINT('Ctrl Pts',(1.60677758290954,1.,1.32534250785782));
#41358=CARTESIAN_POINT('Ctrl Pts',(1.6128423401575,-1.,1.32683074483356));
#41359=CARTESIAN_POINT('Ctrl Pts',(1.6128423401575,1.,1.32683074483356));
#41360=CARTESIAN_POINT('Ctrl Pts',(1.61892832270724,-1.,1.32828000610449));
#41361=CARTESIAN_POINT('Ctrl Pts',(1.61892832270724,1.,1.32828000610449));
#41362=CARTESIAN_POINT('Ctrl Pts',(1.62503464209797,-1.,1.3296901950568));
#41363=CARTESIAN_POINT('Ctrl Pts',(1.62503464209797,1.,1.3296901950568));
#41364=CARTESIAN_POINT('Ctrl Pts',(1.63116079730923,-1.,1.33106149345645));
#41365=CARTESIAN_POINT('Ctrl Pts',(1.63116079730923,1.,1.33106149345645));
#41366=CARTESIAN_POINT('Ctrl Pts',(1.63730653475089,-1.,1.33239425103724));
#41367=CARTESIAN_POINT('Ctrl Pts',(1.63730653475089,1.,1.33239425103724));
#41368=CARTESIAN_POINT('Ctrl Pts',(1.6434717485603,-1.,1.33368890676572));
#41369=CARTESIAN_POINT('Ctrl Pts',(1.6434717485603,1.,1.33368890676572));
#41370=CARTESIAN_POINT('Ctrl Pts',(1.6496563728683,-1.,1.33494590467993));
#41371=CARTESIAN_POINT('Ctrl Pts',(1.6496563728683,1.,1.33494590467993));
#41372=CARTESIAN_POINT('Ctrl Pts',(1.65586025952593,-1.,1.33616559745172));
#41373=CARTESIAN_POINT('Ctrl Pts',(1.65586025952593,1.,1.33616559745172));
#41374=CARTESIAN_POINT('Ctrl Pts',(1.66208312541983,-1.,1.33734820885262));
#41375=CARTESIAN_POINT('Ctrl Pts',(1.66208312541983,1.,1.33734820885262));
#41376=CARTESIAN_POINT('Ctrl Pts',(1.66832460783989,-1.,1.33849388654388));
#41377=CARTESIAN_POINT('Ctrl Pts',(1.66832460783989,1.,1.33849388654388));
#41378=CARTESIAN_POINT('Ctrl Pts',(1.67458429426086,-1.,1.3396027347034));
#41379=CARTESIAN_POINT('Ctrl Pts',(1.67458429426086,1.,1.3396027347034));
#41380=CARTESIAN_POINT('Ctrl Pts',(1.68086176030362,-1.,1.34067485185203));
#41381=CARTESIAN_POINT('Ctrl Pts',(1.68086176030362,1.,1.34067485185203));
#41382=CARTESIAN_POINT('Ctrl Pts',(1.68715660868764,-1.,1.341710374848));
#41383=CARTESIAN_POINT('Ctrl Pts',(1.68715660868764,1.,1.341710374848));
#41384=CARTESIAN_POINT('Ctrl Pts',(1.6934684849687,-1.,1.34270948206319));
#41385=CARTESIAN_POINT('Ctrl Pts',(1.6934684849687,1.,1.34270948206319));
#41386=CARTESIAN_POINT('Ctrl Pts',(1.69979707754427,-1.,1.34367237124483));
#41387=CARTESIAN_POINT('Ctrl Pts',(1.69979707754427,1.,1.34367237124483));
#41388=CARTESIAN_POINT('Ctrl Pts',(1.70614212266738,-1.,1.34459924533831));
#41389=CARTESIAN_POINT('Ctrl Pts',(1.70614212266738,1.,1.34459924533831));
#41390=CARTESIAN_POINT('Ctrl Pts',(1.71250340686822,-1.,1.34549029589416));
#41391=CARTESIAN_POINT('Ctrl Pts',(1.71250340686822,1.,1.34549029589416));
#41392=CARTESIAN_POINT('Ctrl Pts',(1.7188807715049,-1.,1.34634568653227));
#41393=CARTESIAN_POINT('Ctrl Pts',(1.7188807715049,1.,1.34634568653227));
#41394=CARTESIAN_POINT('Ctrl Pts',(1.72527410680674,-1.,1.34716554819527));
#41395=CARTESIAN_POINT('Ctrl Pts',(1.72527410680674,1.,1.34716554819527));
#41396=CARTESIAN_POINT('Ctrl Pts',(1.7304014965394,-1.,1.34779309152035));
#41397=CARTESIAN_POINT('Ctrl Pts',(1.7304014965394,1.,1.34779309152035));
#41398=CARTESIAN_POINT('Ctrl Pts',(1.73425417885907,-1.,1.34824783112887));
#41399=CARTESIAN_POINT('Ctrl Pts',(1.73425417885907,1.,1.34824783112887));
#41400=CARTESIAN_POINT('Ctrl Pts',(1.73682580585691,-1.,1.34854391898045));
#41401=CARTESIAN_POINT('Ctrl Pts',(1.73682580585691,1.,1.34854391898045));
#41402=CARTESIAN_POINT('Ctrl Pts',(1.73811241238545,-1.,1.34869019493419));
#41403=CARTESIAN_POINT('Ctrl Pts',(1.73811241238545,1.,1.34869019493419));
#41404=CARTESIAN_POINT('',(1.31362392696032,1.,1.15624053661742));
#41405=CARTESIAN_POINT('Ctrl Pts',(1.31362392696032,1.,1.15624053661742));
#41406=CARTESIAN_POINT('Ctrl Pts',(1.31722977216397,1.,1.15950888730809));
#41407=CARTESIAN_POINT('Ctrl Pts',(1.32428080721772,1.,1.16589330093588));
#41408=CARTESIAN_POINT('Ctrl Pts',(1.33437539347008,1.,1.17501305789857));
#41409=CARTESIAN_POINT('Ctrl Pts',(1.34687054001093,1.,1.18625865667441));
#41410=CARTESIAN_POINT('Ctrl Pts',(1.36088705043885,1.,1.1987959077932));
#41411=CARTESIAN_POINT('Ctrl Pts',(1.37331915607905,1.,1.20982812925645));
#41412=CARTESIAN_POINT('Ctrl Pts',(1.38420564527715,1.,1.21938737280852));
#41413=CARTESIAN_POINT('Ctrl Pts',(1.39361389568796,1.,1.22752961899387));
#41414=CARTESIAN_POINT('Ctrl Pts',(1.40164708206106,1.,1.23434087290423));
#41415=CARTESIAN_POINT('Ctrl Pts',(1.40845295531283,1.,1.23994455029534));
#41416=CARTESIAN_POINT('Ctrl Pts',(1.41422913175179,1.,1.24450600513056));
#41417=CARTESIAN_POINT('Ctrl Pts',(1.41923722596025,1.,1.24824430986571));
#41418=CARTESIAN_POINT('Ctrl Pts',(1.42378102115575,1.,1.2514145557001));
#41419=CARTESIAN_POINT('Ctrl Pts',(1.42815938799387,1.,1.25426945222639));
#41420=CARTESIAN_POINT('Ctrl Pts',(1.43262645609691,1.,1.25702687965755));
#41421=CARTESIAN_POINT('Ctrl Pts',(1.43734919180847,1.,1.25983531012005));
#41422=CARTESIAN_POINT('Ctrl Pts',(1.44236470511303,1.,1.26273903323859));
#41423=CARTESIAN_POINT('Ctrl Pts',(1.44761985001662,1.,1.26570925118868));
#41424=CARTESIAN_POINT('Ctrl Pts',(1.45301422764247,1.,1.2686778680489));
#41425=CARTESIAN_POINT('Ctrl Pts',(1.45843906294697,1.,1.27156805265289));
#41426=CARTESIAN_POINT('Ctrl Pts',(1.46382431332476,1.,1.27433119897822));
#41427=CARTESIAN_POINT('Ctrl Pts',(1.46916035917133,1.,1.2769641483109));
#41428=CARTESIAN_POINT('Ctrl Pts',(1.4744717526707,1.,1.2794891824849));
#41429=CARTESIAN_POINT('Ctrl Pts',(1.47980070347095,1.,1.28194158939517));
#41430=CARTESIAN_POINT('Ctrl Pts',(1.4851881711891,1.,1.28435533880201));
#41431=CARTESIAN_POINT('Ctrl Pts',(1.4906522831278,1.,1.2867467611644));
#41432=CARTESIAN_POINT('Ctrl Pts',(1.49618896881754,1.,1.28911506584254));
#41433=CARTESIAN_POINT('Ctrl Pts',(1.50178230149776,1.,1.29145022885181));
#41434=CARTESIAN_POINT('Ctrl Pts',(1.50741159078365,1.,1.29373841372842));
#41435=CARTESIAN_POINT('Ctrl Pts',(1.51305994241402,1.,1.29596850710509));
#41436=CARTESIAN_POINT('Ctrl Pts',(1.51872184912724,1.,1.29813791800747));
#41437=CARTESIAN_POINT('Ctrl Pts',(1.52439957861062,1.,1.30024984366328));
#41438=CARTESIAN_POINT('Ctrl Pts',(1.53009970283891,1.,1.30231064395568));
#41439=CARTESIAN_POINT('Ctrl Pts',(1.53582981268977,1.,1.30432735639489));
#41440=CARTESIAN_POINT('Ctrl Pts',(1.54159462645432,1.,1.30630475189556));
#41441=CARTESIAN_POINT('Ctrl Pts',(1.54739413957185,1.,1.30824393907473));
#41442=CARTESIAN_POINT('Ctrl Pts',(1.55322568759481,1.,1.31014393684222));
#41443=CARTESIAN_POINT('Ctrl Pts',(1.55908521254821,1.,1.31200264341696));
#41444=CARTESIAN_POINT('Ctrl Pts',(1.56496872402353,1.,1.31381795281002));
#41445=CARTESIAN_POINT('Ctrl Pts',(1.57087397835723,1.,1.31558903860016));
#41446=CARTESIAN_POINT('Ctrl Pts',(1.5768005650559,1.,1.31731642317187));
#41447=CARTESIAN_POINT('Ctrl Pts',(1.58274907898834,1.,1.31900135021432));
#41448=CARTESIAN_POINT('Ctrl Pts',(1.58872057258245,1.,1.32064537110892));
#41449=CARTESIAN_POINT('Ctrl Pts',(1.59471591079403,1.,1.32224985747682));
#41450=CARTESIAN_POINT('Ctrl Pts',(1.60073511858687,1.,1.32381550858256));
#41451=CARTESIAN_POINT('Ctrl Pts',(1.60677758290954,1.,1.32534250785782));
#41452=CARTESIAN_POINT('Ctrl Pts',(1.6128423401575,1.,1.32683074483356));
#41453=CARTESIAN_POINT('Ctrl Pts',(1.61892832270724,1.,1.32828000610449));
#41454=CARTESIAN_POINT('Ctrl Pts',(1.62503464209797,1.,1.3296901950568));
#41455=CARTESIAN_POINT('Ctrl Pts',(1.63116079730923,1.,1.33106149345645));
#41456=CARTESIAN_POINT('Ctrl Pts',(1.63730653475089,1.,1.33239425103724));
#41457=CARTESIAN_POINT('Ctrl Pts',(1.6434717485603,1.,1.33368890676572));
#41458=CARTESIAN_POINT('Ctrl Pts',(1.6496563728683,1.,1.33494590467993));
#41459=CARTESIAN_POINT('Ctrl Pts',(1.65586025952593,1.,1.33616559745172));
#41460=CARTESIAN_POINT('Ctrl Pts',(1.66208312541983,1.,1.33734820885262));
#41461=CARTESIAN_POINT('Ctrl Pts',(1.66832460783989,1.,1.33849388654388));
#41462=CARTESIAN_POINT('Ctrl Pts',(1.67458429426086,1.,1.3396027347034));
#41463=CARTESIAN_POINT('Ctrl Pts',(1.68086176030362,1.,1.34067485185203));
#41464=CARTESIAN_POINT('Ctrl Pts',(1.68715660868764,1.,1.341710374848));
#41465=CARTESIAN_POINT('Ctrl Pts',(1.6934684849687,1.,1.34270948206319));
#41466=CARTESIAN_POINT('Ctrl Pts',(1.69979707754427,1.,1.34367237124483));
#41467=CARTESIAN_POINT('Ctrl Pts',(1.70614212266738,1.,1.34459924533831));
#41468=CARTESIAN_POINT('Ctrl Pts',(1.71250340686822,1.,1.34549029589416));
#41469=CARTESIAN_POINT('Ctrl Pts',(1.7188807715049,1.,1.34634568653227));
#41470=CARTESIAN_POINT('Ctrl Pts',(1.72527410680674,1.,1.34716554819527));
#41471=CARTESIAN_POINT('Ctrl Pts',(1.7304014965394,1.,1.34779309152035));
#41472=CARTESIAN_POINT('Ctrl Pts',(1.73425417885907,1.,1.34824783112887));
#41473=CARTESIAN_POINT('Ctrl Pts',(1.73682580585691,1.,1.34854391898045));
#41474=CARTESIAN_POINT('Ctrl Pts',(1.73811241238545,1.,1.34869019493419));
#41475=CARTESIAN_POINT('',(1.31362392696032,0.,1.15624053661742));
#41476=CARTESIAN_POINT('Origin',(0.,0.,0.));
#41477=CARTESIAN_POINT('',(1.15624053661742,1.,1.31362392696033));
#41478=CARTESIAN_POINT('Origin',(0.,1.,0.));
#41479=CARTESIAN_POINT('',(1.15624053661742,0.,1.31362392696032));
#41480=CARTESIAN_POINT('Ctrl Pts',(1.34869019493419,-1.,1.73811241238545));
#41481=CARTESIAN_POINT('Ctrl Pts',(1.34869019493419,1.,1.73811241238545));
#41482=CARTESIAN_POINT('Ctrl Pts',(1.34854391898145,-1.,1.73682580585819));
#41483=CARTESIAN_POINT('Ctrl Pts',(1.34854391898145,1.,1.73682580585819));
#41484=CARTESIAN_POINT('Ctrl Pts',(1.34824783113158,-1.,1.73425417886255));
#41485=CARTESIAN_POINT('Ctrl Pts',(1.34824783113158,1.,1.73425417886255));
#41486=CARTESIAN_POINT('Ctrl Pts',(1.3477930915247,-1.,1.73040149654497));
#41487=CARTESIAN_POINT('Ctrl Pts',(1.3477930915247,1.,1.73040149654497));
#41488=CARTESIAN_POINT('Ctrl Pts',(1.34716554820013,-1.,1.72527410681298));
#41489=CARTESIAN_POINT('Ctrl Pts',(1.34716554820013,1.,1.72527410681298));
#41490=CARTESIAN_POINT('Ctrl Pts',(1.34634568653586,-1.,1.7188807715095));
#41491=CARTESIAN_POINT('Ctrl Pts',(1.34634568653586,1.,1.7188807715095));
#41492=CARTESIAN_POINT('Ctrl Pts',(1.34549029589563,-1.,1.71250340687011));
#41493=CARTESIAN_POINT('Ctrl Pts',(1.34549029589563,1.,1.71250340687011));
#41494=CARTESIAN_POINT('Ctrl Pts',(1.34459924533783,-1.,1.70614212266676));
#41495=CARTESIAN_POINT('Ctrl Pts',(1.34459924533783,1.,1.70614212266676));
#41496=CARTESIAN_POINT('Ctrl Pts',(1.34367237124322,-1.,1.69979707754221));
#41497=CARTESIAN_POINT('Ctrl Pts',(1.34367237124322,1.,1.69979707754221));
#41498=CARTESIAN_POINT('Ctrl Pts',(1.34270948206139,-1.,1.6934684849664));
#41499=CARTESIAN_POINT('Ctrl Pts',(1.34270948206139,1.,1.6934684849664));
#41500=CARTESIAN_POINT('Ctrl Pts',(1.34171037484673,-1.,1.68715660868602));
#41501=CARTESIAN_POINT('Ctrl Pts',(1.34171037484673,1.,1.68715660868602));
#41502=CARTESIAN_POINT('Ctrl Pts',(1.3406748518516,-1.,1.68086176030308));
#41503=CARTESIAN_POINT('Ctrl Pts',(1.3406748518516,1.,1.68086176030308));
#41504=CARTESIAN_POINT('Ctrl Pts',(1.33960273470372,-1.,1.67458429426126));
#41505=CARTESIAN_POINT('Ctrl Pts',(1.33960273470372,1.,1.67458429426126));
#41506=CARTESIAN_POINT('Ctrl Pts',(1.33849388654458,-1.,1.66832460784078));
#41507=CARTESIAN_POINT('Ctrl Pts',(1.33849388654458,1.,1.66832460784078));
#41508=CARTESIAN_POINT('Ctrl Pts',(1.33734820885331,-1.,1.66208312542073));
#41509=CARTESIAN_POINT('Ctrl Pts',(1.33734820885331,1.,1.66208312542073));
#41510=CARTESIAN_POINT('Ctrl Pts',(1.33616559745217,-1.,1.65586025952651));
#41511=CARTESIAN_POINT('Ctrl Pts',(1.33616559745217,1.,1.65586025952651));
#41512=CARTESIAN_POINT('Ctrl Pts',(1.33494590468003,-1.,1.64965637286843));
#41513=CARTESIAN_POINT('Ctrl Pts',(1.33494590468003,1.,1.64965637286843));
#41514=CARTESIAN_POINT('Ctrl Pts',(1.33368890676554,-1.,1.64347174856007));
#41515=CARTESIAN_POINT('Ctrl Pts',(1.33368890676554,1.,1.64347174856007));
#41516=CARTESIAN_POINT('Ctrl Pts',(1.33239425103694,-1.,1.6373065347505));
#41517=CARTESIAN_POINT('Ctrl Pts',(1.33239425103694,1.,1.6373065347505));
#41518=CARTESIAN_POINT('Ctrl Pts',(1.33106149345618,-1.,1.63116079730887));
#41519=CARTESIAN_POINT('Ctrl Pts',(1.33106149345618,1.,1.63116079730887));
#41520=CARTESIAN_POINT('Ctrl Pts',(1.32969019505665,-1.,1.62503464209777));
#41521=CARTESIAN_POINT('Ctrl Pts',(1.32969019505665,1.,1.62503464209777));
#41522=CARTESIAN_POINT('Ctrl Pts',(1.32828000610448,-1.,1.61892832270723));
#41523=CARTESIAN_POINT('Ctrl Pts',(1.32828000610448,1.,1.61892832270723));
#41524=CARTESIAN_POINT('Ctrl Pts',(1.32683074483365,-1.,1.61284234015762));
#41525=CARTESIAN_POINT('Ctrl Pts',(1.32683074483365,1.,1.61284234015762));
#41526=CARTESIAN_POINT('Ctrl Pts',(1.32534250785794,-1.,1.6067775829097));
#41527=CARTESIAN_POINT('Ctrl Pts',(1.32534250785794,1.,1.6067775829097));
#41528=CARTESIAN_POINT('Ctrl Pts',(1.32381550858266,-1.,1.600735118587));
#41529=CARTESIAN_POINT('Ctrl Pts',(1.32381550858266,1.,1.600735118587));
#41530=CARTESIAN_POINT('Ctrl Pts',(1.32224985747686,-1.,1.59471591079408));
#41531=CARTESIAN_POINT('Ctrl Pts',(1.32224985747686,1.,1.59471591079408));
#41532=CARTESIAN_POINT('Ctrl Pts',(1.32064537110891,-1.,1.58872057258244));
#41533=CARTESIAN_POINT('Ctrl Pts',(1.32064537110891,1.,1.58872057258244));
#41534=CARTESIAN_POINT('Ctrl Pts',(1.31900135021428,-1.,1.58274907898829));
#41535=CARTESIAN_POINT('Ctrl Pts',(1.31900135021428,1.,1.58274907898829));
#41536=CARTESIAN_POINT('Ctrl Pts',(1.31731642317183,-1.,1.57680056505585));
#41537=CARTESIAN_POINT('Ctrl Pts',(1.31731642317183,1.,1.57680056505585));
#41538=CARTESIAN_POINT('Ctrl Pts',(1.31558903860015,-1.,1.57087397835721));
#41539=CARTESIAN_POINT('Ctrl Pts',(1.31558903860015,1.,1.57087397835721));
#41540=CARTESIAN_POINT('Ctrl Pts',(1.31381795281002,-1.,1.56496872402352));
#41541=CARTESIAN_POINT('Ctrl Pts',(1.31381795281002,1.,1.56496872402352));
#41542=CARTESIAN_POINT('Ctrl Pts',(1.31200264341696,-1.,1.55908521254822));
#41543=CARTESIAN_POINT('Ctrl Pts',(1.31200264341696,1.,1.55908521254822));
#41544=CARTESIAN_POINT('Ctrl Pts',(1.31014393684221,-1.,1.55322568759481));
#41545=CARTESIAN_POINT('Ctrl Pts',(1.31014393684221,1.,1.55322568759481));
#41546=CARTESIAN_POINT('Ctrl Pts',(1.30824393907471,-1.,1.54739413957183));
#41547=CARTESIAN_POINT('Ctrl Pts',(1.30824393907471,1.,1.54739413957183));
#41548=CARTESIAN_POINT('Ctrl Pts',(1.30630475189553,-1.,1.54159462645428));
#41549=CARTESIAN_POINT('Ctrl Pts',(1.30630475189553,1.,1.54159462645428));
#41550=CARTESIAN_POINT('Ctrl Pts',(1.30432735639487,-1.,1.53582981268976));
#41551=CARTESIAN_POINT('Ctrl Pts',(1.30432735639487,1.,1.53582981268976));
#41552=CARTESIAN_POINT('Ctrl Pts',(1.3023106439557,-1.,1.53009970283893));
#41553=CARTESIAN_POINT('Ctrl Pts',(1.3023106439557,1.,1.53009970283893));
#41554=CARTESIAN_POINT('Ctrl Pts',(1.30024984366334,-1.,1.5243995786107));
#41555=CARTESIAN_POINT('Ctrl Pts',(1.30024984366334,1.,1.5243995786107));
#41556=CARTESIAN_POINT('Ctrl Pts',(1.29813791800757,-1.,1.51872184912735));
#41557=CARTESIAN_POINT('Ctrl Pts',(1.29813791800757,1.,1.51872184912735));
#41558=CARTESIAN_POINT('Ctrl Pts',(1.29596850710518,-1.,1.51305994241412));
#41559=CARTESIAN_POINT('Ctrl Pts',(1.29596850710518,1.,1.51305994241412));
#41560=CARTESIAN_POINT('Ctrl Pts',(1.29373841372843,-1.,1.50741159078367));
#41561=CARTESIAN_POINT('Ctrl Pts',(1.29373841372843,1.,1.50741159078367));
#41562=CARTESIAN_POINT('Ctrl Pts',(1.29145022885171,-1.,1.50178230149764));
#41563=CARTESIAN_POINT('Ctrl Pts',(1.29145022885171,1.,1.50178230149764));
#41564=CARTESIAN_POINT('Ctrl Pts',(1.28911506584232,-1.,1.49618896881729));
#41565=CARTESIAN_POINT('Ctrl Pts',(1.28911506584232,1.,1.49618896881729));
#41566=CARTESIAN_POINT('Ctrl Pts',(1.28674676116415,-1.,1.4906522831275));
#41567=CARTESIAN_POINT('Ctrl Pts',(1.28674676116415,1.,1.4906522831275));
#41568=CARTESIAN_POINT('Ctrl Pts',(1.28435533880184,-1.,1.48518817118891));
#41569=CARTESIAN_POINT('Ctrl Pts',(1.28435533880184,1.,1.48518817118891));
#41570=CARTESIAN_POINT('Ctrl Pts',(1.28194158939522,-1.,1.47980070347102));
#41571=CARTESIAN_POINT('Ctrl Pts',(1.28194158939522,1.,1.47980070347102));
#41572=CARTESIAN_POINT('Ctrl Pts',(1.27948918248524,-1.,1.4744717526711));
#41573=CARTESIAN_POINT('Ctrl Pts',(1.27948918248524,1.,1.4744717526711));
#41574=CARTESIAN_POINT('Ctrl Pts',(1.27696414831144,-1.,1.46916035917197));
#41575=CARTESIAN_POINT('Ctrl Pts',(1.27696414831144,1.,1.46916035917197));
#41576=CARTESIAN_POINT('Ctrl Pts',(1.27433119897877,-1.,1.4638243133254));
#41577=CARTESIAN_POINT('Ctrl Pts',(1.27433119897877,1.,1.4638243133254));
#41578=CARTESIAN_POINT('Ctrl Pts',(1.27156805265312,-1.,1.45843906294725));
#41579=CARTESIAN_POINT('Ctrl Pts',(1.27156805265312,1.,1.45843906294725));
#41580=CARTESIAN_POINT('Ctrl Pts',(1.26867786804854,-1.,1.45301422764205));
#41581=CARTESIAN_POINT('Ctrl Pts',(1.26867786804854,1.,1.45301422764205));
#41582=CARTESIAN_POINT('Ctrl Pts',(1.26570925118767,-1.,1.44761985001544));
#41583=CARTESIAN_POINT('Ctrl Pts',(1.26570925118767,1.,1.44761985001544));
#41584=CARTESIAN_POINT('Ctrl Pts',(1.26273903323723,-1.,1.44236470511145));
#41585=CARTESIAN_POINT('Ctrl Pts',(1.26273903323723,1.,1.44236470511145));
#41586=CARTESIAN_POINT('Ctrl Pts',(1.25983531011894,-1.,1.43734919180719));
#41587=CARTESIAN_POINT('Ctrl Pts',(1.25983531011894,1.,1.43734919180719));
#41588=CARTESIAN_POINT('Ctrl Pts',(1.25702687965744,-1.,1.43262645609679));
#41589=CARTESIAN_POINT('Ctrl Pts',(1.25702687965744,1.,1.43262645609679));
#41590=CARTESIAN_POINT('Ctrl Pts',(1.25426945222783,-1.,1.42815938799555));
#41591=CARTESIAN_POINT('Ctrl Pts',(1.25426945222783,1.,1.42815938799555));
#41592=CARTESIAN_POINT('Ctrl Pts',(1.25141455570299,-1.,1.42378102115911));
#41593=CARTESIAN_POINT('Ctrl Pts',(1.25141455570299,1.,1.42378102115911));
#41594=CARTESIAN_POINT('Ctrl Pts',(1.24824430986911,-1.,1.41923722596421));
#41595=CARTESIAN_POINT('Ctrl Pts',(1.24824430986911,1.,1.41923722596421));
#41596=CARTESIAN_POINT('Ctrl Pts',(1.24450600513278,-1.,1.41422913175437));
#41597=CARTESIAN_POINT('Ctrl Pts',(1.24450600513278,1.,1.41422913175437));
#41598=CARTESIAN_POINT('Ctrl Pts',(1.23994455029421,-1.,1.40845295531151));
#41599=CARTESIAN_POINT('Ctrl Pts',(1.23994455029421,1.,1.40845295531151));
#41600=CARTESIAN_POINT('Ctrl Pts',(1.23434087289768,-1.,1.40164708205345));
#41601=CARTESIAN_POINT('Ctrl Pts',(1.23434087289768,1.,1.40164708205345));
#41602=CARTESIAN_POINT('Ctrl Pts',(1.22752961898063,-1.,1.39361389567257));
#41603=CARTESIAN_POINT('Ctrl Pts',(1.22752961898063,1.,1.39361389567257));
#41604=CARTESIAN_POINT('Ctrl Pts',(1.21938737278853,-1.,1.38420564525391));
#41605=CARTESIAN_POINT('Ctrl Pts',(1.21938737278853,1.,1.38420564525391));
#41606=CARTESIAN_POINT('Ctrl Pts',(1.20982812923113,-1.,1.37331915604962));
#41607=CARTESIAN_POINT('Ctrl Pts',(1.20982812923113,1.,1.37331915604962));
#41608=CARTESIAN_POINT('Ctrl Pts',(1.1987959077656,-1.,1.36088705040677));
#41609=CARTESIAN_POINT('Ctrl Pts',(1.1987959077656,1.,1.36088705040677));
#41610=CARTESIAN_POINT('Ctrl Pts',(1.18625865664915,-1.,1.34687053998157));
#41611=CARTESIAN_POINT('Ctrl Pts',(1.18625865664915,1.,1.34687053998157));
#41612=CARTESIAN_POINT('Ctrl Pts',(1.17501305787994,-1.,1.33437539344842));
#41613=CARTESIAN_POINT('Ctrl Pts',(1.17501305787994,1.,1.33437539344842));
#41614=CARTESIAN_POINT('Ctrl Pts',(1.16589330092532,-1.,1.32428080720544));
#41615=CARTESIAN_POINT('Ctrl Pts',(1.16589330092532,1.,1.32428080720544));
#41616=CARTESIAN_POINT('Ctrl Pts',(1.15950888730433,-1.,1.3172297721596));
#41617=CARTESIAN_POINT('Ctrl Pts',(1.15950888730433,1.,1.3172297721596));
#41618=CARTESIAN_POINT('Ctrl Pts',(1.15624053661742,-1.,1.31362392696033));
#41619=CARTESIAN_POINT('Ctrl Pts',(1.15624053661742,1.,1.31362392696033));
#41620=CARTESIAN_POINT('',(1.34869019493419,1.,1.73811241238545));
#41621=CARTESIAN_POINT('Ctrl Pts',(1.34869019493419,1.,1.73811241238545));
#41622=CARTESIAN_POINT('Ctrl Pts',(1.34854391898145,1.,1.73682580585819));
#41623=CARTESIAN_POINT('Ctrl Pts',(1.34824783113158,1.,1.73425417886255));
#41624=CARTESIAN_POINT('Ctrl Pts',(1.3477930915247,1.,1.73040149654497));
#41625=CARTESIAN_POINT('Ctrl Pts',(1.34716554820013,1.,1.72527410681298));
#41626=CARTESIAN_POINT('Ctrl Pts',(1.34634568653586,1.,1.7188807715095));
#41627=CARTESIAN_POINT('Ctrl Pts',(1.34549029589563,1.,1.71250340687011));
#41628=CARTESIAN_POINT('Ctrl Pts',(1.34459924533783,1.,1.70614212266676));
#41629=CARTESIAN_POINT('Ctrl Pts',(1.34367237124322,1.,1.69979707754221));
#41630=CARTESIAN_POINT('Ctrl Pts',(1.34270948206139,1.,1.6934684849664));
#41631=CARTESIAN_POINT('Ctrl Pts',(1.34171037484673,1.,1.68715660868602));
#41632=CARTESIAN_POINT('Ctrl Pts',(1.3406748518516,1.,1.68086176030308));
#41633=CARTESIAN_POINT('Ctrl Pts',(1.33960273470372,1.,1.67458429426126));
#41634=CARTESIAN_POINT('Ctrl Pts',(1.33849388654458,1.,1.66832460784078));
#41635=CARTESIAN_POINT('Ctrl Pts',(1.33734820885331,1.,1.66208312542073));
#41636=CARTESIAN_POINT('Ctrl Pts',(1.33616559745217,1.,1.65586025952651));
#41637=CARTESIAN_POINT('Ctrl Pts',(1.33494590468003,1.,1.64965637286843));
#41638=CARTESIAN_POINT('Ctrl Pts',(1.33368890676554,1.,1.64347174856007));
#41639=CARTESIAN_POINT('Ctrl Pts',(1.33239425103694,1.,1.6373065347505));
#41640=CARTESIAN_POINT('Ctrl Pts',(1.33106149345618,1.,1.63116079730887));
#41641=CARTESIAN_POINT('Ctrl Pts',(1.32969019505665,1.,1.62503464209777));
#41642=CARTESIAN_POINT('Ctrl Pts',(1.32828000610448,1.,1.61892832270723));
#41643=CARTESIAN_POINT('Ctrl Pts',(1.32683074483365,1.,1.61284234015762));
#41644=CARTESIAN_POINT('Ctrl Pts',(1.32534250785794,1.,1.6067775829097));
#41645=CARTESIAN_POINT('Ctrl Pts',(1.32381550858266,1.,1.600735118587));
#41646=CARTESIAN_POINT('Ctrl Pts',(1.32224985747686,1.,1.59471591079408));
#41647=CARTESIAN_POINT('Ctrl Pts',(1.32064537110891,1.,1.58872057258244));
#41648=CARTESIAN_POINT('Ctrl Pts',(1.31900135021428,1.,1.58274907898829));
#41649=CARTESIAN_POINT('Ctrl Pts',(1.31731642317183,1.,1.57680056505585));
#41650=CARTESIAN_POINT('Ctrl Pts',(1.31558903860015,1.,1.57087397835721));
#41651=CARTESIAN_POINT('Ctrl Pts',(1.31381795281002,1.,1.56496872402352));
#41652=CARTESIAN_POINT('Ctrl Pts',(1.31200264341696,1.,1.55908521254822));
#41653=CARTESIAN_POINT('Ctrl Pts',(1.31014393684221,1.,1.55322568759481));
#41654=CARTESIAN_POINT('Ctrl Pts',(1.30824393907471,1.,1.54739413957183));
#41655=CARTESIAN_POINT('Ctrl Pts',(1.30630475189553,1.,1.54159462645428));
#41656=CARTESIAN_POINT('Ctrl Pts',(1.30432735639487,1.,1.53582981268976));
#41657=CARTESIAN_POINT('Ctrl Pts',(1.3023106439557,1.,1.53009970283893));
#41658=CARTESIAN_POINT('Ctrl Pts',(1.30024984366334,1.,1.5243995786107));
#41659=CARTESIAN_POINT('Ctrl Pts',(1.29813791800757,1.,1.51872184912735));
#41660=CARTESIAN_POINT('Ctrl Pts',(1.29596850710518,1.,1.51305994241412));
#41661=CARTESIAN_POINT('Ctrl Pts',(1.29373841372843,1.,1.50741159078367));
#41662=CARTESIAN_POINT('Ctrl Pts',(1.29145022885171,1.,1.50178230149764));
#41663=CARTESIAN_POINT('Ctrl Pts',(1.28911506584232,1.,1.49618896881729));
#41664=CARTESIAN_POINT('Ctrl Pts',(1.28674676116415,1.,1.4906522831275));
#41665=CARTESIAN_POINT('Ctrl Pts',(1.28435533880184,1.,1.48518817118891));
#41666=CARTESIAN_POINT('Ctrl Pts',(1.28194158939522,1.,1.47980070347102));
#41667=CARTESIAN_POINT('Ctrl Pts',(1.27948918248524,1.,1.4744717526711));
#41668=CARTESIAN_POINT('Ctrl Pts',(1.27696414831144,1.,1.46916035917197));
#41669=CARTESIAN_POINT('Ctrl Pts',(1.27433119897877,1.,1.4638243133254));
#41670=CARTESIAN_POINT('Ctrl Pts',(1.27156805265312,1.,1.45843906294725));
#41671=CARTESIAN_POINT('Ctrl Pts',(1.26867786804854,1.,1.45301422764205));
#41672=CARTESIAN_POINT('Ctrl Pts',(1.26570925118767,1.,1.44761985001544));
#41673=CARTESIAN_POINT('Ctrl Pts',(1.26273903323723,1.,1.44236470511145));
#41674=CARTESIAN_POINT('Ctrl Pts',(1.25983531011894,1.,1.43734919180719));
#41675=CARTESIAN_POINT('Ctrl Pts',(1.25702687965744,1.,1.43262645609679));
#41676=CARTESIAN_POINT('Ctrl Pts',(1.25426945222783,1.,1.42815938799555));
#41677=CARTESIAN_POINT('Ctrl Pts',(1.25141455570299,1.,1.42378102115911));
#41678=CARTESIAN_POINT('Ctrl Pts',(1.24824430986911,1.,1.41923722596421));
#41679=CARTESIAN_POINT('Ctrl Pts',(1.24450600513278,1.,1.41422913175437));
#41680=CARTESIAN_POINT('Ctrl Pts',(1.23994455029421,1.,1.40845295531151));
#41681=CARTESIAN_POINT('Ctrl Pts',(1.23434087289768,1.,1.40164708205345));
#41682=CARTESIAN_POINT('Ctrl Pts',(1.22752961898063,1.,1.39361389567257));
#41683=CARTESIAN_POINT('Ctrl Pts',(1.21938737278853,1.,1.38420564525391));
#41684=CARTESIAN_POINT('Ctrl Pts',(1.20982812923113,1.,1.37331915604962));
#41685=CARTESIAN_POINT('Ctrl Pts',(1.1987959077656,1.,1.36088705040677));
#41686=CARTESIAN_POINT('Ctrl Pts',(1.18625865664915,1.,1.34687053998157));
#41687=CARTESIAN_POINT('Ctrl Pts',(1.17501305787994,1.,1.33437539344842));
#41688=CARTESIAN_POINT('Ctrl Pts',(1.16589330092532,1.,1.32428080720544));
#41689=CARTESIAN_POINT('Ctrl Pts',(1.15950888730433,1.,1.3172297721596));
#41690=CARTESIAN_POINT('Ctrl Pts',(1.15624053661742,1.,1.31362392696033));
#41691=CARTESIAN_POINT('',(1.34869019493419,0.,1.73811241238545));
#41692=CARTESIAN_POINT('Origin',(1.23627494547115,0.,1.81978687191668));
#41693=CARTESIAN_POINT('',(1.23627494547115,1.,1.81978687191668));
#41694=CARTESIAN_POINT('',(1.34869019493419,1.,1.73811241238545));
#41695=CARTESIAN_POINT('',(1.23627494547115,0.,1.81978687191668));
#41696=CARTESIAN_POINT('Ctrl Pts',(0.892032620296855,-1.,1.5055822144029));
#41697=CARTESIAN_POINT('Ctrl Pts',(0.892032620296855,1.,1.5055822144029));
#41698=CARTESIAN_POINT('Ctrl Pts',(0.894452006967538,-1.,1.50980486807181));
#41699=CARTESIAN_POINT('Ctrl Pts',(0.894452006967538,1.,1.50980486807181));
#41700=CARTESIAN_POINT('Ctrl Pts',(0.89918504749193,-1.,1.51805569591479));
#41701=CARTESIAN_POINT('Ctrl Pts',(0.89918504749193,1.,1.51805569591479));
#41702=CARTESIAN_POINT('Ctrl Pts',(0.905967409640498,-1.,1.52984849890434));
#41703=CARTESIAN_POINT('Ctrl Pts',(0.905967409640498,1.,1.52984849890434));
#41704=CARTESIAN_POINT('Ctrl Pts',(0.914375919046579,-1.,1.54440491152808));
#41705=CARTESIAN_POINT('Ctrl Pts',(0.914375919046579,1.,1.54440491152808));
#41706=CARTESIAN_POINT('Ctrl Pts',(0.923832188966322,-1.,1.56065988582509));
#41707=CARTESIAN_POINT('Ctrl Pts',(0.923832188966322,1.,1.56065988582509));
#41708=CARTESIAN_POINT('Ctrl Pts',(0.932246680128848,-1.,1.57499388385561));
#41709=CARTESIAN_POINT('Ctrl Pts',(0.932246680128848,1.,1.57499388385561));
#41710=CARTESIAN_POINT('Ctrl Pts',(0.939646377909319,-1.,1.58744937489796));
#41711=CARTESIAN_POINT('Ctrl Pts',(0.939646377909319,1.,1.58744937489796));
#41712=CARTESIAN_POINT('Ctrl Pts',(0.946078063325795,-1.,1.59810042045408));
#41713=CARTESIAN_POINT('Ctrl Pts',(0.946078063325795,1.,1.59810042045408));
#41714=CARTESIAN_POINT('Ctrl Pts',(0.951613284361247,-1.,1.60706069897794));
#41715=CARTESIAN_POINT('Ctrl Pts',(0.951613284361247,1.,1.60706069897794));
#41716=CARTESIAN_POINT('Ctrl Pts',(0.956354422921572,-1.,1.61449324337233));
#41717=CARTESIAN_POINT('Ctrl Pts',(0.956354422921572,1.,1.61449324337233));
#41718=CARTESIAN_POINT('Ctrl Pts',(0.960438326099958,-1.,1.62061638139929));
#41719=CARTESIAN_POINT('Ctrl Pts',(0.960438326099958,1.,1.62061638139929));
#41720=CARTESIAN_POINT('Ctrl Pts',(0.964046107037821,-1.,1.6257193066974));
#41721=CARTESIAN_POINT('Ctrl Pts',(0.964046107037821,1.,1.6257193066974));
#41722=CARTESIAN_POINT('Ctrl Pts',(0.967387853228041,-1.,1.63013849959083));
#41723=CARTESIAN_POINT('Ctrl Pts',(0.967387853228041,1.,1.63013849959083));
#41724=CARTESIAN_POINT('Ctrl Pts',(0.970669715996356,-1.,1.63420665729609));
#41725=CARTESIAN_POINT('Ctrl Pts',(0.970669715996356,1.,1.63420665729609));
#41726=CARTESIAN_POINT('Ctrl Pts',(0.974066058287501,-1.,1.63820952658157));
#41727=CARTESIAN_POINT('Ctrl Pts',(0.974066058287501,1.,1.63820952658157));
#41728=CARTESIAN_POINT('Ctrl Pts',(0.977689794120296,-1.,1.64233990826831));
#41729=CARTESIAN_POINT('Ctrl Pts',(0.977689794120296,1.,1.64233990826831));
#41730=CARTESIAN_POINT('Ctrl Pts',(0.981562530940574,-1.,1.64665139190834));
#41731=CARTESIAN_POINT('Ctrl Pts',(0.981562530940574,1.,1.64665139190834));
#41732=CARTESIAN_POINT('Ctrl Pts',(0.985642622921626,-1.,1.6511001661277));
#41733=CARTESIAN_POINT('Ctrl Pts',(0.985642622921626,1.,1.6511001661277));
#41734=CARTESIAN_POINT('Ctrl Pts',(0.98985562785445,-1.,1.65559044289746));
#41735=CARTESIAN_POINT('Ctrl Pts',(0.98985562785445,1.,1.65559044289746));
#41736=CARTESIAN_POINT('Ctrl Pts',(0.994121836661115,-1.,1.66001553809916));
#41737=CARTESIAN_POINT('Ctrl Pts',(0.994121836661115,1.,1.66001553809916));
#41738=CARTESIAN_POINT('Ctrl Pts',(0.998389654952317,-1.,1.66430758030304));
#41739=CARTESIAN_POINT('Ctrl Pts',(0.998389654952317,1.,1.66430758030304));
#41740=CARTESIAN_POINT('Ctrl Pts',(1.00265091003682,-1.,1.66846059277231));
#41741=CARTESIAN_POINT('Ctrl Pts',(1.00265091003682,1.,1.66846059277231));
#41742=CARTESIAN_POINT('Ctrl Pts',(1.00692206696387,-1.,1.67250335383248));
#41743=CARTESIAN_POINT('Ctrl Pts',(1.00692206696387,1.,1.67250335383248));
#41744=CARTESIAN_POINT('Ctrl Pts',(1.01123236493507,-1.,1.67648246776457));
#41745=CARTESIAN_POINT('Ctrl Pts',(1.01123236493507,1.,1.67648246776457));
#41746=CARTESIAN_POINT('Ctrl Pts',(1.01561026162786,-1.,1.6804428989482));
#41747=CARTESIAN_POINT('Ctrl Pts',(1.01561026162786,1.,1.6804428989482));
#41748=CARTESIAN_POINT('Ctrl Pts',(1.02006795074222,-1.,1.68440578021739));
#41749=CARTESIAN_POINT('Ctrl Pts',(1.02006795074222,1.,1.68440578021739));
#41750=CARTESIAN_POINT('Ctrl Pts',(1.02460180535272,-1.,1.68836910178475));
#41751=CARTESIAN_POINT('Ctrl Pts',(1.02460180535272,1.,1.68836910178475));
#41752=CARTESIAN_POINT('Ctrl Pts',(1.02919977579155,-1.,1.69231840863471));
#41753=CARTESIAN_POINT('Ctrl Pts',(1.02919977579155,1.,1.69231840863471));
#41754=CARTESIAN_POINT('Ctrl Pts',(1.03384646003587,-1.,1.69623414782769));
#41755=CARTESIAN_POINT('Ctrl Pts',(1.03384646003587,1.,1.69623414782769));
#41756=CARTESIAN_POINT('Ctrl Pts',(1.03852922490782,-1.,1.70010052930951));
#41757=CARTESIAN_POINT('Ctrl Pts',(1.03852922490782,1.,1.70010052930951));
#41758=CARTESIAN_POINT('Ctrl Pts',(1.04324363334546,-1.,1.70391338707969));
#41759=CARTESIAN_POINT('Ctrl Pts',(1.04324363334546,1.,1.70391338707969));
#41760=CARTESIAN_POINT('Ctrl Pts',(1.0479908540499,-1.,1.70767646263641));
#41761=CARTESIAN_POINT('Ctrl Pts',(1.0479908540499,1.,1.70767646263641));
#41762=CARTESIAN_POINT('Ctrl Pts',(1.05277517202853,-1.,1.71139783543986));
#41763=CARTESIAN_POINT('Ctrl Pts',(1.05277517202853,1.,1.71139783543986));
#41764=CARTESIAN_POINT('Ctrl Pts',(1.05760163192481,-1.,1.71508654427022));
#41765=CARTESIAN_POINT('Ctrl Pts',(1.05760163192481,1.,1.71508654427022));
#41766=CARTESIAN_POINT('Ctrl Pts',(1.06247324680649,-1.,1.71874858456908));
#41767=CARTESIAN_POINT('Ctrl Pts',(1.06247324680649,1.,1.71874858456908));
#41768=CARTESIAN_POINT('Ctrl Pts',(1.06738966975463,-1.,1.72238500928456));
#41769=CARTESIAN_POINT('Ctrl Pts',(1.06738966975463,1.,1.72238500928456));
#41770=CARTESIAN_POINT('Ctrl Pts',(1.07234866990252,-1.,1.72599406198489));
#41771=CARTESIAN_POINT('Ctrl Pts',(1.07234866990252,1.,1.72599406198489));
#41772=CARTESIAN_POINT('Ctrl Pts',(1.0773470373727,-1.,1.72957248977424));
#41773=CARTESIAN_POINT('Ctrl Pts',(1.0773470373727,1.,1.72957248977424));
#41774=CARTESIAN_POINT('Ctrl Pts',(1.08238162784749,-1.,1.73311705663407));
#41775=CARTESIAN_POINT('Ctrl Pts',(1.08238162784749,1.,1.73311705663407));
#41776=CARTESIAN_POINT('Ctrl Pts',(1.08745056285429,-1.,1.73662628326093));
#41777=CARTESIAN_POINT('Ctrl Pts',(1.08745056285429,1.,1.73662628326093));
#41778=CARTESIAN_POINT('Ctrl Pts',(1.09255329056496,-1.,1.74010053962252));
#41779=CARTESIAN_POINT('Ctrl Pts',(1.09255329056496,1.,1.74010053962252));
#41780=CARTESIAN_POINT('Ctrl Pts',(1.09768999241229,-1.,1.74354119236212));
#41781=CARTESIAN_POINT('Ctrl Pts',(1.09768999241229,1.,1.74354119236212));
#41782=CARTESIAN_POINT('Ctrl Pts',(1.10286118991144,-1.,1.74695004214924));
#41783=CARTESIAN_POINT('Ctrl Pts',(1.10286118991144,1.,1.74695004214924));
#41784=CARTESIAN_POINT('Ctrl Pts',(1.10806728183003,-1.,1.75032866075914));
#41785=CARTESIAN_POINT('Ctrl Pts',(1.10806728183003,1.,1.75032866075914));
#41786=CARTESIAN_POINT('Ctrl Pts',(1.11330807582542,-1.,1.75367772094617));
#41787=CARTESIAN_POINT('Ctrl Pts',(1.11330807582542,1.,1.75367772094617));
#41788=CARTESIAN_POINT('Ctrl Pts',(1.11858293216752,-1.,1.75699720772089));
#41789=CARTESIAN_POINT('Ctrl Pts',(1.11858293216752,1.,1.75699720772089));
#41790=CARTESIAN_POINT('Ctrl Pts',(1.12389096855078,-1.,1.76028671825084));
#41791=CARTESIAN_POINT('Ctrl Pts',(1.12389096855078,1.,1.76028671825084));
#41792=CARTESIAN_POINT('Ctrl Pts',(1.12923123555076,-1.,1.76354571966171));
#41793=CARTESIAN_POINT('Ctrl Pts',(1.12923123555076,1.,1.76354571966171));
#41794=CARTESIAN_POINT('Ctrl Pts',(1.13460291804634,-1.,1.76677384551883));
#41795=CARTESIAN_POINT('Ctrl Pts',(1.13460291804634,1.,1.76677384551883));
#41796=CARTESIAN_POINT('Ctrl Pts',(1.14000548337,-1.,1.76997111386806));
#41797=CARTESIAN_POINT('Ctrl Pts',(1.14000548337,1.,1.76997111386806));
#41798=CARTESIAN_POINT('Ctrl Pts',(1.14543858226948,-1.,1.77313777896234));
#41799=CARTESIAN_POINT('Ctrl Pts',(1.14543858226948,1.,1.77313777896234));
#41800=CARTESIAN_POINT('Ctrl Pts',(1.15090197841531,-1.,1.77627422557034));
#41801=CARTESIAN_POINT('Ctrl Pts',(1.15090197841531,1.,1.77627422557034));
#41802=CARTESIAN_POINT('Ctrl Pts',(1.15639547194689,-1.,1.77938085564261));
#41803=CARTESIAN_POINT('Ctrl Pts',(1.15639547194689,1.,1.77938085564261));
#41804=CARTESIAN_POINT('Ctrl Pts',(1.16191881298458,-1.,1.78245795880949));
#41805=CARTESIAN_POINT('Ctrl Pts',(1.16191881298458,1.,1.78245795880949));
#41806=CARTESIAN_POINT('Ctrl Pts',(1.16747166312239,-1.,1.78550566040349));
#41807=CARTESIAN_POINT('Ctrl Pts',(1.16747166312239,1.,1.78550566040349));
#41808=CARTESIAN_POINT('Ctrl Pts',(1.17305363177265,-1.,1.78852398877523));
#41809=CARTESIAN_POINT('Ctrl Pts',(1.17305363177265,1.,1.78852398877523));
#41810=CARTESIAN_POINT('Ctrl Pts',(1.17866429440781,-1.,1.79151291552646));
#41811=CARTESIAN_POINT('Ctrl Pts',(1.17866429440781,1.,1.79151291552646));
#41812=CARTESIAN_POINT('Ctrl Pts',(1.18430321697471,-1.,1.79447240321572));
#41813=CARTESIAN_POINT('Ctrl Pts',(1.18430321697471,1.,1.79447240321572));
#41814=CARTESIAN_POINT('Ctrl Pts',(1.1899699793456,-1.,1.79740245923649));
#41815=CARTESIAN_POINT('Ctrl Pts',(1.1899699793456,1.,1.79740245923649));
#41816=CARTESIAN_POINT('Ctrl Pts',(1.19566418930405,-1.,1.80030314370121));
#41817=CARTESIAN_POINT('Ctrl Pts',(1.19566418930405,1.,1.80030314370121));
#41818=CARTESIAN_POINT('Ctrl Pts',(1.2013854893912,-1.,1.8031745483882));
#41819=CARTESIAN_POINT('Ctrl Pts',(1.2013854893912,1.,1.8031745483882));
#41820=CARTESIAN_POINT('Ctrl Pts',(1.20713356605519,-1.,1.80601678480772));
#41821=CARTESIAN_POINT('Ctrl Pts',(1.20713356605519,1.,1.80601678480772));
#41822=CARTESIAN_POINT('Ctrl Pts',(1.2129081570818,-1.,1.80882996916931));
#41823=CARTESIAN_POINT('Ctrl Pts',(1.2129081570818,1.,1.80882996916931));
#41824=CARTESIAN_POINT('Ctrl Pts',(1.2187090610323,-1.,1.81161420806172));
#41825=CARTESIAN_POINT('Ctrl Pts',(1.2187090610323,1.,1.81161420806172));
#41826=CARTESIAN_POINT('Ctrl Pts',(1.22453613304507,-1.,1.81436959209778));
#41827=CARTESIAN_POINT('Ctrl Pts',(1.22453613304507,1.,1.81436959209778));
#41828=CARTESIAN_POINT('Ctrl Pts',(1.22921864890975,-1.,1.81655087183054));
#41829=CARTESIAN_POINT('Ctrl Pts',(1.22921864890975,1.,1.81655087183054));
#41830=CARTESIAN_POINT('Ctrl Pts',(1.23274224526804,-1.,1.81817389920914));
#41831=CARTESIAN_POINT('Ctrl Pts',(1.23274224526804,1.,1.81817389920914));
#41832=CARTESIAN_POINT('Ctrl Pts',(1.23509651170384,-1.,1.81925017193531));
#41833=CARTESIAN_POINT('Ctrl Pts',(1.23509651170384,1.,1.81925017193531));
#41834=CARTESIAN_POINT('Ctrl Pts',(1.23627494547115,-1.,1.81978687191668));
#41835=CARTESIAN_POINT('Ctrl Pts',(1.23627494547115,1.,1.81978687191668));
#41836=CARTESIAN_POINT('',(0.892032620296855,1.,1.5055822144029));
#41837=CARTESIAN_POINT('Ctrl Pts',(0.892032620296855,1.,1.5055822144029));
#41838=CARTESIAN_POINT('Ctrl Pts',(0.894452006967538,1.,1.50980486807181));
#41839=CARTESIAN_POINT('Ctrl Pts',(0.89918504749193,1.,1.51805569591479));
#41840=CARTESIAN_POINT('Ctrl Pts',(0.905967409640498,1.,1.52984849890434));
#41841=CARTESIAN_POINT('Ctrl Pts',(0.914375919046579,1.,1.54440491152808));
#41842=CARTESIAN_POINT('Ctrl Pts',(0.923832188966322,1.,1.56065988582509));
#41843=CARTESIAN_POINT('Ctrl Pts',(0.932246680128848,1.,1.57499388385561));
#41844=CARTESIAN_POINT('Ctrl Pts',(0.939646377909319,1.,1.58744937489796));
#41845=CARTESIAN_POINT('Ctrl Pts',(0.946078063325795,1.,1.59810042045408));
#41846=CARTESIAN_POINT('Ctrl Pts',(0.951613284361247,1.,1.60706069897794));
#41847=CARTESIAN_POINT('Ctrl Pts',(0.956354422921572,1.,1.61449324337233));
#41848=CARTESIAN_POINT('Ctrl Pts',(0.960438326099958,1.,1.62061638139929));
#41849=CARTESIAN_POINT('Ctrl Pts',(0.964046107037821,1.,1.6257193066974));
#41850=CARTESIAN_POINT('Ctrl Pts',(0.967387853228041,1.,1.63013849959083));
#41851=CARTESIAN_POINT('Ctrl Pts',(0.970669715996356,1.,1.63420665729609));
#41852=CARTESIAN_POINT('Ctrl Pts',(0.974066058287501,1.,1.63820952658157));
#41853=CARTESIAN_POINT('Ctrl Pts',(0.977689794120296,1.,1.64233990826831));
#41854=CARTESIAN_POINT('Ctrl Pts',(0.981562530940574,1.,1.64665139190834));
#41855=CARTESIAN_POINT('Ctrl Pts',(0.985642622921626,1.,1.6511001661277));
#41856=CARTESIAN_POINT('Ctrl Pts',(0.98985562785445,1.,1.65559044289746));
#41857=CARTESIAN_POINT('Ctrl Pts',(0.994121836661115,1.,1.66001553809916));
#41858=CARTESIAN_POINT('Ctrl Pts',(0.998389654952317,1.,1.66430758030304));
#41859=CARTESIAN_POINT('Ctrl Pts',(1.00265091003682,1.,1.66846059277231));
#41860=CARTESIAN_POINT('Ctrl Pts',(1.00692206696387,1.,1.67250335383248));
#41861=CARTESIAN_POINT('Ctrl Pts',(1.01123236493507,1.,1.67648246776457));
#41862=CARTESIAN_POINT('Ctrl Pts',(1.01561026162786,1.,1.6804428989482));
#41863=CARTESIAN_POINT('Ctrl Pts',(1.02006795074222,1.,1.68440578021739));
#41864=CARTESIAN_POINT('Ctrl Pts',(1.02460180535272,1.,1.68836910178475));
#41865=CARTESIAN_POINT('Ctrl Pts',(1.02919977579155,1.,1.69231840863471));
#41866=CARTESIAN_POINT('Ctrl Pts',(1.03384646003587,1.,1.69623414782769));
#41867=CARTESIAN_POINT('Ctrl Pts',(1.03852922490782,1.,1.70010052930951));
#41868=CARTESIAN_POINT('Ctrl Pts',(1.04324363334546,1.,1.70391338707969));
#41869=CARTESIAN_POINT('Ctrl Pts',(1.0479908540499,1.,1.70767646263641));
#41870=CARTESIAN_POINT('Ctrl Pts',(1.05277517202853,1.,1.71139783543986));
#41871=CARTESIAN_POINT('Ctrl Pts',(1.05760163192481,1.,1.71508654427022));
#41872=CARTESIAN_POINT('Ctrl Pts',(1.06247324680649,1.,1.71874858456908));
#41873=CARTESIAN_POINT('Ctrl Pts',(1.06738966975463,1.,1.72238500928456));
#41874=CARTESIAN_POINT('Ctrl Pts',(1.07234866990252,1.,1.72599406198489));
#41875=CARTESIAN_POINT('Ctrl Pts',(1.0773470373727,1.,1.72957248977424));
#41876=CARTESIAN_POINT('Ctrl Pts',(1.08238162784749,1.,1.73311705663407));
#41877=CARTESIAN_POINT('Ctrl Pts',(1.08745056285429,1.,1.73662628326093));
#41878=CARTESIAN_POINT('Ctrl Pts',(1.09255329056496,1.,1.74010053962252));
#41879=CARTESIAN_POINT('Ctrl Pts',(1.09768999241229,1.,1.74354119236212));
#41880=CARTESIAN_POINT('Ctrl Pts',(1.10286118991144,1.,1.74695004214924));
#41881=CARTESIAN_POINT('Ctrl Pts',(1.10806728183003,1.,1.75032866075914));
#41882=CARTESIAN_POINT('Ctrl Pts',(1.11330807582542,1.,1.75367772094617));
#41883=CARTESIAN_POINT('Ctrl Pts',(1.11858293216752,1.,1.75699720772089));
#41884=CARTESIAN_POINT('Ctrl Pts',(1.12389096855078,1.,1.76028671825084));
#41885=CARTESIAN_POINT('Ctrl Pts',(1.12923123555076,1.,1.76354571966171));
#41886=CARTESIAN_POINT('Ctrl Pts',(1.13460291804634,1.,1.76677384551883));
#41887=CARTESIAN_POINT('Ctrl Pts',(1.14000548337,1.,1.76997111386806));
#41888=CARTESIAN_POINT('Ctrl Pts',(1.14543858226948,1.,1.77313777896234));
#41889=CARTESIAN_POINT('Ctrl Pts',(1.15090197841531,1.,1.77627422557034));
#41890=CARTESIAN_POINT('Ctrl Pts',(1.15639547194689,1.,1.77938085564261));
#41891=CARTESIAN_POINT('Ctrl Pts',(1.16191881298458,1.,1.78245795880949));
#41892=CARTESIAN_POINT('Ctrl Pts',(1.16747166312239,1.,1.78550566040349));
#41893=CARTESIAN_POINT('Ctrl Pts',(1.17305363177265,1.,1.78852398877523));
#41894=CARTESIAN_POINT('Ctrl Pts',(1.17866429440781,1.,1.79151291552646));
#41895=CARTESIAN_POINT('Ctrl Pts',(1.18430321697471,1.,1.79447240321572));
#41896=CARTESIAN_POINT('Ctrl Pts',(1.1899699793456,1.,1.79740245923649));
#41897=CARTESIAN_POINT('Ctrl Pts',(1.19566418930405,1.,1.80030314370121));
#41898=CARTESIAN_POINT('Ctrl Pts',(1.2013854893912,1.,1.8031745483882));
#41899=CARTESIAN_POINT('Ctrl Pts',(1.20713356605519,1.,1.80601678480772));
#41900=CARTESIAN_POINT('Ctrl Pts',(1.2129081570818,1.,1.80882996916931));
#41901=CARTESIAN_POINT('Ctrl Pts',(1.2187090610323,1.,1.81161420806172));
#41902=CARTESIAN_POINT('Ctrl Pts',(1.22453613304507,1.,1.81436959209778));
#41903=CARTESIAN_POINT('Ctrl Pts',(1.22921864890975,1.,1.81655087183054));
#41904=CARTESIAN_POINT('Ctrl Pts',(1.23274224526804,1.,1.81817389920914));
#41905=CARTESIAN_POINT('Ctrl Pts',(1.23509651170384,1.,1.81925017193531));
#41906=CARTESIAN_POINT('Ctrl Pts',(1.23627494547115,1.,1.81978687191668));
#41907=CARTESIAN_POINT('',(0.892032620296854,0.,1.5055822144029));
#41908=CARTESIAN_POINT('Origin',(0.,0.,0.));
#41909=CARTESIAN_POINT('',(0.693717979106305,1.,1.60662857109684));
#41910=CARTESIAN_POINT('Origin',(0.,1.,0.));
#41911=CARTESIAN_POINT('',(0.693717979106305,0.,1.60662857109684));
#41912=CARTESIAN_POINT('Ctrl Pts',(0.7455743247944,-1.,2.0698113262342));
#41913=CARTESIAN_POINT('Ctrl Pts',(0.7455743247944,1.,2.0698113262342));
#41914=CARTESIAN_POINT('Ctrl Pts',(0.745832791378367,-1.,2.06854248895728));
#41915=CARTESIAN_POINT('Ctrl Pts',(0.745832791378367,1.,2.06854248895728));
#41916=CARTESIAN_POINT('Ctrl Pts',(0.7463458715442,-1.,2.06600523016815));
#41917=CARTESIAN_POINT('Ctrl Pts',(0.7463458715442,1.,2.06600523016815));
#41918=CARTESIAN_POINT('Ctrl Pts',(0.747103932787919,-1.,2.06220058927826));
#41919=CARTESIAN_POINT('Ctrl Pts',(0.747103932787919,1.,2.06220058927826));
#41920=CARTESIAN_POINT('Ctrl Pts',(0.748091554183802,-1.,2.05713023031007));
#41921=CARTESIAN_POINT('Ctrl Pts',(0.748091554183802,1.,2.05713023031007));
#41922=CARTESIAN_POINT('Ctrl Pts',(0.749287468665046,-1.,2.05079645592154));
#41923=CARTESIAN_POINT('Ctrl Pts',(0.749287468665046,1.,2.05079645592154));
#41924=CARTESIAN_POINT('Ctrl Pts',(0.750444657875575,-1.,2.04446689147979));
#41925=CARTESIAN_POINT('Ctrl Pts',(0.750444657875575,1.,2.04446689147979));
#41926=CARTESIAN_POINT('Ctrl Pts',(0.751562963361115,-1.,2.03814160092099));
#41927=CARTESIAN_POINT('Ctrl Pts',(0.751562963361115,1.,2.03814160092099));
#41928=CARTESIAN_POINT('Ctrl Pts',(0.75264218048721,-1.,2.03182068456221));
#41929=CARTESIAN_POINT('Ctrl Pts',(0.75264218048721,1.,2.03182068456221));
#41930=CARTESIAN_POINT('Ctrl Pts',(0.753682061112768,-1.,2.02550428623313));
#41931=CARTESIAN_POINT('Ctrl Pts',(0.753682061112768,1.,2.02550428623313));
#41932=CARTESIAN_POINT('Ctrl Pts',(0.754682330722816,-1.,2.01919259405809));
#41933=CARTESIAN_POINT('Ctrl Pts',(0.754682330722816,1.,2.01919259405809));
#41934=CARTESIAN_POINT('Ctrl Pts',(0.755642704957865,-1.,2.01288584328084));
#41935=CARTESIAN_POINT('Ctrl Pts',(0.755642704957865,1.,2.01288584328084));
#41936=CARTESIAN_POINT('Ctrl Pts',(0.75656290464667,-1.,2.0065843158773));
#41937=CARTESIAN_POINT('Ctrl Pts',(0.75656290464667,1.,2.0065843158773));
#41938=CARTESIAN_POINT('Ctrl Pts',(0.757442676862724,-1.,2.00028834739178));
#41939=CARTESIAN_POINT('Ctrl Pts',(0.757442676862724,1.,2.00028834739178));
#41940=CARTESIAN_POINT('Ctrl Pts',(0.758281796766761,-1.,1.99399831098817));
#41941=CARTESIAN_POINT('Ctrl Pts',(0.758281796766761,1.,1.99399831098817));
#41942=CARTESIAN_POINT('Ctrl Pts',(0.759080037802488,-1.,1.98771456680874));
#41943=CARTESIAN_POINT('Ctrl Pts',(0.759080037802488,1.,1.98771456680874));
#41944=CARTESIAN_POINT('Ctrl Pts',(0.75983714745219,-1.,1.98143741418172));
#41945=CARTESIAN_POINT('Ctrl Pts',(0.75983714745219,1.,1.98143741418172));
#41946=CARTESIAN_POINT('Ctrl Pts',(0.760552825409757,-1.,1.97516705321494));
#41947=CARTESIAN_POINT('Ctrl Pts',(0.760552825409757,1.,1.97516705321494));
#41948=CARTESIAN_POINT('Ctrl Pts',(0.76122669048382,-1.,1.96890351582499));
#41949=CARTESIAN_POINT('Ctrl Pts',(0.76122669048382,1.,1.96890351582499));
#41950=CARTESIAN_POINT('Ctrl Pts',(0.761858300014423,-1.,1.96264672744186));
#41951=CARTESIAN_POINT('Ctrl Pts',(0.761858300014423,1.,1.96264672744186));
#41952=CARTESIAN_POINT('Ctrl Pts',(0.762447203806178,-1.,1.95639665309869));
#41953=CARTESIAN_POINT('Ctrl Pts',(0.762447203806178,1.,1.95639665309869));
#41954=CARTESIAN_POINT('Ctrl Pts',(0.762992990878769,-1.,1.95015342590024));
#41955=CARTESIAN_POINT('Ctrl Pts',(0.762992990878769,1.,1.95015342590024));
#41956=CARTESIAN_POINT('Ctrl Pts',(0.763495333538629,-1.,1.9439174661764));
#41957=CARTESIAN_POINT('Ctrl Pts',(0.763495333538629,1.,1.9439174661764));
#41958=CARTESIAN_POINT('Ctrl Pts',(0.763954049121458,-1.,1.93768964875886));
#41959=CARTESIAN_POINT('Ctrl Pts',(0.763954049121458,1.,1.93768964875886));
#41960=CARTESIAN_POINT('Ctrl Pts',(0.76436901067394,-1.,1.93147105496382));
#41961=CARTESIAN_POINT('Ctrl Pts',(0.76436901067394,1.,1.93147105496382));
#41962=CARTESIAN_POINT('Ctrl Pts',(0.764740025488211,-1.,1.92526263537048));
#41963=CARTESIAN_POINT('Ctrl Pts',(0.764740025488211,1.,1.92526263537048));
#41964=CARTESIAN_POINT('Ctrl Pts',(0.765066729667088,-1.,1.91906491634196));
#41965=CARTESIAN_POINT('Ctrl Pts',(0.765066729667088,1.,1.91906491634196));
#41966=CARTESIAN_POINT('Ctrl Pts',(0.765348465884722,-1.,1.91287765805169));
#41967=CARTESIAN_POINT('Ctrl Pts',(0.765348465884722,1.,1.91287765805169));
#41968=CARTESIAN_POINT('Ctrl Pts',(0.765584196937919,-1.,1.90669961402356));
#41969=CARTESIAN_POINT('Ctrl Pts',(0.765584196937919,1.,1.90669961402356));
#41970=CARTESIAN_POINT('Ctrl Pts',(0.765772772593386,-1.,1.90052930393596));
#41971=CARTESIAN_POINT('Ctrl Pts',(0.765772772593386,1.,1.90052930393596));
#41972=CARTESIAN_POINT('Ctrl Pts',(0.765913193856978,-1.,1.89436577771388));
#41973=CARTESIAN_POINT('Ctrl Pts',(0.765913193856978,1.,1.89436577771388));
#41974=CARTESIAN_POINT('Ctrl Pts',(0.766004837062091,-1.,1.88820926433409));
#41975=CARTESIAN_POINT('Ctrl Pts',(0.766004837062091,1.,1.88820926433409));
#41976=CARTESIAN_POINT('Ctrl Pts',(0.766047794851864,-1.,1.88206215302561));
#41977=CARTESIAN_POINT('Ctrl Pts',(0.766047794851864,1.,1.88206215302561));
#41978=CARTESIAN_POINT('Ctrl Pts',(0.766042837036744,-1.,1.87592888967883));
#41979=CARTESIAN_POINT('Ctrl Pts',(0.766042837036744,1.,1.87592888967883));
#41980=CARTESIAN_POINT('Ctrl Pts',(0.765990708546091,-1.,1.86981398314341));
#41981=CARTESIAN_POINT('Ctrl Pts',(0.765990708546091,1.,1.86981398314341));
#41982=CARTESIAN_POINT('Ctrl Pts',(0.765891519092547,-1.,1.86372027063312));
#41983=CARTESIAN_POINT('Ctrl Pts',(0.765891519092547,1.,1.86372027063312));
#41984=CARTESIAN_POINT('Ctrl Pts',(0.765744212909318,-1.,1.85764741390394));
#41985=CARTESIAN_POINT('Ctrl Pts',(0.765744212909318,1.,1.85764741390394));
#41986=CARTESIAN_POINT('Ctrl Pts',(0.765545710619062,-1.,1.85158945130063));
#41987=CARTESIAN_POINT('Ctrl Pts',(0.765545710619062,1.,1.85158945130063));
#41988=CARTESIAN_POINT('Ctrl Pts',(0.765291664862029,-1.,1.84553698875924));
#41989=CARTESIAN_POINT('Ctrl Pts',(0.765291664862029,1.,1.84553698875924));
#41990=CARTESIAN_POINT('Ctrl Pts',(0.764978057881737,-1.,1.83948181064835));
#41991=CARTESIAN_POINT('Ctrl Pts',(0.764978057881737,1.,1.83948181064835));
#41992=CARTESIAN_POINT('Ctrl Pts',(0.764602549687853,-1.,1.83342077227142));
#41993=CARTESIAN_POINT('Ctrl Pts',(0.764602549687853,1.,1.83342077227142));
#41994=CARTESIAN_POINT('Ctrl Pts',(0.764165902605995,-1.,1.82735991200065));
#41995=CARTESIAN_POINT('Ctrl Pts',(0.764165902605995,1.,1.82735991200065));
#41996=CARTESIAN_POINT('Ctrl Pts',(0.763673465462726,-1.,1.82131873145266));
#41997=CARTESIAN_POINT('Ctrl Pts',(0.763673465462726,1.,1.82131873145266));
#41998=CARTESIAN_POINT('Ctrl Pts',(0.763132003836634,-1.,1.8153211840553));
#41999=CARTESIAN_POINT('Ctrl Pts',(0.763132003836634,1.,1.8153211840553));
#42000=CARTESIAN_POINT('Ctrl Pts',(0.762546129463938,-1.,1.80938551463965));
#42001=CARTESIAN_POINT('Ctrl Pts',(0.762546129463938,1.,1.80938551463965));
#42002=CARTESIAN_POINT('Ctrl Pts',(0.761915336443547,-1.,1.80351583877342));
#42003=CARTESIAN_POINT('Ctrl Pts',(0.761915336443547,1.,1.80351583877342));
#42004=CARTESIAN_POINT('Ctrl Pts',(0.761229695230558,-1.,1.79768986997783));
#42005=CARTESIAN_POINT('Ctrl Pts',(0.761229695230558,1.,1.79768986997783));
#42006=CARTESIAN_POINT('Ctrl Pts',(0.760469555880749,-1.,1.7918581561088));
#42007=CARTESIAN_POINT('Ctrl Pts',(0.760469555880749,1.,1.7918581561088));
#42008=CARTESIAN_POINT('Ctrl Pts',(0.759614401110189,-1.,1.78596964884604));
#42009=CARTESIAN_POINT('Ctrl Pts',(0.759614401110189,1.,1.78596964884604));
#42010=CARTESIAN_POINT('Ctrl Pts',(0.758650626677518,-1.,1.77999411220945));
#42011=CARTESIAN_POINT('Ctrl Pts',(0.758650626677518,1.,1.77999411220945));
#42012=CARTESIAN_POINT('Ctrl Pts',(0.757578264077028,-1.,1.77394167108292));
#42013=CARTESIAN_POINT('Ctrl Pts',(0.757578264077028,1.,1.77394167108292));
#42014=CARTESIAN_POINT('Ctrl Pts',(0.75642189602781,-1.,1.76789396002998));
#42015=CARTESIAN_POINT('Ctrl Pts',(0.75642189602781,1.,1.76789396002998));
#42016=CARTESIAN_POINT('Ctrl Pts',(0.755220979974461,-1.,1.76197817240128));
#42017=CARTESIAN_POINT('Ctrl Pts',(0.755220979974461,1.,1.76197817240128));
#42018=CARTESIAN_POINT('Ctrl Pts',(0.754009254027828,-1.,1.75631083600019));
#42019=CARTESIAN_POINT('Ctrl Pts',(0.754009254027828,1.,1.75631083600019));
#42020=CARTESIAN_POINT('Ctrl Pts',(0.752797683531314,-1.,1.75095139468794));
#42021=CARTESIAN_POINT('Ctrl Pts',(0.752797683531314,1.,1.75095139468794));
#42022=CARTESIAN_POINT('Ctrl Pts',(0.751555614164482,-1.,1.74585086852502));
#42023=CARTESIAN_POINT('Ctrl Pts',(0.751555614164482,1.,1.74585086852502));
#42024=CARTESIAN_POINT('Ctrl Pts',(0.750193435981249,-1.,1.74080458267114));
#42025=CARTESIAN_POINT('Ctrl Pts',(0.750193435981249,1.,1.74080458267114));
#42026=CARTESIAN_POINT('Ctrl Pts',(0.74858246295687,-1.,1.7355035168033));
#42027=CARTESIAN_POINT('Ctrl Pts',(0.74858246295687,1.,1.7355035168033));
#42028=CARTESIAN_POINT('Ctrl Pts',(0.746574710097752,-1.,1.72958533647714));
#42029=CARTESIAN_POINT('Ctrl Pts',(0.746574710097752,1.,1.72958533647714));
#42030=CARTESIAN_POINT('Ctrl Pts',(0.744021445433093,-1.,1.72268229916769));
#42031=CARTESIAN_POINT('Ctrl Pts',(0.744021445433093,1.,1.72268229916769));
#42032=CARTESIAN_POINT('Ctrl Pts',(0.74079516202821,-1.,1.71447789751001));
#42033=CARTESIAN_POINT('Ctrl Pts',(0.74079516202821,1.,1.71447789751001));
#42034=CARTESIAN_POINT('Ctrl Pts',(0.736799665716932,-1.,1.70473309004249));
#42035=CARTESIAN_POINT('Ctrl Pts',(0.736799665716932,1.,1.70473309004249));
#42036=CARTESIAN_POINT('Ctrl Pts',(0.731963238685357,-1.,1.69326921972915));
#42037=CARTESIAN_POINT('Ctrl Pts',(0.731963238685357,1.,1.69326921972915));
#42038=CARTESIAN_POINT('Ctrl Pts',(0.726235967982445,-1.,1.67996158451922));
#42039=CARTESIAN_POINT('Ctrl Pts',(0.726235967982445,1.,1.67996158451922));
#42040=CARTESIAN_POINT('Ctrl Pts',(0.719585433787949,-1.,1.66472880551777));
#42041=CARTESIAN_POINT('Ctrl Pts',(0.719585433787949,1.,1.66472880551777));
#42042=CARTESIAN_POINT('Ctrl Pts',(0.711993139340447,-1.,1.64752408828442));
#42043=CARTESIAN_POINT('Ctrl Pts',(0.711993139340447,1.,1.64752408828442));
#42044=CARTESIAN_POINT('Ctrl Pts',(0.705159151977294,-1.,1.6321654166204));
#42045=CARTESIAN_POINT('Ctrl Pts',(0.705159151977294,1.,1.6321654166204));
#42046=CARTESIAN_POINT('Ctrl Pts',(0.699605146398836,-1.,1.61974673471117));
#42047=CARTESIAN_POINT('Ctrl Pts',(0.699605146398836,1.,1.61974673471117));
#42048=CARTESIAN_POINT('Ctrl Pts',(0.69571209787897,-1.,1.61106790957619));
#42049=CARTESIAN_POINT('Ctrl Pts',(0.69571209787897,1.,1.61106790957619));
#42050=CARTESIAN_POINT('Ctrl Pts',(0.693717979106305,-1.,1.60662857109684));
#42051=CARTESIAN_POINT('Ctrl Pts',(0.693717979106305,1.,1.60662857109684));
#42052=CARTESIAN_POINT('',(0.7455743247944,1.,2.0698113262342));
#42053=CARTESIAN_POINT('Ctrl Pts',(0.7455743247944,1.,2.0698113262342));
#42054=CARTESIAN_POINT('Ctrl Pts',(0.745832791378367,1.,2.06854248895728));
#42055=CARTESIAN_POINT('Ctrl Pts',(0.7463458715442,1.,2.06600523016815));
#42056=CARTESIAN_POINT('Ctrl Pts',(0.747103932787919,1.,2.06220058927826));
#42057=CARTESIAN_POINT('Ctrl Pts',(0.748091554183802,1.,2.05713023031007));
#42058=CARTESIAN_POINT('Ctrl Pts',(0.749287468665046,1.,2.05079645592154));
#42059=CARTESIAN_POINT('Ctrl Pts',(0.750444657875575,1.,2.04446689147979));
#42060=CARTESIAN_POINT('Ctrl Pts',(0.751562963361115,1.,2.03814160092099));
#42061=CARTESIAN_POINT('Ctrl Pts',(0.75264218048721,1.,2.03182068456221));
#42062=CARTESIAN_POINT('Ctrl Pts',(0.753682061112768,1.,2.02550428623313));
#42063=CARTESIAN_POINT('Ctrl Pts',(0.754682330722816,1.,2.01919259405809));
#42064=CARTESIAN_POINT('Ctrl Pts',(0.755642704957865,1.,2.01288584328084));
#42065=CARTESIAN_POINT('Ctrl Pts',(0.75656290464667,1.,2.0065843158773));
#42066=CARTESIAN_POINT('Ctrl Pts',(0.757442676862724,1.,2.00028834739178));
#42067=CARTESIAN_POINT('Ctrl Pts',(0.758281796766761,1.,1.99399831098817));
#42068=CARTESIAN_POINT('Ctrl Pts',(0.759080037802488,1.,1.98771456680874));
#42069=CARTESIAN_POINT('Ctrl Pts',(0.75983714745219,1.,1.98143741418172));
#42070=CARTESIAN_POINT('Ctrl Pts',(0.760552825409757,1.,1.97516705321494));
#42071=CARTESIAN_POINT('Ctrl Pts',(0.76122669048382,1.,1.96890351582499));
#42072=CARTESIAN_POINT('Ctrl Pts',(0.761858300014423,1.,1.96264672744186));
#42073=CARTESIAN_POINT('Ctrl Pts',(0.762447203806178,1.,1.95639665309869));
#42074=CARTESIAN_POINT('Ctrl Pts',(0.762992990878769,1.,1.95015342590024));
#42075=CARTESIAN_POINT('Ctrl Pts',(0.763495333538629,1.,1.9439174661764));
#42076=CARTESIAN_POINT('Ctrl Pts',(0.763954049121458,1.,1.93768964875886));
#42077=CARTESIAN_POINT('Ctrl Pts',(0.76436901067394,1.,1.93147105496382));
#42078=CARTESIAN_POINT('Ctrl Pts',(0.764740025488211,1.,1.92526263537048));
#42079=CARTESIAN_POINT('Ctrl Pts',(0.765066729667088,1.,1.91906491634196));
#42080=CARTESIAN_POINT('Ctrl Pts',(0.765348465884722,1.,1.91287765805169));
#42081=CARTESIAN_POINT('Ctrl Pts',(0.765584196937919,1.,1.90669961402356));
#42082=CARTESIAN_POINT('Ctrl Pts',(0.765772772593386,1.,1.90052930393596));
#42083=CARTESIAN_POINT('Ctrl Pts',(0.765913193856978,1.,1.89436577771388));
#42084=CARTESIAN_POINT('Ctrl Pts',(0.766004837062091,1.,1.88820926433409));
#42085=CARTESIAN_POINT('Ctrl Pts',(0.766047794851864,1.,1.88206215302561));
#42086=CARTESIAN_POINT('Ctrl Pts',(0.766042837036744,1.,1.87592888967883));
#42087=CARTESIAN_POINT('Ctrl Pts',(0.765990708546091,1.,1.86981398314341));
#42088=CARTESIAN_POINT('Ctrl Pts',(0.765891519092547,1.,1.86372027063312));
#42089=CARTESIAN_POINT('Ctrl Pts',(0.765744212909318,1.,1.85764741390394));
#42090=CARTESIAN_POINT('Ctrl Pts',(0.765545710619062,1.,1.85158945130063));
#42091=CARTESIAN_POINT('Ctrl Pts',(0.765291664862029,1.,1.84553698875924));
#42092=CARTESIAN_POINT('Ctrl Pts',(0.764978057881737,1.,1.83948181064835));
#42093=CARTESIAN_POINT('Ctrl Pts',(0.764602549687853,1.,1.83342077227142));
#42094=CARTESIAN_POINT('Ctrl Pts',(0.764165902605995,1.,1.82735991200065));
#42095=CARTESIAN_POINT('Ctrl Pts',(0.763673465462726,1.,1.82131873145266));
#42096=CARTESIAN_POINT('Ctrl Pts',(0.763132003836634,1.,1.8153211840553));
#42097=CARTESIAN_POINT('Ctrl Pts',(0.762546129463938,1.,1.80938551463965));
#42098=CARTESIAN_POINT('Ctrl Pts',(0.761915336443547,1.,1.80351583877342));
#42099=CARTESIAN_POINT('Ctrl Pts',(0.761229695230558,1.,1.79768986997783));
#42100=CARTESIAN_POINT('Ctrl Pts',(0.760469555880749,1.,1.7918581561088));
#42101=CARTESIAN_POINT('Ctrl Pts',(0.759614401110189,1.,1.78596964884604));
#42102=CARTESIAN_POINT('Ctrl Pts',(0.758650626677518,1.,1.77999411220945));
#42103=CARTESIAN_POINT('Ctrl Pts',(0.757578264077028,1.,1.77394167108292));
#42104=CARTESIAN_POINT('Ctrl Pts',(0.75642189602781,1.,1.76789396002998));
#42105=CARTESIAN_POINT('Ctrl Pts',(0.755220979974461,1.,1.76197817240128));
#42106=CARTESIAN_POINT('Ctrl Pts',(0.754009254027828,1.,1.75631083600019));
#42107=CARTESIAN_POINT('Ctrl Pts',(0.752797683531314,1.,1.75095139468794));
#42108=CARTESIAN_POINT('Ctrl Pts',(0.751555614164482,1.,1.74585086852502));
#42109=CARTESIAN_POINT('Ctrl Pts',(0.750193435981249,1.,1.74080458267114));
#42110=CARTESIAN_POINT('Ctrl Pts',(0.74858246295687,1.,1.7355035168033));
#42111=CARTESIAN_POINT('Ctrl Pts',(0.746574710097752,1.,1.72958533647714));
#42112=CARTESIAN_POINT('Ctrl Pts',(0.744021445433093,1.,1.72268229916769));
#42113=CARTESIAN_POINT('Ctrl Pts',(0.74079516202821,1.,1.71447789751001));
#42114=CARTESIAN_POINT('Ctrl Pts',(0.736799665716932,1.,1.70473309004249));
#42115=CARTESIAN_POINT('Ctrl Pts',(0.731963238685357,1.,1.69326921972915));
#42116=CARTESIAN_POINT('Ctrl Pts',(0.726235967982445,1.,1.67996158451922));
#42117=CARTESIAN_POINT('Ctrl Pts',(0.719585433787949,1.,1.66472880551777));
#42118=CARTESIAN_POINT('Ctrl Pts',(0.711993139340447,1.,1.64752408828442));
#42119=CARTESIAN_POINT('Ctrl Pts',(0.705159151977294,1.,1.6321654166204));
#42120=CARTESIAN_POINT('Ctrl Pts',(0.699605146398836,1.,1.61974673471117));
#42121=CARTESIAN_POINT('Ctrl Pts',(0.69571209787897,1.,1.61106790957619));
#42122=CARTESIAN_POINT('Ctrl Pts',(0.693717979106305,1.,1.60662857109684));
#42123=CARTESIAN_POINT('',(0.7455743247944,0.,2.0698113262342));
#42124=CARTESIAN_POINT('Origin',(0.61342227326009,0.,2.11275013067528));
#42125=CARTESIAN_POINT('',(0.61342227326009,1.,2.11275013067528));
#42126=CARTESIAN_POINT('',(0.7455743247944,1.,2.0698113262342));
#42127=CARTESIAN_POINT('',(0.61342227326009,0.,2.11275013067528));
#42128=CARTESIAN_POINT('Ctrl Pts',(0.383122945602004,-1.,1.7075470150345));
#42129=CARTESIAN_POINT('Ctrl Pts',(0.383122945602004,1.,1.7075470150345));
#42130=CARTESIAN_POINT('Ctrl Pts',(0.384119047315541,-1.,1.71231062891958));
#42131=CARTESIAN_POINT('Ctrl Pts',(0.384119047315541,1.,1.71231062891958));
#42132=CARTESIAN_POINT('Ctrl Pts',(0.38607079032701,-1.,1.72162022246158));
#42133=CARTESIAN_POINT('Ctrl Pts',(0.38607079032701,1.,1.72162022246158));
#42134=CARTESIAN_POINT('Ctrl Pts',(0.388877023509191,-1.,1.7349317097561));
#42135=CARTESIAN_POINT('Ctrl Pts',(0.388877023509191,1.,1.7349317097561));
#42136=CARTESIAN_POINT('Ctrl Pts',(0.392375812294307,-1.,1.75137405313962));
#42137=CARTESIAN_POINT('Ctrl Pts',(0.392375812294307,1.,1.75137405313962));
#42138=CARTESIAN_POINT('Ctrl Pts',(0.39634619612042,-1.,1.7697556004756));
#42139=CARTESIAN_POINT('Ctrl Pts',(0.39634619612042,1.,1.7697556004756));
#42140=CARTESIAN_POINT('Ctrl Pts',(0.39991940378308,-1.,1.78598826347533));
#42141=CARTESIAN_POINT('Ctrl Pts',(0.39991940378308,1.,1.78598826347533));
#42142=CARTESIAN_POINT('Ctrl Pts',(0.403107976170441,-1.,1.80012077176221));
#42143=CARTESIAN_POINT('Ctrl Pts',(0.403107976170441,1.,1.80012077176221));
#42144=CARTESIAN_POINT('Ctrl Pts',(0.405933518411838,-1.,1.81223801813988));
#42145=CARTESIAN_POINT('Ctrl Pts',(0.405933518411838,1.,1.81223801813988));
#42146=CARTESIAN_POINT('Ctrl Pts',(0.408428948108533,-1.,1.8224702267854));
#42147=CARTESIAN_POINT('Ctrl Pts',(0.408428948108533,1.,1.8224702267854));
#42148=CARTESIAN_POINT('Ctrl Pts',(0.410641256301674,-1.,1.83100408895216));
#42149=CARTESIAN_POINT('Ctrl Pts',(0.410641256301674,1.,1.83100408895216));
#42150=CARTESIAN_POINT('Ctrl Pts',(0.412633125322161,-1.,1.83808953475839));
#42151=CARTESIAN_POINT('Ctrl Pts',(0.412633125322161,1.,1.83808953475839));
#42152=CARTESIAN_POINT('Ctrl Pts',(0.41448743825434,-1.,1.8440575707371));
#42153=CARTESIAN_POINT('Ctrl Pts',(0.41448743825434,1.,1.8440575707371));
#42154=CARTESIAN_POINT('Ctrl Pts',(0.416300022038864,-1.,1.84929312929882));
#42155=CARTESIAN_POINT('Ctrl Pts',(0.416300022038864,1.,1.84929312929882));
#42156=CARTESIAN_POINT('Ctrl Pts',(0.418164129143534,-1.,1.85417632856234));
#42157=CARTESIAN_POINT('Ctrl Pts',(0.418164129143534,1.,1.85417632856234));
#42158=CARTESIAN_POINT('Ctrl Pts',(0.420157287975619,-1.,1.85903281096686));
#42159=CARTESIAN_POINT('Ctrl Pts',(0.420157287975619,1.,1.85903281096686));
#42160=CARTESIAN_POINT('Ctrl Pts',(0.422327307418275,-1.,1.86408083334028));
#42161=CARTESIAN_POINT('Ctrl Pts',(0.422327307418275,1.,1.86408083334028));
#42162=CARTESIAN_POINT('Ctrl Pts',(0.424678177291358,-1.,1.86937803944323));
#42163=CARTESIAN_POINT('Ctrl Pts',(0.424678177291358,1.,1.86937803944323));
#42164=CARTESIAN_POINT('Ctrl Pts',(0.427183828519102,-1.,1.87486989291484));
#42165=CARTESIAN_POINT('Ctrl Pts',(0.427183828519102,1.,1.87486989291484));
#42166=CARTESIAN_POINT('Ctrl Pts',(0.429803062482344,-1.,1.88044229001832));
#42167=CARTESIAN_POINT('Ctrl Pts',(0.429803062482344,1.,1.88044229001832));
#42168=CARTESIAN_POINT('Ctrl Pts',(0.432493038548748,-1.,1.88596913666793));
#42169=CARTESIAN_POINT('Ctrl Pts',(0.432493038548748,1.,1.88596913666793));
#42170=CARTESIAN_POINT('Ctrl Pts',(0.435225660963383,-1.,1.89136993975504));
#42171=CARTESIAN_POINT('Ctrl Pts',(0.435225660963383,1.,1.89136993975504));
#42172=CARTESIAN_POINT('Ctrl Pts',(0.437995003948244,-1.,1.89663648956466));
#42173=CARTESIAN_POINT('Ctrl Pts',(0.437995003948244,1.,1.89663648956466));
#42174=CARTESIAN_POINT('Ctrl Pts',(0.440807833704038,-1.,1.90180124389086));
#42175=CARTESIAN_POINT('Ctrl Pts',(0.440807833704038,1.,1.90180124389086));
#42176=CARTESIAN_POINT('Ctrl Pts',(0.44367755684915,-1.,1.90691756144898));
#42177=CARTESIAN_POINT('Ctrl Pts',(0.44367755684915,1.,1.90691756144898));
#42178=CARTESIAN_POINT('Ctrl Pts',(0.446617343485711,-1.,1.9120369998112));
#42179=CARTESIAN_POINT('Ctrl Pts',(0.446617343485711,1.,1.9120369998112));
#42180=CARTESIAN_POINT('Ctrl Pts',(0.449632260106662,-1.,1.91718342555755));
#42181=CARTESIAN_POINT('Ctrl Pts',(0.449632260106662,1.,1.91718342555755));
#42182=CARTESIAN_POINT('Ctrl Pts',(0.452719478359432,-1.,1.92235380648502));
#42183=CARTESIAN_POINT('Ctrl Pts',(0.452719478359432,1.,1.92235380648502));
#42184=CARTESIAN_POINT('Ctrl Pts',(0.45587200517437,-1.,1.92753067150476));
#42185=CARTESIAN_POINT('Ctrl Pts',(0.45587200517437,1.,1.92753067150476));
#42186=CARTESIAN_POINT('Ctrl Pts',(0.459081234547926,-1.,1.93269066517934));
#42187=CARTESIAN_POINT('Ctrl Pts',(0.459081234547926,1.,1.93269066517934));
#42188=CARTESIAN_POINT('Ctrl Pts',(0.462340031009056,-1.,1.93781486640821));
#42189=CARTESIAN_POINT('Ctrl Pts',(0.462340031009056,1.,1.93781486640821));
#42190=CARTESIAN_POINT('Ctrl Pts',(0.46564546202603,-1.,1.9428979419619));
#42191=CARTESIAN_POINT('Ctrl Pts',(0.46564546202603,1.,1.9428979419619));
#42192=CARTESIAN_POINT('Ctrl Pts',(0.468997482913135,-1.,1.94794381136514));
#42193=CARTESIAN_POINT('Ctrl Pts',(0.468997482913135,1.,1.94794381136514));
#42194=CARTESIAN_POINT('Ctrl Pts',(0.472397672264072,-1.,1.95296148278133));
#42195=CARTESIAN_POINT('Ctrl Pts',(0.472397672264072,1.,1.95296148278133));
#42196=CARTESIAN_POINT('Ctrl Pts',(0.475848034683176,-1.,1.95796111148177));
#42197=CARTESIAN_POINT('Ctrl Pts',(0.475848034683176,1.,1.95796111148177));
#42198=CARTESIAN_POINT('Ctrl Pts',(0.479349583074855,-1.,1.96294933055943));
#42199=CARTESIAN_POINT('Ctrl Pts',(0.479349583074855,1.,1.96294933055943));
#42200=CARTESIAN_POINT('Ctrl Pts',(0.48290166212069,-1.,1.96792703422362));
#42201=CARTESIAN_POINT('Ctrl Pts',(0.48290166212069,1.,1.96792703422362));
#42202=CARTESIAN_POINT('Ctrl Pts',(0.486502692907658,-1.,1.97289186263272));
#42203=CARTESIAN_POINT('Ctrl Pts',(0.486502692907658,1.,1.97289186263272));
#42204=CARTESIAN_POINT('Ctrl Pts',(0.490150627860952,-1.,1.97783973019229));
#42205=CARTESIAN_POINT('Ctrl Pts',(0.490150627860952,1.,1.97783973019229));
#42206=CARTESIAN_POINT('Ctrl Pts',(0.493843476541494,-1.,1.98276658761821));
#42207=CARTESIAN_POINT('Ctrl Pts',(0.493843476541494,1.,1.98276658761821));
#42208=CARTESIAN_POINT('Ctrl Pts',(0.497579909545574,-1.,1.98767044752932));
#42209=CARTESIAN_POINT('Ctrl Pts',(0.497579909545574,1.,1.98767044752932));
#42210=CARTESIAN_POINT('Ctrl Pts',(0.501359287727146,-1.,1.99255149126155));
#42211=CARTESIAN_POINT('Ctrl Pts',(0.501359287727146,1.,1.99255149126155));
#42212=CARTESIAN_POINT('Ctrl Pts',(0.505181361323026,-1.,1.99741107463572));
#42213=CARTESIAN_POINT('Ctrl Pts',(0.505181361323026,1.,1.99741107463572));
#42214=CARTESIAN_POINT('Ctrl Pts',(0.509046069886157,-1.,2.00225107134734));
#42215=CARTESIAN_POINT('Ctrl Pts',(0.509046069886157,1.,2.00225107134734));
#42216=CARTESIAN_POINT('Ctrl Pts',(0.512953306961792,-1.,2.00707309946949));
#42217=CARTESIAN_POINT('Ctrl Pts',(0.512953306961792,1.,2.00707309946949));
#42218=CARTESIAN_POINT('Ctrl Pts',(0.516902681728687,-1.,2.01187773939242));
#42219=CARTESIAN_POINT('Ctrl Pts',(0.516902681728687,1.,2.01187773939242));
#42220=CARTESIAN_POINT('Ctrl Pts',(0.52089359039937,-1.,2.01666477917286));
#42221=CARTESIAN_POINT('Ctrl Pts',(0.52089359039937,1.,2.01666477917286));
#42222=CARTESIAN_POINT('Ctrl Pts',(0.524925318333476,-1.,2.02143356304698));
#42223=CARTESIAN_POINT('Ctrl Pts',(0.524925318333476,1.,2.02143356304698));
#42224=CARTESIAN_POINT('Ctrl Pts',(0.528997127241914,-1.,2.0261832908329));
#42225=CARTESIAN_POINT('Ctrl Pts',(0.528997127241914,1.,2.0261832908329));
#42226=CARTESIAN_POINT('Ctrl Pts',(0.533108355132976,-1.,2.03091336214426));
#42227=CARTESIAN_POINT('Ctrl Pts',(0.533108355132976,1.,2.03091336214426));
#42228=CARTESIAN_POINT('Ctrl Pts',(0.537258489833262,-1.,2.03562362954037));
#42229=CARTESIAN_POINT('Ctrl Pts',(0.537258489833262,1.,2.03562362954037));
#42230=CARTESIAN_POINT('Ctrl Pts',(0.541447120615659,-1.,2.04031422690527));
#42231=CARTESIAN_POINT('Ctrl Pts',(0.541447120615659,1.,2.04031422690527));
#42232=CARTESIAN_POINT('Ctrl Pts',(0.54567390381743,-1.,2.04498544714588));
#42233=CARTESIAN_POINT('Ctrl Pts',(0.54567390381743,1.,2.04498544714588));
#42234=CARTESIAN_POINT('Ctrl Pts',(0.549938525150295,-1.,2.04963761077958));
#42235=CARTESIAN_POINT('Ctrl Pts',(0.549938525150295,1.,2.04963761077958));
#42236=CARTESIAN_POINT('Ctrl Pts',(0.554240657463906,-1.,2.05427091604413));
#42237=CARTESIAN_POINT('Ctrl Pts',(0.554240657463906,1.,2.05427091604413));
#42238=CARTESIAN_POINT('Ctrl Pts',(0.558579940185151,-1.,2.05888537756462));
#42239=CARTESIAN_POINT('Ctrl Pts',(0.558579940185151,1.,2.05888537756462));
#42240=CARTESIAN_POINT('Ctrl Pts',(0.562955993082261,-1.,2.06348090160589));
#42241=CARTESIAN_POINT('Ctrl Pts',(0.562955993082261,1.,2.06348090160589));
#42242=CARTESIAN_POINT('Ctrl Pts',(0.567368421181087,-1.,2.06805732997334));
#42243=CARTESIAN_POINT('Ctrl Pts',(0.567368421181087,1.,2.06805732997334));
#42244=CARTESIAN_POINT('Ctrl Pts',(0.571816823242602,-1.,2.07261449292824));
#42245=CARTESIAN_POINT('Ctrl Pts',(0.571816823242602,1.,2.07261449292824));
#42246=CARTESIAN_POINT('Ctrl Pts',(0.576300797416844,-1.,2.07715226767559));
#42247=CARTESIAN_POINT('Ctrl Pts',(0.576300797416844,1.,2.07715226767559));
#42248=CARTESIAN_POINT('Ctrl Pts',(0.580819952108063,-1.,2.08167059018418));
#42249=CARTESIAN_POINT('Ctrl Pts',(0.580819952108063,1.,2.08167059018418));
#42250=CARTESIAN_POINT('Ctrl Pts',(0.585373918991617,-1.,2.08616943727951));
#42251=CARTESIAN_POINT('Ctrl Pts',(0.585373918991617,1.,2.08616943727951));
#42252=CARTESIAN_POINT('Ctrl Pts',(0.589962365403406,-1.,2.09064881812129));
#42253=CARTESIAN_POINT('Ctrl Pts',(0.589962365403406,1.,2.09064881812129));
#42254=CARTESIAN_POINT('Ctrl Pts',(0.594585006052162,-1.,2.0951087622027));
#42255=CARTESIAN_POINT('Ctrl Pts',(0.594585006052162,1.,2.0951087622027));
#42256=CARTESIAN_POINT('Ctrl Pts',(0.599241616420533,-1.,2.0995493086477));
#42257=CARTESIAN_POINT('Ctrl Pts',(0.599241616420533,1.,2.0995493086477));
#42258=CARTESIAN_POINT('Ctrl Pts',(0.60393203073603,-1.,2.10397049886949));
#42259=CARTESIAN_POINT('Ctrl Pts',(0.60393203073603,1.,2.10397049886949));
#42260=CARTESIAN_POINT('Ctrl Pts',(0.607711315454876,-1.,2.1074919961518));
#42261=CARTESIAN_POINT('Ctrl Pts',(0.607711315454876,1.,2.1074919961518));
#42262=CARTESIAN_POINT('Ctrl Pts',(0.610560911689898,-1.,2.11012443807238));
#42263=CARTESIAN_POINT('Ctrl Pts',(0.610560911689898,1.,2.11012443807238));
#42264=CARTESIAN_POINT('Ctrl Pts',(0.6124673655618,-1.,2.11187554259986));
#42265=CARTESIAN_POINT('Ctrl Pts',(0.6124673655618,1.,2.11187554259986));
#42266=CARTESIAN_POINT('Ctrl Pts',(0.61342227326009,-1.,2.11275013067528));
#42267=CARTESIAN_POINT('Ctrl Pts',(0.61342227326009,1.,2.11275013067528));
#42268=CARTESIAN_POINT('',(0.383122945602004,1.,1.7075470150345));
#42269=CARTESIAN_POINT('Ctrl Pts',(0.383122945602004,1.,1.7075470150345));
#42270=CARTESIAN_POINT('Ctrl Pts',(0.384119047315541,1.,1.71231062891958));
#42271=CARTESIAN_POINT('Ctrl Pts',(0.38607079032701,1.,1.72162022246158));
#42272=CARTESIAN_POINT('Ctrl Pts',(0.388877023509191,1.,1.7349317097561));
#42273=CARTESIAN_POINT('Ctrl Pts',(0.392375812294307,1.,1.75137405313962));
#42274=CARTESIAN_POINT('Ctrl Pts',(0.39634619612042,1.,1.7697556004756));
#42275=CARTESIAN_POINT('Ctrl Pts',(0.39991940378308,1.,1.78598826347533));
#42276=CARTESIAN_POINT('Ctrl Pts',(0.403107976170441,1.,1.80012077176221));
#42277=CARTESIAN_POINT('Ctrl Pts',(0.405933518411838,1.,1.81223801813988));
#42278=CARTESIAN_POINT('Ctrl Pts',(0.408428948108533,1.,1.8224702267854));
#42279=CARTESIAN_POINT('Ctrl Pts',(0.410641256301674,1.,1.83100408895216));
#42280=CARTESIAN_POINT('Ctrl Pts',(0.412633125322161,1.,1.83808953475839));
#42281=CARTESIAN_POINT('Ctrl Pts',(0.41448743825434,1.,1.8440575707371));
#42282=CARTESIAN_POINT('Ctrl Pts',(0.416300022038864,1.,1.84929312929882));
#42283=CARTESIAN_POINT('Ctrl Pts',(0.418164129143534,1.,1.85417632856234));
#42284=CARTESIAN_POINT('Ctrl Pts',(0.420157287975619,1.,1.85903281096686));
#42285=CARTESIAN_POINT('Ctrl Pts',(0.422327307418275,1.,1.86408083334028));
#42286=CARTESIAN_POINT('Ctrl Pts',(0.424678177291358,1.,1.86937803944323));
#42287=CARTESIAN_POINT('Ctrl Pts',(0.427183828519102,1.,1.87486989291484));
#42288=CARTESIAN_POINT('Ctrl Pts',(0.429803062482344,1.,1.88044229001832));
#42289=CARTESIAN_POINT('Ctrl Pts',(0.432493038548748,1.,1.88596913666793));
#42290=CARTESIAN_POINT('Ctrl Pts',(0.435225660963383,1.,1.89136993975504));
#42291=CARTESIAN_POINT('Ctrl Pts',(0.437995003948244,1.,1.89663648956466));
#42292=CARTESIAN_POINT('Ctrl Pts',(0.440807833704038,1.,1.90180124389086));
#42293=CARTESIAN_POINT('Ctrl Pts',(0.44367755684915,1.,1.90691756144898));
#42294=CARTESIAN_POINT('Ctrl Pts',(0.446617343485711,1.,1.9120369998112));
#42295=CARTESIAN_POINT('Ctrl Pts',(0.449632260106662,1.,1.91718342555755));
#42296=CARTESIAN_POINT('Ctrl Pts',(0.452719478359432,1.,1.92235380648502));
#42297=CARTESIAN_POINT('Ctrl Pts',(0.45587200517437,1.,1.92753067150476));
#42298=CARTESIAN_POINT('Ctrl Pts',(0.459081234547926,1.,1.93269066517934));
#42299=CARTESIAN_POINT('Ctrl Pts',(0.462340031009056,1.,1.93781486640821));
#42300=CARTESIAN_POINT('Ctrl Pts',(0.46564546202603,1.,1.9428979419619));
#42301=CARTESIAN_POINT('Ctrl Pts',(0.468997482913135,1.,1.94794381136514));
#42302=CARTESIAN_POINT('Ctrl Pts',(0.472397672264072,1.,1.95296148278133));
#42303=CARTESIAN_POINT('Ctrl Pts',(0.475848034683176,1.,1.95796111148177));
#42304=CARTESIAN_POINT('Ctrl Pts',(0.479349583074855,1.,1.96294933055943));
#42305=CARTESIAN_POINT('Ctrl Pts',(0.48290166212069,1.,1.96792703422362));
#42306=CARTESIAN_POINT('Ctrl Pts',(0.486502692907658,1.,1.97289186263272));
#42307=CARTESIAN_POINT('Ctrl Pts',(0.490150627860952,1.,1.97783973019229));
#42308=CARTESIAN_POINT('Ctrl Pts',(0.493843476541494,1.,1.98276658761821));
#42309=CARTESIAN_POINT('Ctrl Pts',(0.497579909545574,1.,1.98767044752932));
#42310=CARTESIAN_POINT('Ctrl Pts',(0.501359287727146,1.,1.99255149126155));
#42311=CARTESIAN_POINT('Ctrl Pts',(0.505181361323026,1.,1.99741107463572));
#42312=CARTESIAN_POINT('Ctrl Pts',(0.509046069886157,1.,2.00225107134734));
#42313=CARTESIAN_POINT('Ctrl Pts',(0.512953306961792,1.,2.00707309946949));
#42314=CARTESIAN_POINT('Ctrl Pts',(0.516902681728687,1.,2.01187773939242));
#42315=CARTESIAN_POINT('Ctrl Pts',(0.52089359039937,1.,2.01666477917286));
#42316=CARTESIAN_POINT('Ctrl Pts',(0.524925318333476,1.,2.02143356304698));
#42317=CARTESIAN_POINT('Ctrl Pts',(0.528997127241914,1.,2.0261832908329));
#42318=CARTESIAN_POINT('Ctrl Pts',(0.533108355132976,1.,2.03091336214426));
#42319=CARTESIAN_POINT('Ctrl Pts',(0.537258489833262,1.,2.03562362954037));
#42320=CARTESIAN_POINT('Ctrl Pts',(0.541447120615659,1.,2.04031422690527));
#42321=CARTESIAN_POINT('Ctrl Pts',(0.54567390381743,1.,2.04498544714588));
#42322=CARTESIAN_POINT('Ctrl Pts',(0.549938525150295,1.,2.04963761077958));
#42323=CARTESIAN_POINT('Ctrl Pts',(0.554240657463906,1.,2.05427091604413));
#42324=CARTESIAN_POINT('Ctrl Pts',(0.558579940185151,1.,2.05888537756462));
#42325=CARTESIAN_POINT('Ctrl Pts',(0.562955993082261,1.,2.06348090160589));
#42326=CARTESIAN_POINT('Ctrl Pts',(0.567368421181087,1.,2.06805732997334));
#42327=CARTESIAN_POINT('Ctrl Pts',(0.571816823242602,1.,2.07261449292824));
#42328=CARTESIAN_POINT('Ctrl Pts',(0.576300797416844,1.,2.07715226767559));
#42329=CARTESIAN_POINT('Ctrl Pts',(0.580819952108063,1.,2.08167059018418));
#42330=CARTESIAN_POINT('Ctrl Pts',(0.585373918991617,1.,2.08616943727951));
#42331=CARTESIAN_POINT('Ctrl Pts',(0.589962365403406,1.,2.09064881812129));
#42332=CARTESIAN_POINT('Ctrl Pts',(0.594585006052162,1.,2.0951087622027));
#42333=CARTESIAN_POINT('Ctrl Pts',(0.599241616420533,1.,2.0995493086477));
#42334=CARTESIAN_POINT('Ctrl Pts',(0.60393203073603,1.,2.10397049886949));
#42335=CARTESIAN_POINT('Ctrl Pts',(0.607711315454876,1.,2.1074919961518));
#42336=CARTESIAN_POINT('Ctrl Pts',(0.610560911689898,1.,2.11012443807238));
#42337=CARTESIAN_POINT('Ctrl Pts',(0.6124673655618,1.,2.11187554259986));
#42338=CARTESIAN_POINT('Ctrl Pts',(0.61342227326009,1.,2.11275013067528));
#42339=CARTESIAN_POINT('',(0.383122945602003,0.,1.7075470150345));
#42340=CARTESIAN_POINT('Origin',(0.,0.,0.));
#42341=CARTESIAN_POINT('',(0.163289472382896,1.,1.74236521665491));
#42342=CARTESIAN_POINT('Origin',(0.,1.,0.));
#42343=CARTESIAN_POINT('',(0.163289472382896,0.,1.74236521665491));
#42344=CARTESIAN_POINT('Ctrl Pts',(0.0694764450219578,-1.,2.19890268624765));
#42345=CARTESIAN_POINT('Ctrl Pts',(0.0694764450219578,1.,2.19890268624765));
#42346=CARTESIAN_POINT('Ctrl Pts',(0.0701143536325487,-1.,2.19777582085423));
#42347=CARTESIAN_POINT('Ctrl Pts',(0.0701143536325487,1.,2.19777582085423));
#42348=CARTESIAN_POINT('Ctrl Pts',(0.0713863779526151,-1.,2.19552129484002));
#42349=CARTESIAN_POINT('Ctrl Pts',(0.0713863779526151,1.,2.19552129484002));
#42350=CARTESIAN_POINT('Ctrl Pts',(0.0732830357306722,-1.,2.19213712013662));
#42351=CARTESIAN_POINT('Ctrl Pts',(0.0732830357306722,1.,2.19213712013662));
#42352=CARTESIAN_POINT('Ctrl Pts',(0.0757891465836145,-1.,2.1876201139953));
#42353=CARTESIAN_POINT('Ctrl Pts',(0.0757891465836145,1.,2.1876201139953));
#42354=CARTESIAN_POINT('Ctrl Pts',(0.078883772768524,-1.,2.18196589448887));
#42355=CARTESIAN_POINT('Ctrl Pts',(0.078883772768524,1.,2.18196589448887));
#42356=CARTESIAN_POINT('Ctrl Pts',(0.0819402680872763,-1.,2.176303712113));
#42357=CARTESIAN_POINT('Ctrl Pts',(0.0819402680872763,1.,2.176303712113));
#42358=CARTESIAN_POINT('Ctrl Pts',(0.084958462083537,-1.,2.17063357870952));
#42359=CARTESIAN_POINT('Ctrl Pts',(0.084958462083537,1.,2.17063357870952));
#42360=CARTESIAN_POINT('Ctrl Pts',(0.087938129138692,-1.,2.16495552645014));
#42361=CARTESIAN_POINT('Ctrl Pts',(0.087938129138692,1.,2.16495552645014));
#42362=CARTESIAN_POINT('Ctrl Pts',(0.0908789888107263,-1.,2.15926961544516));
#42363=CARTESIAN_POINT('Ctrl Pts',(0.0908789888107263,1.,2.15926961544516));
#42364=CARTESIAN_POINT('Ctrl Pts',(0.0937807218867641,-1.,2.1535759397817));
#42365=CARTESIAN_POINT('Ctrl Pts',(0.0937807218867641,1.,2.1535759397817));
#42366=CARTESIAN_POINT('Ctrl Pts',(0.0966429852305456,-1.,2.14787463531795));
#42367=CARTESIAN_POINT('Ctrl Pts',(0.0966429852305456,1.,2.14787463531795));
#42368=CARTESIAN_POINT('Ctrl Pts',(0.0994654261990913,-1.,2.14216588396025));
#42369=CARTESIAN_POINT('Ctrl Pts',(0.0994654261990913,1.,2.14216588396025));
#42370=CARTESIAN_POINT('Ctrl Pts',(0.1022477005561,-1.,2.13644992667165));
#42371=CARTESIAN_POINT('Ctrl Pts',(0.1022477005561,1.,2.13644992667165));
#42372=CARTESIAN_POINT('Ctrl Pts',(0.104989479152739,-1.,2.13072704887293));
#42373=CARTESIAN_POINT('Ctrl Pts',(0.104989479152739,1.,2.13072704887293));
#42374=CARTESIAN_POINT('Ctrl Pts',(0.10769043523109,-1.,2.12499752307));
#42375=CARTESIAN_POINT('Ctrl Pts',(0.10769043523109,1.,2.12499752307));
#42376=CARTESIAN_POINT('Ctrl Pts',(0.110350236135025,-1.,2.11926155590865));
#42377=CARTESIAN_POINT('Ctrl Pts',(0.110350236135025,1.,2.11926155590865));
#42378=CARTESIAN_POINT('Ctrl Pts',(0.112968534419737,-1.,2.11351924490306));
#42379=CARTESIAN_POINT('Ctrl Pts',(0.112968534419737,1.,2.11351924490306));
#42380=CARTESIAN_POINT('Ctrl Pts',(0.115544957687926,-1.,2.10777050261309));
#42381=CARTESIAN_POINT('Ctrl Pts',(0.115544957687926,1.,2.10777050261309));
#42382=CARTESIAN_POINT('Ctrl Pts',(0.118079107988355,-1.,2.102015121329));
#42383=CARTESIAN_POINT('Ctrl Pts',(0.118079107988355,1.,2.102015121329));
#42384=CARTESIAN_POINT('Ctrl Pts',(0.120570567965122,-1.,2.0962529286773));
#42385=CARTESIAN_POINT('Ctrl Pts',(0.120570567965122,1.,2.0962529286773));
#42386=CARTESIAN_POINT('Ctrl Pts',(0.123018905621083,-1.,2.09048392424825));
#42387=CARTESIAN_POINT('Ctrl Pts',(0.123018905621083,1.,2.09048392424825));
#42388=CARTESIAN_POINT('Ctrl Pts',(0.125423679412061,-1.,2.08470840653643));
#42389=CARTESIAN_POINT('Ctrl Pts',(0.125423679412061,1.,2.08470840653643));
#42390=CARTESIAN_POINT('Ctrl Pts',(0.12778444527612,-1.,2.07892715110987));
#42391=CARTESIAN_POINT('Ctrl Pts',(0.12778444527612,1.,2.07892715110987));
#42392=CARTESIAN_POINT('Ctrl Pts',(0.130100748328403,-1.,2.07314114713063));
#42393=CARTESIAN_POINT('Ctrl Pts',(0.130100748328403,1.,2.07314114713063));
#42394=CARTESIAN_POINT('Ctrl Pts',(0.13237211154771,-1.,2.06735123910326));
#42395=CARTESIAN_POINT('Ctrl Pts',(0.13237211154771,1.,2.06735123910326));
#42396=CARTESIAN_POINT('Ctrl Pts',(0.134598026192106,-1.,2.06155781517842));
#42397=CARTESIAN_POINT('Ctrl Pts',(0.134598026192106,1.,2.06155781517842));
#42398=CARTESIAN_POINT('Ctrl Pts',(0.136777941218043,-1.,2.05576044414264));
#42399=CARTESIAN_POINT('Ctrl Pts',(0.136777941218043,1.,2.05576044414264));
#42400=CARTESIAN_POINT('Ctrl Pts',(0.138911255368966,-1.,2.04995762001328));
#42401=CARTESIAN_POINT('Ctrl Pts',(0.138911255368966,1.,2.04995762001328));
#42402=CARTESIAN_POINT('Ctrl Pts',(0.140997332152546,-1.,2.04414757947916));
#42403=CARTESIAN_POINT('Ctrl Pts',(0.140997332152546,1.,2.04414757947916));
#42404=CARTESIAN_POINT('Ctrl Pts',(0.143035515058208,-1.,2.03832911025912));
#42405=CARTESIAN_POINT('Ctrl Pts',(0.143035515058208,1.,2.03832911025912));
#42406=CARTESIAN_POINT('Ctrl Pts',(0.145025140186057,-1.,2.03250223739942));
#42407=CARTESIAN_POINT('Ctrl Pts',(0.145025140186057,1.,2.03250223739942));
#42408=CARTESIAN_POINT('Ctrl Pts',(0.146965557332583,-1.,2.02666926182017));
#42409=CARTESIAN_POINT('Ctrl Pts',(0.146965557332583,1.,2.02666926182017));
#42410=CARTESIAN_POINT('Ctrl Pts',(0.148856124775337,-1.,2.02083464969894));
#42411=CARTESIAN_POINT('Ctrl Pts',(0.148856124775337,1.,2.02083464969894));
#42412=CARTESIAN_POINT('Ctrl Pts',(0.150696157673078,-1.,2.01500291940238));
#42413=CARTESIAN_POINT('Ctrl Pts',(0.150696157673078,1.,2.01500291940238));
#42414=CARTESIAN_POINT('Ctrl Pts',(0.152484883621449,-1.,2.00917680318424));
#42415=CARTESIAN_POINT('Ctrl Pts',(0.152484883621449,1.,2.00917680318424));
#42416=CARTESIAN_POINT('Ctrl Pts',(0.154221403049722,-1.,2.00335565310543));
#42417=CARTESIAN_POINT('Ctrl Pts',(0.154221403049722,1.,2.00335565310543));
#42418=CARTESIAN_POINT('Ctrl Pts',(0.155904629548783,-1.,1.99753284771497));
#42419=CARTESIAN_POINT('Ctrl Pts',(0.155904629548783,1.,1.99753284771497));
#42420=CARTESIAN_POINT('Ctrl Pts',(0.157533331459227,-1.,1.99169810931908));
#42421=CARTESIAN_POINT('Ctrl Pts',(0.157533331459227,1.,1.99169810931908));
#42422=CARTESIAN_POINT('Ctrl Pts',(0.159106226437299,-1.,1.98584238283292));
#42423=CARTESIAN_POINT('Ctrl Pts',(0.159106226437299,1.,1.98584238283292));
#42424=CARTESIAN_POINT('Ctrl Pts',(0.160622060784611,-1.,1.97996195437559));
#42425=CARTESIAN_POINT('Ctrl Pts',(0.160622060784611,1.,1.97996195437559));
#42426=CARTESIAN_POINT('Ctrl Pts',(0.162079693556288,-1.,1.97406280235188));
#42427=CARTESIAN_POINT('Ctrl Pts',(0.162079693556288,1.,1.97406280235188));
#42428=CARTESIAN_POINT('Ctrl Pts',(0.163478185457734,-1.,1.96816512677967));
#42429=CARTESIAN_POINT('Ctrl Pts',(0.163478185457734,1.,1.96816512677967));
#42430=CARTESIAN_POINT('Ctrl Pts',(0.164816568920269,-1.,1.96229379940136));
#42431=CARTESIAN_POINT('Ctrl Pts',(0.164816568920269,1.,1.96229379940136));
#42432=CARTESIAN_POINT('Ctrl Pts',(0.166093592002812,-1.,1.9564675971873));
#42433=CARTESIAN_POINT('Ctrl Pts',(0.166093592002812,1.,1.9564675971873));
#42434=CARTESIAN_POINT('Ctrl Pts',(0.167307501784475,-1.,1.95069027794294));
#42435=CARTESIAN_POINT('Ctrl Pts',(0.167307501784475,1.,1.95069027794294));
#42436=CARTESIAN_POINT('Ctrl Pts',(0.168455741607556,-1.,1.94493757756931));
#42437=CARTESIAN_POINT('Ctrl Pts',(0.168455741607556,1.,1.94493757756931));
#42438=CARTESIAN_POINT('Ctrl Pts',(0.16953490481749,-1.,1.93915639211581));
#42439=CARTESIAN_POINT('Ctrl Pts',(0.16953490481749,1.,1.93915639211581));
#42440=CARTESIAN_POINT('Ctrl Pts',(0.170541253116201,-1.,1.93329183155539));
#42441=CARTESIAN_POINT('Ctrl Pts',(0.170541253116201,1.,1.93329183155539));
#42442=CARTESIAN_POINT('Ctrl Pts',(0.171471191532988,-1.,1.92731093582036));
#42443=CARTESIAN_POINT('Ctrl Pts',(0.171471191532988,1.,1.92731093582036));
#42444=CARTESIAN_POINT('Ctrl Pts',(0.172321621259513,-1.,1.9212233439798));
#42445=CARTESIAN_POINT('Ctrl Pts',(0.172321621259513,1.,1.9212233439798));
#42446=CARTESIAN_POINT('Ctrl Pts',(0.173090695383496,-1.,1.91511429159527));
#42447=CARTESIAN_POINT('Ctrl Pts',(0.173090695383496,1.,1.91511429159527));
#42448=CARTESIAN_POINT('Ctrl Pts',(0.173776635257816,-1.,1.90911693975267));
#42449=CARTESIAN_POINT('Ctrl Pts',(0.173776635257816,1.,1.90911693975267));
#42450=CARTESIAN_POINT('Ctrl Pts',(0.174375518661085,-1.,1.90335253862834));
#42451=CARTESIAN_POINT('Ctrl Pts',(0.174375518661085,1.,1.90335253862834));
#42452=CARTESIAN_POINT('Ctrl Pts',(0.174879405091263,-1.,1.89788101117132));
#42453=CARTESIAN_POINT('Ctrl Pts',(0.174879405091263,1.,1.89788101117132));
#42454=CARTESIAN_POINT('Ctrl Pts',(0.175274276190844,-1.,1.892646301985));
#42455=CARTESIAN_POINT('Ctrl Pts',(0.175274276190844,1.,1.892646301985));
#42456=CARTESIAN_POINT('Ctrl Pts',(0.175538155840648,-1.,1.88742606273259));
#42457=CARTESIAN_POINT('Ctrl Pts',(0.175538155840648,1.,1.88742606273259));
#42458=CARTESIAN_POINT('Ctrl Pts',(0.175644148889698,-1.,1.88188663145367));
#42459=CARTESIAN_POINT('Ctrl Pts',(0.175644148889698,1.,1.88188663145367));
#42460=CARTESIAN_POINT('Ctrl Pts',(0.175563480746485,-1.,1.87563767773588));
#42461=CARTESIAN_POINT('Ctrl Pts',(0.175563480746485,1.,1.87563767773588));
#42462=CARTESIAN_POINT('Ctrl Pts',(0.175268337590757,-1.,1.86828349694799));
#42463=CARTESIAN_POINT('Ctrl Pts',(0.175268337590757,1.,1.86828349694799));
#42464=CARTESIAN_POINT('Ctrl Pts',(0.17473525927603,-1.,1.85948367088837));
#42465=CARTESIAN_POINT('Ctrl Pts',(0.17473525927603,1.,1.85948367088837));
#42466=CARTESIAN_POINT('Ctrl Pts',(0.173946627587731,-1.,1.8489811319852));
#42467=CARTESIAN_POINT('Ctrl Pts',(0.173946627587731,1.,1.8489811319852));
#42468=CARTESIAN_POINT('Ctrl Pts',(0.1728894428919,-1.,1.83658380527692));
#42469=CARTESIAN_POINT('Ctrl Pts',(0.1728894428919,1.,1.83658380527692));
#42470=CARTESIAN_POINT('Ctrl Pts',(0.171554770204119,-1.,1.82215766811545));
#42471=CARTESIAN_POINT('Ctrl Pts',(0.171554770204119,1.,1.82215766811545));
#42472=CARTESIAN_POINT('Ctrl Pts',(0.169936923904608,-1.,1.80561530629706));
#42473=CARTESIAN_POINT('Ctrl Pts',(0.169936923904608,1.,1.80561530629706));
#42474=CARTESIAN_POINT('Ctrl Pts',(0.168032772805197,-1.,1.7869064998507));
#42475=CARTESIAN_POINT('Ctrl Pts',(0.168032772805197,1.,1.7869064998507));
#42476=CARTESIAN_POINT('Ctrl Pts',(0.1662793551464,-1.,1.77018771684844));
#42477=CARTESIAN_POINT('Ctrl Pts',(0.1662793551464,1.,1.77018771684844));
#42478=CARTESIAN_POINT('Ctrl Pts',(0.164834765707158,-1.,1.75666056638427));
#42479=CARTESIAN_POINT('Ctrl Pts',(0.164834765707158,1.,1.75666056638427));
#42480=CARTESIAN_POINT('Ctrl Pts',(0.163814161002002,-1.,1.7472034950333));
#42481=CARTESIAN_POINT('Ctrl Pts',(0.163814161002002,1.,1.7472034950333));
#42482=CARTESIAN_POINT('Ctrl Pts',(0.163289472382896,-1.,1.74236521665491));
#42483=CARTESIAN_POINT('Ctrl Pts',(0.163289472382896,1.,1.74236521665491));
#42484=CARTESIAN_POINT('',(0.0694764450219578,1.,2.19890268624765));
#42485=CARTESIAN_POINT('Ctrl Pts',(0.0694764450219578,1.,2.19890268624765));
#42486=CARTESIAN_POINT('Ctrl Pts',(0.0701143536325487,1.,2.19777582085423));
#42487=CARTESIAN_POINT('Ctrl Pts',(0.0713863779526151,1.,2.19552129484002));
#42488=CARTESIAN_POINT('Ctrl Pts',(0.0732830357306722,1.,2.19213712013662));
#42489=CARTESIAN_POINT('Ctrl Pts',(0.0757891465836145,1.,2.1876201139953));
#42490=CARTESIAN_POINT('Ctrl Pts',(0.078883772768524,1.,2.18196589448887));
#42491=CARTESIAN_POINT('Ctrl Pts',(0.0819402680872763,1.,2.176303712113));
#42492=CARTESIAN_POINT('Ctrl Pts',(0.084958462083537,1.,2.17063357870952));
#42493=CARTESIAN_POINT('Ctrl Pts',(0.087938129138692,1.,2.16495552645014));
#42494=CARTESIAN_POINT('Ctrl Pts',(0.0908789888107263,1.,2.15926961544516));
#42495=CARTESIAN_POINT('Ctrl Pts',(0.0937807218867641,1.,2.1535759397817));
#42496=CARTESIAN_POINT('Ctrl Pts',(0.0966429852305456,1.,2.14787463531795));
#42497=CARTESIAN_POINT('Ctrl Pts',(0.0994654261990913,1.,2.14216588396025));
#42498=CARTESIAN_POINT('Ctrl Pts',(0.1022477005561,1.,2.13644992667165));
#42499=CARTESIAN_POINT('Ctrl Pts',(0.104989479152739,1.,2.13072704887293));
#42500=CARTESIAN_POINT('Ctrl Pts',(0.10769043523109,1.,2.12499752307));
#42501=CARTESIAN_POINT('Ctrl Pts',(0.110350236135025,1.,2.11926155590865));
#42502=CARTESIAN_POINT('Ctrl Pts',(0.112968534419737,1.,2.11351924490306));
#42503=CARTESIAN_POINT('Ctrl Pts',(0.115544957687926,1.,2.10777050261309));
#42504=CARTESIAN_POINT('Ctrl Pts',(0.118079107988355,1.,2.102015121329));
#42505=CARTESIAN_POINT('Ctrl Pts',(0.120570567965122,1.,2.0962529286773));
#42506=CARTESIAN_POINT('Ctrl Pts',(0.123018905621083,1.,2.09048392424825));
#42507=CARTESIAN_POINT('Ctrl Pts',(0.125423679412061,1.,2.08470840653643));
#42508=CARTESIAN_POINT('Ctrl Pts',(0.12778444527612,1.,2.07892715110987));
#42509=CARTESIAN_POINT('Ctrl Pts',(0.130100748328403,1.,2.07314114713063));
#42510=CARTESIAN_POINT('Ctrl Pts',(0.13237211154771,1.,2.06735123910326));
#42511=CARTESIAN_POINT('Ctrl Pts',(0.134598026192106,1.,2.06155781517842));
#42512=CARTESIAN_POINT('Ctrl Pts',(0.136777941218043,1.,2.05576044414264));
#42513=CARTESIAN_POINT('Ctrl Pts',(0.138911255368966,1.,2.04995762001328));
#42514=CARTESIAN_POINT('Ctrl Pts',(0.140997332152546,1.,2.04414757947916));
#42515=CARTESIAN_POINT('Ctrl Pts',(0.143035515058208,1.,2.03832911025912));
#42516=CARTESIAN_POINT('Ctrl Pts',(0.145025140186057,1.,2.03250223739942));
#42517=CARTESIAN_POINT('Ctrl Pts',(0.146965557332583,1.,2.02666926182017));
#42518=CARTESIAN_POINT('Ctrl Pts',(0.148856124775337,1.,2.02083464969894));
#42519=CARTESIAN_POINT('Ctrl Pts',(0.150696157673078,1.,2.01500291940238));
#42520=CARTESIAN_POINT('Ctrl Pts',(0.152484883621449,1.,2.00917680318424));
#42521=CARTESIAN_POINT('Ctrl Pts',(0.154221403049722,1.,2.00335565310543));
#42522=CARTESIAN_POINT('Ctrl Pts',(0.155904629548783,1.,1.99753284771497));
#42523=CARTESIAN_POINT('Ctrl Pts',(0.157533331459227,1.,1.99169810931908));
#42524=CARTESIAN_POINT('Ctrl Pts',(0.159106226437299,1.,1.98584238283292));
#42525=CARTESIAN_POINT('Ctrl Pts',(0.160622060784611,1.,1.97996195437559));
#42526=CARTESIAN_POINT('Ctrl Pts',(0.162079693556288,1.,1.97406280235188));
#42527=CARTESIAN_POINT('Ctrl Pts',(0.163478185457734,1.,1.96816512677967));
#42528=CARTESIAN_POINT('Ctrl Pts',(0.164816568920269,1.,1.96229379940136));
#42529=CARTESIAN_POINT('Ctrl Pts',(0.166093592002812,1.,1.9564675971873));
#42530=CARTESIAN_POINT('Ctrl Pts',(0.167307501784475,1.,1.95069027794294));
#42531=CARTESIAN_POINT('Ctrl Pts',(0.168455741607556,1.,1.94493757756931));
#42532=CARTESIAN_POINT('Ctrl Pts',(0.16953490481749,1.,1.93915639211581));
#42533=CARTESIAN_POINT('Ctrl Pts',(0.170541253116201,1.,1.93329183155539));
#42534=CARTESIAN_POINT('Ctrl Pts',(0.171471191532988,1.,1.92731093582036));
#42535=CARTESIAN_POINT('Ctrl Pts',(0.172321621259513,1.,1.9212233439798));
#42536=CARTESIAN_POINT('Ctrl Pts',(0.173090695383496,1.,1.91511429159527));
#42537=CARTESIAN_POINT('Ctrl Pts',(0.173776635257816,1.,1.90911693975267));
#42538=CARTESIAN_POINT('Ctrl Pts',(0.174375518661085,1.,1.90335253862834));
#42539=CARTESIAN_POINT('Ctrl Pts',(0.174879405091263,1.,1.89788101117132));
#42540=CARTESIAN_POINT('Ctrl Pts',(0.175274276190844,1.,1.892646301985));
#42541=CARTESIAN_POINT('Ctrl Pts',(0.175538155840648,1.,1.88742606273259));
#42542=CARTESIAN_POINT('Ctrl Pts',(0.175644148889698,1.,1.88188663145367));
#42543=CARTESIAN_POINT('Ctrl Pts',(0.175563480746485,1.,1.87563767773588));
#42544=CARTESIAN_POINT('Ctrl Pts',(0.175268337590757,1.,1.86828349694799));
#42545=CARTESIAN_POINT('Ctrl Pts',(0.17473525927603,1.,1.85948367088837));
#42546=CARTESIAN_POINT('Ctrl Pts',(0.173946627587731,1.,1.8489811319852));
#42547=CARTESIAN_POINT('Ctrl Pts',(0.1728894428919,1.,1.83658380527692));
#42548=CARTESIAN_POINT('Ctrl Pts',(0.171554770204119,1.,1.82215766811545));
#42549=CARTESIAN_POINT('Ctrl Pts',(0.169936923904608,1.,1.80561530629706));
#42550=CARTESIAN_POINT('Ctrl Pts',(0.168032772805197,1.,1.7869064998507));
#42551=CARTESIAN_POINT('Ctrl Pts',(0.1662793551464,1.,1.77018771684844));
#42552=CARTESIAN_POINT('Ctrl Pts',(0.164834765707158,1.,1.75666056638427));
#42553=CARTESIAN_POINT('Ctrl Pts',(0.163814161002002,1.,1.7472034950333));
#42554=CARTESIAN_POINT('Ctrl Pts',(0.163289472382896,1.,1.74236521665491));
#42555=CARTESIAN_POINT('',(0.0694764450219578,0.,2.19890268624765));
#42556=CARTESIAN_POINT('Origin',(-0.0694764450219586,0.,2.19890268624765));
#42557=CARTESIAN_POINT('',(-0.0694764450219586,1.,2.19890268624765));
#42558=CARTESIAN_POINT('',(0.0694764450219578,1.,2.19890268624765));
#42559=CARTESIAN_POINT('',(-0.0694764450219586,0.,2.19890268624765));
#42560=CARTESIAN_POINT('Ctrl Pts',(-0.163289472382896,-1.,1.74236521665491));
#42561=CARTESIAN_POINT('Ctrl Pts',(-0.163289472382896,1.,1.74236521665491));
#42562=CARTESIAN_POINT('Ctrl Pts',(-0.163814161002474,-1.,1.74720349503904));
#42563=CARTESIAN_POINT('Ctrl Pts',(-0.163814161002474,1.,1.74720349503904));
#42564=CARTESIAN_POINT('Ctrl Pts',(-0.164834765708484,-1.,1.75666056640041));
#42565=CARTESIAN_POINT('Ctrl Pts',(-0.164834765708484,1.,1.75666056640041));
#42566=CARTESIAN_POINT('Ctrl Pts',(-0.166279355148738,-1.,1.77018771687692));
#42567=CARTESIAN_POINT('Ctrl Pts',(-0.166279355148738,1.,1.77018771687692));
#42568=CARTESIAN_POINT('Ctrl Pts',(-0.16803277280837,-1.,1.78690649988931));
#42569=CARTESIAN_POINT('Ctrl Pts',(-0.16803277280837,1.,1.78690649988931));
#42570=CARTESIAN_POINT('Ctrl Pts',(-0.169936923908078,-1.,1.80561530633924));
#42571=CARTESIAN_POINT('Ctrl Pts',(-0.169936923908078,1.,1.80561530633924));
#42572=CARTESIAN_POINT('Ctrl Pts',(-0.171554770207306,-1.,1.82215766815414));
#42573=CARTESIAN_POINT('Ctrl Pts',(-0.171554770207306,1.,1.82215766815414));
#42574=CARTESIAN_POINT('Ctrl Pts',(-0.17288944289442,-1.,1.83658380530747));
#42575=CARTESIAN_POINT('Ctrl Pts',(-0.17288944289442,1.,1.83658380530747));
#42576=CARTESIAN_POINT('Ctrl Pts',(-0.173946627589401,-1.,1.84898113200543));
#42577=CARTESIAN_POINT('Ctrl Pts',(-0.173946627589401,1.,1.84898113200543));
#42578=CARTESIAN_POINT('Ctrl Pts',(-0.174735259276856,-1.,1.85948367089838));
#42579=CARTESIAN_POINT('Ctrl Pts',(-0.174735259276856,1.,1.85948367089838));
#42580=CARTESIAN_POINT('Ctrl Pts',(-0.175268337590901,-1.,1.86828349694972));
#42581=CARTESIAN_POINT('Ctrl Pts',(-0.175268337590901,1.,1.86828349694972));
#42582=CARTESIAN_POINT('Ctrl Pts',(-0.175563480746206,-1.,1.87563767773249));
#42583=CARTESIAN_POINT('Ctrl Pts',(-0.175563480746206,1.,1.87563767773249));
#42584=CARTESIAN_POINT('Ctrl Pts',(-0.175644148889271,-1.,1.88188663144846));
#42585=CARTESIAN_POINT('Ctrl Pts',(-0.175644148889271,1.,1.88188663144846));
#42586=CARTESIAN_POINT('Ctrl Pts',(-0.175538155840286,-1.,1.88742606272818));
#42587=CARTESIAN_POINT('Ctrl Pts',(-0.175538155840286,1.,1.88742606272818));
#42588=CARTESIAN_POINT('Ctrl Pts',(-0.175274276190664,-1.,1.89264630198279));
#42589=CARTESIAN_POINT('Ctrl Pts',(-0.175274276190664,1.,1.89264630198279));
#42590=CARTESIAN_POINT('Ctrl Pts',(-0.174879405091277,-1.,1.89788101117148));
#42591=CARTESIAN_POINT('Ctrl Pts',(-0.174879405091277,1.,1.89788101117148));
#42592=CARTESIAN_POINT('Ctrl Pts',(-0.174375518661222,-1.,1.90335253863003));
#42593=CARTESIAN_POINT('Ctrl Pts',(-0.174375518661222,1.,1.90335253863003));
#42594=CARTESIAN_POINT('Ctrl Pts',(-0.173776635257984,-1.,1.90911693975475));
#42595=CARTESIAN_POINT('Ctrl Pts',(-0.173776635257984,1.,1.90911693975475));
#42596=CARTESIAN_POINT('Ctrl Pts',(-0.173090695383619,-1.,1.91511429159681));
#42597=CARTESIAN_POINT('Ctrl Pts',(-0.173090695383619,1.,1.91511429159681));
#42598=CARTESIAN_POINT('Ctrl Pts',(-0.172321621259557,-1.,1.92122334398034));
#42599=CARTESIAN_POINT('Ctrl Pts',(-0.172321621259557,1.,1.92122334398034));
#42600=CARTESIAN_POINT('Ctrl Pts',(-0.17147119153296,-1.,1.92731093582));
#42601=CARTESIAN_POINT('Ctrl Pts',(-0.17147119153296,1.,1.92731093582));
#42602=CARTESIAN_POINT('Ctrl Pts',(-0.170541253116136,-1.,1.93329183155455));
#42603=CARTESIAN_POINT('Ctrl Pts',(-0.170541253116136,1.,1.93329183155455));
#42604=CARTESIAN_POINT('Ctrl Pts',(-0.169534904817425,-1.,1.93915639211497));
#42605=CARTESIAN_POINT('Ctrl Pts',(-0.169534904817425,1.,1.93915639211497));
#42606=CARTESIAN_POINT('Ctrl Pts',(-0.168455741607516,-1.,1.94493757756879));
#42607=CARTESIAN_POINT('Ctrl Pts',(-0.168455741607516,1.,1.94493757756879));
#42608=CARTESIAN_POINT('Ctrl Pts',(-0.167307501784469,-1.,1.95069027794286));
#42609=CARTESIAN_POINT('Ctrl Pts',(-0.167307501784469,1.,1.95069027794286));
#42610=CARTESIAN_POINT('Ctrl Pts',(-0.166093592002833,-1.,1.95646759718755));
#42611=CARTESIAN_POINT('Ctrl Pts',(-0.166093592002833,1.,1.95646759718755));
#42612=CARTESIAN_POINT('Ctrl Pts',(-0.1648165689203,-1.,1.96229379940174));
#42613=CARTESIAN_POINT('Ctrl Pts',(-0.1648165689203,1.,1.96229379940174));
#42614=CARTESIAN_POINT('Ctrl Pts',(-0.16347818545776,-1.,1.96816512678));
#42615=CARTESIAN_POINT('Ctrl Pts',(-0.16347818545776,1.,1.96816512678));
#42616=CARTESIAN_POINT('Ctrl Pts',(-0.162079693556302,-1.,1.97406280235204));
#42617=CARTESIAN_POINT('Ctrl Pts',(-0.162079693556302,1.,1.97406280235204));
#42618=CARTESIAN_POINT('Ctrl Pts',(-0.16062206078461,-1.,1.97996195437557));
#42619=CARTESIAN_POINT('Ctrl Pts',(-0.16062206078461,1.,1.97996195437557));
#42620=CARTESIAN_POINT('Ctrl Pts',(-0.159106226437289,-1.,1.98584238283279));
#42621=CARTESIAN_POINT('Ctrl Pts',(-0.159106226437289,1.,1.98584238283279));
#42622=CARTESIAN_POINT('Ctrl Pts',(-0.157533331459215,-1.,1.99169810931893));
#42623=CARTESIAN_POINT('Ctrl Pts',(-0.157533331459215,1.,1.99169810931893));
#42624=CARTESIAN_POINT('Ctrl Pts',(-0.155904629548775,-1.,1.99753284771487));
#42625=CARTESIAN_POINT('Ctrl Pts',(-0.155904629548775,1.,1.99753284771487));
#42626=CARTESIAN_POINT('Ctrl Pts',(-0.154221403049719,-1.,2.00335565310539));
#42627=CARTESIAN_POINT('Ctrl Pts',(-0.154221403049719,1.,2.00335565310539));
#42628=CARTESIAN_POINT('Ctrl Pts',(-0.152484883621452,-1.,2.00917680318426));
#42629=CARTESIAN_POINT('Ctrl Pts',(-0.152484883621452,1.,2.00917680318426));
#42630=CARTESIAN_POINT('Ctrl Pts',(-0.150696157673084,-1.,2.01500291940243));
#42631=CARTESIAN_POINT('Ctrl Pts',(-0.150696157673084,1.,2.01500291940243));
#42632=CARTESIAN_POINT('Ctrl Pts',(-0.148856124775343,-1.,2.02083464969897));
#42633=CARTESIAN_POINT('Ctrl Pts',(-0.148856124775343,1.,2.02083464969897));
#42634=CARTESIAN_POINT('Ctrl Pts',(-0.146965557332586,-1.,2.02666926182017));
#42635=CARTESIAN_POINT('Ctrl Pts',(-0.146965557332586,1.,2.02666926182017));
#42636=CARTESIAN_POINT('Ctrl Pts',(-0.145025140186058,-1.,2.03250223739941));
#42637=CARTESIAN_POINT('Ctrl Pts',(-0.145025140186058,1.,2.03250223739941));
#42638=CARTESIAN_POINT('Ctrl Pts',(-0.143035515058208,-1.,2.03832911025913));
#42639=CARTESIAN_POINT('Ctrl Pts',(-0.143035515058208,1.,2.03832911025913));
#42640=CARTESIAN_POINT('Ctrl Pts',(-0.140997332152546,-1.,2.04414757947919));
#42641=CARTESIAN_POINT('Ctrl Pts',(-0.140997332152546,1.,2.04414757947919));
#42642=CARTESIAN_POINT('Ctrl Pts',(-0.138911255368966,-1.,2.04995762001333));
#42643=CARTESIAN_POINT('Ctrl Pts',(-0.138911255368966,1.,2.04995762001333));
#42644=CARTESIAN_POINT('Ctrl Pts',(-0.136777941218044,-1.,2.0557604441427));
#42645=CARTESIAN_POINT('Ctrl Pts',(-0.136777941218044,1.,2.0557604441427));
#42646=CARTESIAN_POINT('Ctrl Pts',(-0.134598026192107,-1.,2.06155781517844));
#42647=CARTESIAN_POINT('Ctrl Pts',(-0.134598026192107,1.,2.06155781517844));
#42648=CARTESIAN_POINT('Ctrl Pts',(-0.13237211154771,-1.,2.06735123910319));
#42649=CARTESIAN_POINT('Ctrl Pts',(-0.13237211154771,1.,2.06735123910319));
#42650=CARTESIAN_POINT('Ctrl Pts',(-0.130100748328401,-1.,2.07314114713047));
#42651=CARTESIAN_POINT('Ctrl Pts',(-0.130100748328401,1.,2.07314114713047));
#42652=CARTESIAN_POINT('Ctrl Pts',(-0.127784445276116,-1.,2.07892715110967));
#42653=CARTESIAN_POINT('Ctrl Pts',(-0.127784445276116,1.,2.07892715110967));
#42654=CARTESIAN_POINT('Ctrl Pts',(-0.125423679412058,-1.,2.08470840653628));
#42655=CARTESIAN_POINT('Ctrl Pts',(-0.125423679412058,1.,2.08470840653628));
#42656=CARTESIAN_POINT('Ctrl Pts',(-0.123018905621083,-1.,2.09048392424826));
#42657=CARTESIAN_POINT('Ctrl Pts',(-0.123018905621083,1.,2.09048392424826));
#42658=CARTESIAN_POINT('Ctrl Pts',(-0.120570567965129,-1.,2.09625292867756));
#42659=CARTESIAN_POINT('Ctrl Pts',(-0.120570567965129,1.,2.09625292867756));
#42660=CARTESIAN_POINT('Ctrl Pts',(-0.118079107988368,-1.,2.10201512132945));
#42661=CARTESIAN_POINT('Ctrl Pts',(-0.118079107988368,1.,2.10201512132945));
#42662=CARTESIAN_POINT('Ctrl Pts',(-0.115544957687941,-1.,2.10777050261359));
#42663=CARTESIAN_POINT('Ctrl Pts',(-0.115544957687941,1.,2.10777050261359));
#42664=CARTESIAN_POINT('Ctrl Pts',(-0.112968534419746,-1.,2.11351924490335));
#42665=CARTESIAN_POINT('Ctrl Pts',(-0.112968534419746,1.,2.11351924490335));
#42666=CARTESIAN_POINT('Ctrl Pts',(-0.11035023613502,-1.,2.11926155590849));
#42667=CARTESIAN_POINT('Ctrl Pts',(-0.11035023613502,1.,2.11926155590849));
#42668=CARTESIAN_POINT('Ctrl Pts',(-0.107690435231068,-1.,2.12499752306927));
#42669=CARTESIAN_POINT('Ctrl Pts',(-0.107690435231068,1.,2.12499752306927));
#42670=CARTESIAN_POINT('Ctrl Pts',(-0.104989479152703,-1.,2.1307270488718));
#42671=CARTESIAN_POINT('Ctrl Pts',(-0.104989479152703,1.,2.1307270488718));
#42672=CARTESIAN_POINT('Ctrl Pts',(-0.102247700556064,-1.,2.13644992667052));
#42673=CARTESIAN_POINT('Ctrl Pts',(-0.102247700556064,1.,2.13644992667052));
#42674=CARTESIAN_POINT('Ctrl Pts',(-0.0994654261990745,-1.,2.14216588395974));
#42675=CARTESIAN_POINT('Ctrl Pts',(-0.0994654261990745,1.,2.14216588395974));
#42676=CARTESIAN_POINT('Ctrl Pts',(-0.0966429852305691,-1.,2.14787463531864));
#42677=CARTESIAN_POINT('Ctrl Pts',(-0.0966429852305691,1.,2.14787463531864));
#42678=CARTESIAN_POINT('Ctrl Pts',(-0.0937807218868348,-1.,2.15357593978377));
#42679=CARTESIAN_POINT('Ctrl Pts',(-0.0937807218868348,1.,2.15357593978377));
#42680=CARTESIAN_POINT('Ctrl Pts',(-0.0908789888108269,-1.,2.15926961544808));
#42681=CARTESIAN_POINT('Ctrl Pts',(-0.0908789888108269,1.,2.15926961544808));
#42682=CARTESIAN_POINT('Ctrl Pts',(-0.0879381291387825,-1.,2.16495552645275));
#42683=CARTESIAN_POINT('Ctrl Pts',(-0.0879381291387825,1.,2.16495552645275));
#42684=CARTESIAN_POINT('Ctrl Pts',(-0.0849584620835646,-1.,2.17063357871031));
#42685=CARTESIAN_POINT('Ctrl Pts',(-0.0849584620835646,1.,2.17063357871031));
#42686=CARTESIAN_POINT('Ctrl Pts',(-0.0819402680871942,-1.,2.1763037121106));
#42687=CARTESIAN_POINT('Ctrl Pts',(-0.0819402680871942,1.,2.1763037121106));
#42688=CARTESIAN_POINT('Ctrl Pts',(-0.078883772768323,-1.,2.18196589448304));
#42689=CARTESIAN_POINT('Ctrl Pts',(-0.078883772768323,1.,2.18196589448304));
#42690=CARTESIAN_POINT('Ctrl Pts',(-0.0757891465833414,-1.,2.1876201139874));
#42691=CARTESIAN_POINT('Ctrl Pts',(-0.0757891465833414,1.,2.1876201139874));
#42692=CARTESIAN_POINT('Ctrl Pts',(-0.0732830357304279,-1.,2.19213712012956));
#42693=CARTESIAN_POINT('Ctrl Pts',(-0.0732830357304279,1.,2.19213712012956));
#42694=CARTESIAN_POINT('Ctrl Pts',(-0.071386377952463,-1.,2.19552129483562));
#42695=CARTESIAN_POINT('Ctrl Pts',(-0.071386377952463,1.,2.19552129483562));
#42696=CARTESIAN_POINT('Ctrl Pts',(-0.0701143536324929,-1.,2.19777582085261));
#42697=CARTESIAN_POINT('Ctrl Pts',(-0.0701143536324929,1.,2.19777582085261));
#42698=CARTESIAN_POINT('Ctrl Pts',(-0.0694764450219586,-1.,2.19890268624765));
#42699=CARTESIAN_POINT('Ctrl Pts',(-0.0694764450219586,1.,2.19890268624765));
#42700=CARTESIAN_POINT('',(-0.163289472382896,1.,1.74236521665491));
#42701=CARTESIAN_POINT('Ctrl Pts',(-0.163289472382896,1.,1.74236521665491));
#42702=CARTESIAN_POINT('Ctrl Pts',(-0.163814161002474,1.,1.74720349503904));
#42703=CARTESIAN_POINT('Ctrl Pts',(-0.164834765708484,1.,1.75666056640041));
#42704=CARTESIAN_POINT('Ctrl Pts',(-0.166279355148738,1.,1.77018771687692));
#42705=CARTESIAN_POINT('Ctrl Pts',(-0.16803277280837,1.,1.78690649988931));
#42706=CARTESIAN_POINT('Ctrl Pts',(-0.169936923908078,1.,1.80561530633924));
#42707=CARTESIAN_POINT('Ctrl Pts',(-0.171554770207306,1.,1.82215766815414));
#42708=CARTESIAN_POINT('Ctrl Pts',(-0.17288944289442,1.,1.83658380530747));
#42709=CARTESIAN_POINT('Ctrl Pts',(-0.173946627589401,1.,1.84898113200543));
#42710=CARTESIAN_POINT('Ctrl Pts',(-0.174735259276856,1.,1.85948367089838));
#42711=CARTESIAN_POINT('Ctrl Pts',(-0.175268337590901,1.,1.86828349694972));
#42712=CARTESIAN_POINT('Ctrl Pts',(-0.175563480746206,1.,1.87563767773249));
#42713=CARTESIAN_POINT('Ctrl Pts',(-0.175644148889271,1.,1.88188663144846));
#42714=CARTESIAN_POINT('Ctrl Pts',(-0.175538155840286,1.,1.88742606272818));
#42715=CARTESIAN_POINT('Ctrl Pts',(-0.175274276190664,1.,1.89264630198279));
#42716=CARTESIAN_POINT('Ctrl Pts',(-0.174879405091277,1.,1.89788101117148));
#42717=CARTESIAN_POINT('Ctrl Pts',(-0.174375518661222,1.,1.90335253863003));
#42718=CARTESIAN_POINT('Ctrl Pts',(-0.173776635257984,1.,1.90911693975475));
#42719=CARTESIAN_POINT('Ctrl Pts',(-0.173090695383619,1.,1.91511429159681));
#42720=CARTESIAN_POINT('Ctrl Pts',(-0.172321621259557,1.,1.92122334398034));
#42721=CARTESIAN_POINT('Ctrl Pts',(-0.17147119153296,1.,1.92731093582));
#42722=CARTESIAN_POINT('Ctrl Pts',(-0.170541253116136,1.,1.93329183155455));
#42723=CARTESIAN_POINT('Ctrl Pts',(-0.169534904817425,1.,1.93915639211497));
#42724=CARTESIAN_POINT('Ctrl Pts',(-0.168455741607516,1.,1.94493757756879));
#42725=CARTESIAN_POINT('Ctrl Pts',(-0.167307501784469,1.,1.95069027794286));
#42726=CARTESIAN_POINT('Ctrl Pts',(-0.166093592002833,1.,1.95646759718755));
#42727=CARTESIAN_POINT('Ctrl Pts',(-0.1648165689203,1.,1.96229379940174));
#42728=CARTESIAN_POINT('Ctrl Pts',(-0.16347818545776,1.,1.96816512678));
#42729=CARTESIAN_POINT('Ctrl Pts',(-0.162079693556302,1.,1.97406280235204));
#42730=CARTESIAN_POINT('Ctrl Pts',(-0.16062206078461,1.,1.97996195437557));
#42731=CARTESIAN_POINT('Ctrl Pts',(-0.159106226437289,1.,1.98584238283279));
#42732=CARTESIAN_POINT('Ctrl Pts',(-0.157533331459215,1.,1.99169810931893));
#42733=CARTESIAN_POINT('Ctrl Pts',(-0.155904629548775,1.,1.99753284771487));
#42734=CARTESIAN_POINT('Ctrl Pts',(-0.154221403049719,1.,2.00335565310539));
#42735=CARTESIAN_POINT('Ctrl Pts',(-0.152484883621452,1.,2.00917680318426));
#42736=CARTESIAN_POINT('Ctrl Pts',(-0.150696157673084,1.,2.01500291940243));
#42737=CARTESIAN_POINT('Ctrl Pts',(-0.148856124775343,1.,2.02083464969897));
#42738=CARTESIAN_POINT('Ctrl Pts',(-0.146965557332586,1.,2.02666926182017));
#42739=CARTESIAN_POINT('Ctrl Pts',(-0.145025140186058,1.,2.03250223739941));
#42740=CARTESIAN_POINT('Ctrl Pts',(-0.143035515058208,1.,2.03832911025913));
#42741=CARTESIAN_POINT('Ctrl Pts',(-0.140997332152546,1.,2.04414757947919));
#42742=CARTESIAN_POINT('Ctrl Pts',(-0.138911255368966,1.,2.04995762001333));
#42743=CARTESIAN_POINT('Ctrl Pts',(-0.136777941218044,1.,2.0557604441427));
#42744=CARTESIAN_POINT('Ctrl Pts',(-0.134598026192107,1.,2.06155781517844));
#42745=CARTESIAN_POINT('Ctrl Pts',(-0.13237211154771,1.,2.06735123910319));
#42746=CARTESIAN_POINT('Ctrl Pts',(-0.130100748328401,1.,2.07314114713047));
#42747=CARTESIAN_POINT('Ctrl Pts',(-0.127784445276116,1.,2.07892715110967));
#42748=CARTESIAN_POINT('Ctrl Pts',(-0.125423679412058,1.,2.08470840653628));
#42749=CARTESIAN_POINT('Ctrl Pts',(-0.123018905621083,1.,2.09048392424826));
#42750=CARTESIAN_POINT('Ctrl Pts',(-0.120570567965129,1.,2.09625292867756));
#42751=CARTESIAN_POINT('Ctrl Pts',(-0.118079107988368,1.,2.10201512132945));
#42752=CARTESIAN_POINT('Ctrl Pts',(-0.115544957687941,1.,2.10777050261359));
#42753=CARTESIAN_POINT('Ctrl Pts',(-0.112968534419746,1.,2.11351924490335));
#42754=CARTESIAN_POINT('Ctrl Pts',(-0.11035023613502,1.,2.11926155590849));
#42755=CARTESIAN_POINT('Ctrl Pts',(-0.107690435231068,1.,2.12499752306927));
#42756=CARTESIAN_POINT('Ctrl Pts',(-0.104989479152703,1.,2.1307270488718));
#42757=CARTESIAN_POINT('Ctrl Pts',(-0.102247700556064,1.,2.13644992667052));
#42758=CARTESIAN_POINT('Ctrl Pts',(-0.0994654261990745,1.,2.14216588395974));
#42759=CARTESIAN_POINT('Ctrl Pts',(-0.0966429852305691,1.,2.14787463531864));
#42760=CARTESIAN_POINT('Ctrl Pts',(-0.0937807218868348,1.,2.15357593978377));
#42761=CARTESIAN_POINT('Ctrl Pts',(-0.0908789888108269,1.,2.15926961544808));
#42762=CARTESIAN_POINT('Ctrl Pts',(-0.0879381291387825,1.,2.16495552645275));
#42763=CARTESIAN_POINT('Ctrl Pts',(-0.0849584620835646,1.,2.17063357871031));
#42764=CARTESIAN_POINT('Ctrl Pts',(-0.0819402680871942,1.,2.1763037121106));
#42765=CARTESIAN_POINT('Ctrl Pts',(-0.078883772768323,1.,2.18196589448304));
#42766=CARTESIAN_POINT('Ctrl Pts',(-0.0757891465833414,1.,2.1876201139874));
#42767=CARTESIAN_POINT('Ctrl Pts',(-0.0732830357304279,1.,2.19213712012956));
#42768=CARTESIAN_POINT('Ctrl Pts',(-0.071386377952463,1.,2.19552129483562));
#42769=CARTESIAN_POINT('Ctrl Pts',(-0.0701143536324929,1.,2.19777582085261));
#42770=CARTESIAN_POINT('Ctrl Pts',(-0.0694764450219586,1.,2.19890268624765));
#42771=CARTESIAN_POINT('',(-0.163289472382897,0.,1.74236521665491));
#42772=CARTESIAN_POINT('Origin',(0.,0.,0.));
#42773=CARTESIAN_POINT('',(-0.383122945602004,1.,1.7075470150345));
#42774=CARTESIAN_POINT('Origin',(0.,1.,0.));
#42775=CARTESIAN_POINT('',(-0.383122945602004,0.,1.7075470150345));
#42776=CARTESIAN_POINT('Ctrl Pts',(-0.61342227326009,-1.,2.11275013067528));
#42777=CARTESIAN_POINT('Ctrl Pts',(-0.61342227326009,1.,2.11275013067528));
#42778=CARTESIAN_POINT('Ctrl Pts',(-0.61246736556225,-1.,2.11187554260142));
#42779=CARTESIAN_POINT('Ctrl Pts',(-0.61246736556225,1.,2.11187554260142));
#42780=CARTESIAN_POINT('Ctrl Pts',(-0.610560911691113,-1.,2.11012443807661));
#42781=CARTESIAN_POINT('Ctrl Pts',(-0.610560911691113,1.,2.11012443807661));
#42782=CARTESIAN_POINT('Ctrl Pts',(-0.607711315456826,-1.,2.10749199615859));
#42783=CARTESIAN_POINT('Ctrl Pts',(-0.607711315456826,1.,2.10749199615859));
#42784=CARTESIAN_POINT('Ctrl Pts',(-0.603932030738212,-1.,2.10397049887709));
#42785=CARTESIAN_POINT('Ctrl Pts',(-0.603932030738212,1.,2.10397049887709));
#42786=CARTESIAN_POINT('Ctrl Pts',(-0.599241616422144,-1.,2.09954930865331));
#42787=CARTESIAN_POINT('Ctrl Pts',(-0.599241616422144,1.,2.09954930865331));
#42788=CARTESIAN_POINT('Ctrl Pts',(-0.594585006052824,-1.,2.09510876220501));
#42789=CARTESIAN_POINT('Ctrl Pts',(-0.594585006052824,1.,2.09510876220501));
#42790=CARTESIAN_POINT('Ctrl Pts',(-0.589962365403189,-1.,2.09064881812053));
#42791=CARTESIAN_POINT('Ctrl Pts',(-0.589962365403189,1.,2.09064881812053));
#42792=CARTESIAN_POINT('Ctrl Pts',(-0.585373918990895,-1.,2.086169437277));
#42793=CARTESIAN_POINT('Ctrl Pts',(-0.585373918990895,1.,2.086169437277));
#42794=CARTESIAN_POINT('Ctrl Pts',(-0.580819952107257,-1.,2.08167059018138));
#42795=CARTESIAN_POINT('Ctrl Pts',(-0.580819952107257,1.,2.08167059018138));
#42796=CARTESIAN_POINT('Ctrl Pts',(-0.576300797416275,-1.,2.07715226767361));
#42797=CARTESIAN_POINT('Ctrl Pts',(-0.576300797416275,1.,2.07715226767361));
#42798=CARTESIAN_POINT('Ctrl Pts',(-0.571816823242411,-1.,2.07261449292757));
#42799=CARTESIAN_POINT('Ctrl Pts',(-0.571816823242411,1.,2.07261449292757));
#42800=CARTESIAN_POINT('Ctrl Pts',(-0.567368421181229,-1.,2.06805732997383));
#42801=CARTESIAN_POINT('Ctrl Pts',(-0.567368421181229,1.,2.06805732997383));
#42802=CARTESIAN_POINT('Ctrl Pts',(-0.562955993082574,-1.,2.06348090160697));
#42803=CARTESIAN_POINT('Ctrl Pts',(-0.562955993082574,1.,2.06348090160697));
#42804=CARTESIAN_POINT('Ctrl Pts',(-0.558579940185467,-1.,2.05888537756571));
#42805=CARTESIAN_POINT('Ctrl Pts',(-0.558579940185467,1.,2.05888537756571));
#42806=CARTESIAN_POINT('Ctrl Pts',(-0.55424065746411,-1.,2.05427091604482));
#42807=CARTESIAN_POINT('Ctrl Pts',(-0.55424065746411,1.,2.05427091604482));
#42808=CARTESIAN_POINT('Ctrl Pts',(-0.549938525150342,-1.,2.04963761077974));
#42809=CARTESIAN_POINT('Ctrl Pts',(-0.549938525150342,1.,2.04963761077974));
#42810=CARTESIAN_POINT('Ctrl Pts',(-0.545673903817348,-1.,2.0449854471456));
#42811=CARTESIAN_POINT('Ctrl Pts',(-0.545673903817348,1.,2.0449854471456));
#42812=CARTESIAN_POINT('Ctrl Pts',(-0.54144712061552,-1.,2.0403142269048));
#42813=CARTESIAN_POINT('Ctrl Pts',(-0.54144712061552,1.,2.0403142269048));
#42814=CARTESIAN_POINT('Ctrl Pts',(-0.537258489833134,-1.,2.03562362953993));
#42815=CARTESIAN_POINT('Ctrl Pts',(-0.537258489833134,1.,2.03562362953993));
#42816=CARTESIAN_POINT('Ctrl Pts',(-0.533108355132905,-1.,2.03091336214401));
#42817=CARTESIAN_POINT('Ctrl Pts',(-0.533108355132905,1.,2.03091336214401));
#42818=CARTESIAN_POINT('Ctrl Pts',(-0.528997127241911,-1.,2.02618329083289));
#42819=CARTESIAN_POINT('Ctrl Pts',(-0.528997127241911,1.,2.02618329083289));
#42820=CARTESIAN_POINT('Ctrl Pts',(-0.524925318333518,-1.,2.02143356304712));
#42821=CARTESIAN_POINT('Ctrl Pts',(-0.524925318333518,1.,2.02143356304712));
#42822=CARTESIAN_POINT('Ctrl Pts',(-0.520893590399428,-1.,2.01666477917305));
#42823=CARTESIAN_POINT('Ctrl Pts',(-0.520893590399428,1.,2.01666477917305));
#42824=CARTESIAN_POINT('Ctrl Pts',(-0.516902681728733,-1.,2.01187773939257));
#42825=CARTESIAN_POINT('Ctrl Pts',(-0.516902681728733,1.,2.01187773939257));
#42826=CARTESIAN_POINT('Ctrl Pts',(-0.512953306961814,-1.,2.00707309946955));
#42827=CARTESIAN_POINT('Ctrl Pts',(-0.512953306961814,1.,2.00707309946955));
#42828=CARTESIAN_POINT('Ctrl Pts',(-0.509046069886152,-1.,2.00225107134733));
#42829=CARTESIAN_POINT('Ctrl Pts',(-0.509046069886152,1.,2.00225107134733));
#42830=CARTESIAN_POINT('Ctrl Pts',(-0.505181361323011,-1.,1.99741107463567));
#42831=CARTESIAN_POINT('Ctrl Pts',(-0.505181361323011,1.,1.99741107463567));
#42832=CARTESIAN_POINT('Ctrl Pts',(-0.501359287727129,-1.,1.9925514912615));
#42833=CARTESIAN_POINT('Ctrl Pts',(-0.501359287727129,1.,1.9925514912615));
#42834=CARTESIAN_POINT('Ctrl Pts',(-0.497579909545564,-1.,1.98767044752929));
#42835=CARTESIAN_POINT('Ctrl Pts',(-0.497579909545564,1.,1.98767044752929));
#42836=CARTESIAN_POINT('Ctrl Pts',(-0.493843476541492,-1.,1.9827665876182));
#42837=CARTESIAN_POINT('Ctrl Pts',(-0.493843476541492,1.,1.9827665876182));
#42838=CARTESIAN_POINT('Ctrl Pts',(-0.490150627860955,-1.,1.97783973019229));
#42839=CARTESIAN_POINT('Ctrl Pts',(-0.490150627860955,1.,1.97783973019229));
#42840=CARTESIAN_POINT('Ctrl Pts',(-0.486502692907661,-1.,1.97289186263272));
#42841=CARTESIAN_POINT('Ctrl Pts',(-0.486502692907661,1.,1.97289186263272));
#42842=CARTESIAN_POINT('Ctrl Pts',(-0.482901662120687,-1.,1.96792703422358));
#42843=CARTESIAN_POINT('Ctrl Pts',(-0.482901662120687,1.,1.96792703422358));
#42844=CARTESIAN_POINT('Ctrl Pts',(-0.479349583074846,-1.,1.96294933055938));
#42845=CARTESIAN_POINT('Ctrl Pts',(-0.479349583074846,1.,1.96294933055938));
#42846=CARTESIAN_POINT('Ctrl Pts',(-0.475848034683172,-1.,1.95796111148175));
#42847=CARTESIAN_POINT('Ctrl Pts',(-0.475848034683172,1.,1.95796111148175));
#42848=CARTESIAN_POINT('Ctrl Pts',(-0.47239767226408,-1.,1.95296148278136));
#42849=CARTESIAN_POINT('Ctrl Pts',(-0.47239767226408,1.,1.95296148278136));
#42850=CARTESIAN_POINT('Ctrl Pts',(-0.468997482913158,-1.,1.94794381136524));
#42851=CARTESIAN_POINT('Ctrl Pts',(-0.468997482913158,1.,1.94794381136524));
#42852=CARTESIAN_POINT('Ctrl Pts',(-0.465645462026065,-1.,1.94289794196205));
#42853=CARTESIAN_POINT('Ctrl Pts',(-0.465645462026065,1.,1.94289794196205));
#42854=CARTESIAN_POINT('Ctrl Pts',(-0.462340031009087,-1.,1.93781486640834));
#42855=CARTESIAN_POINT('Ctrl Pts',(-0.462340031009087,1.,1.93781486640834));
#42856=CARTESIAN_POINT('Ctrl Pts',(-0.459081234547931,-1.,1.93269066517936));
#42857=CARTESIAN_POINT('Ctrl Pts',(-0.459081234547931,1.,1.93269066517936));
#42858=CARTESIAN_POINT('Ctrl Pts',(-0.455872005174335,-1.,1.92753067150461));
#42859=CARTESIAN_POINT('Ctrl Pts',(-0.455872005174335,1.,1.92753067150461));
#42860=CARTESIAN_POINT('Ctrl Pts',(-0.452719478359356,-1.,1.9223538064847));
#42861=CARTESIAN_POINT('Ctrl Pts',(-0.452719478359356,1.,1.9223538064847));
#42862=CARTESIAN_POINT('Ctrl Pts',(-0.449632260106572,-1.,1.91718342555717));
#42863=CARTESIAN_POINT('Ctrl Pts',(-0.449632260106572,1.,1.91718342555717));
#42864=CARTESIAN_POINT('Ctrl Pts',(-0.446617343485651,-1.,1.91203699981095));
#42865=CARTESIAN_POINT('Ctrl Pts',(-0.446617343485651,1.,1.91203699981095));
#42866=CARTESIAN_POINT('Ctrl Pts',(-0.44367755684917,-1.,1.90691756144906));
#42867=CARTESIAN_POINT('Ctrl Pts',(-0.44367755684917,1.,1.90691756144906));
#42868=CARTESIAN_POINT('Ctrl Pts',(-0.440807833704161,-1.,1.90180124389137));
#42869=CARTESIAN_POINT('Ctrl Pts',(-0.440807833704161,1.,1.90180124389137));
#42870=CARTESIAN_POINT('Ctrl Pts',(-0.437995003948443,-1.,1.89663648956549));
#42871=CARTESIAN_POINT('Ctrl Pts',(-0.437995003948443,1.,1.89663648956549));
#42872=CARTESIAN_POINT('Ctrl Pts',(-0.43522566096358,-1.,1.89136993975585));
#42873=CARTESIAN_POINT('Ctrl Pts',(-0.43522566096358,1.,1.89136993975585));
#42874=CARTESIAN_POINT('Ctrl Pts',(-0.432493038548833,-1.,1.88596913666828));
#42875=CARTESIAN_POINT('Ctrl Pts',(-0.432493038548833,1.,1.88596913666828));
#42876=CARTESIAN_POINT('Ctrl Pts',(-0.429803062482217,-1.,1.88044229001778));
#42877=CARTESIAN_POINT('Ctrl Pts',(-0.429803062482217,1.,1.88044229001778));
#42878=CARTESIAN_POINT('Ctrl Pts',(-0.427183828518743,-1.,1.87486989291333));
#42879=CARTESIAN_POINT('Ctrl Pts',(-0.427183828518743,1.,1.87486989291333));
#42880=CARTESIAN_POINT('Ctrl Pts',(-0.424678177290876,-1.,1.8693780394412));
#42881=CARTESIAN_POINT('Ctrl Pts',(-0.424678177290876,1.,1.8693780394412));
#42882=CARTESIAN_POINT('Ctrl Pts',(-0.422327307417885,-1.,1.86408083333863));
#42883=CARTESIAN_POINT('Ctrl Pts',(-0.422327307417885,1.,1.86408083333863));
#42884=CARTESIAN_POINT('Ctrl Pts',(-0.420157287975583,-1.,1.8590328109667));
#42885=CARTESIAN_POINT('Ctrl Pts',(-0.420157287975583,1.,1.8590328109667));
#42886=CARTESIAN_POINT('Ctrl Pts',(-0.418164129144045,-1.,1.8541763285645));
#42887=CARTESIAN_POINT('Ctrl Pts',(-0.418164129144045,1.,1.8541763285645));
#42888=CARTESIAN_POINT('Ctrl Pts',(-0.416300022039885,-1.,1.84929312930314));
#42889=CARTESIAN_POINT('Ctrl Pts',(-0.416300022039885,1.,1.84929312930314));
#42890=CARTESIAN_POINT('Ctrl Pts',(-0.414487438255542,-1.,1.84405757074218));
#42891=CARTESIAN_POINT('Ctrl Pts',(-0.414487438255542,1.,1.84405757074218));
#42892=CARTESIAN_POINT('Ctrl Pts',(-0.412633125322945,-1.,1.8380895347617));
#42893=CARTESIAN_POINT('Ctrl Pts',(-0.412633125322945,1.,1.8380895347617));
#42894=CARTESIAN_POINT('Ctrl Pts',(-0.410641256301276,-1.,1.83100408895047));
#42895=CARTESIAN_POINT('Ctrl Pts',(-0.410641256301276,1.,1.83100408895047));
#42896=CARTESIAN_POINT('Ctrl Pts',(-0.408428948106227,-1.,1.82247022677562));
#42897=CARTESIAN_POINT('Ctrl Pts',(-0.408428948106227,1.,1.82247022677562));
#42898=CARTESIAN_POINT('Ctrl Pts',(-0.405933518407175,-1.,1.81223801812013));
#42899=CARTESIAN_POINT('Ctrl Pts',(-0.405933518407175,1.,1.81223801812013));
#42900=CARTESIAN_POINT('Ctrl Pts',(-0.403107976163396,-1.,1.80012077173238));
#42901=CARTESIAN_POINT('Ctrl Pts',(-0.403107976163396,1.,1.80012077173238));
#42902=CARTESIAN_POINT('Ctrl Pts',(-0.399919403774155,-1.,1.78598826343754));
#42903=CARTESIAN_POINT('Ctrl Pts',(-0.399919403774155,1.,1.78598826343754));
#42904=CARTESIAN_POINT('Ctrl Pts',(-0.396346196110688,-1.,1.76975560043442));
#42905=CARTESIAN_POINT('Ctrl Pts',(-0.396346196110688,1.,1.76975560043442));
#42906=CARTESIAN_POINT('Ctrl Pts',(-0.392375812285395,-1.,1.75137405310193));
#42907=CARTESIAN_POINT('Ctrl Pts',(-0.392375812285395,1.,1.75137405310193));
#42908=CARTESIAN_POINT('Ctrl Pts',(-0.388877023502615,-1.,1.73493170972829));
#42909=CARTESIAN_POINT('Ctrl Pts',(-0.388877023502615,1.,1.73493170972829));
#42910=CARTESIAN_POINT('Ctrl Pts',(-0.386070790323281,-1.,1.72162022244582));
#42911=CARTESIAN_POINT('Ctrl Pts',(-0.386070790323281,1.,1.72162022244582));
#42912=CARTESIAN_POINT('Ctrl Pts',(-0.384119047314215,-1.,1.71231062891398));
#42913=CARTESIAN_POINT('Ctrl Pts',(-0.384119047314215,1.,1.71231062891398));
#42914=CARTESIAN_POINT('Ctrl Pts',(-0.383122945602004,-1.,1.7075470150345));
#42915=CARTESIAN_POINT('Ctrl Pts',(-0.383122945602004,1.,1.7075470150345));
#42916=CARTESIAN_POINT('',(-0.61342227326009,1.,2.11275013067528));
#42917=CARTESIAN_POINT('Ctrl Pts',(-0.61342227326009,1.,2.11275013067528));
#42918=CARTESIAN_POINT('Ctrl Pts',(-0.61246736556225,1.,2.11187554260142));
#42919=CARTESIAN_POINT('Ctrl Pts',(-0.610560911691113,1.,2.11012443807661));
#42920=CARTESIAN_POINT('Ctrl Pts',(-0.607711315456826,1.,2.10749199615859));
#42921=CARTESIAN_POINT('Ctrl Pts',(-0.603932030738212,1.,2.10397049887709));
#42922=CARTESIAN_POINT('Ctrl Pts',(-0.599241616422144,1.,2.09954930865331));
#42923=CARTESIAN_POINT('Ctrl Pts',(-0.594585006052824,1.,2.09510876220501));
#42924=CARTESIAN_POINT('Ctrl Pts',(-0.589962365403189,1.,2.09064881812053));
#42925=CARTESIAN_POINT('Ctrl Pts',(-0.585373918990895,1.,2.086169437277));
#42926=CARTESIAN_POINT('Ctrl Pts',(-0.580819952107257,1.,2.08167059018138));
#42927=CARTESIAN_POINT('Ctrl Pts',(-0.576300797416275,1.,2.07715226767361));
#42928=CARTESIAN_POINT('Ctrl Pts',(-0.571816823242411,1.,2.07261449292757));
#42929=CARTESIAN_POINT('Ctrl Pts',(-0.567368421181229,1.,2.06805732997383));
#42930=CARTESIAN_POINT('Ctrl Pts',(-0.562955993082574,1.,2.06348090160697));
#42931=CARTESIAN_POINT('Ctrl Pts',(-0.558579940185467,1.,2.05888537756571));
#42932=CARTESIAN_POINT('Ctrl Pts',(-0.55424065746411,1.,2.05427091604482));
#42933=CARTESIAN_POINT('Ctrl Pts',(-0.549938525150342,1.,2.04963761077974));
#42934=CARTESIAN_POINT('Ctrl Pts',(-0.545673903817348,1.,2.0449854471456));
#42935=CARTESIAN_POINT('Ctrl Pts',(-0.54144712061552,1.,2.0403142269048));
#42936=CARTESIAN_POINT('Ctrl Pts',(-0.537258489833134,1.,2.03562362953993));
#42937=CARTESIAN_POINT('Ctrl Pts',(-0.533108355132905,1.,2.03091336214401));
#42938=CARTESIAN_POINT('Ctrl Pts',(-0.528997127241911,1.,2.02618329083289));
#42939=CARTESIAN_POINT('Ctrl Pts',(-0.524925318333518,1.,2.02143356304712));
#42940=CARTESIAN_POINT('Ctrl Pts',(-0.520893590399428,1.,2.01666477917305));
#42941=CARTESIAN_POINT('Ctrl Pts',(-0.516902681728733,1.,2.01187773939257));
#42942=CARTESIAN_POINT('Ctrl Pts',(-0.512953306961814,1.,2.00707309946955));
#42943=CARTESIAN_POINT('Ctrl Pts',(-0.509046069886152,1.,2.00225107134733));
#42944=CARTESIAN_POINT('Ctrl Pts',(-0.505181361323011,1.,1.99741107463567));
#42945=CARTESIAN_POINT('Ctrl Pts',(-0.501359287727129,1.,1.9925514912615));
#42946=CARTESIAN_POINT('Ctrl Pts',(-0.497579909545564,1.,1.98767044752929));
#42947=CARTESIAN_POINT('Ctrl Pts',(-0.493843476541492,1.,1.9827665876182));
#42948=CARTESIAN_POINT('Ctrl Pts',(-0.490150627860955,1.,1.97783973019229));
#42949=CARTESIAN_POINT('Ctrl Pts',(-0.486502692907661,1.,1.97289186263272));
#42950=CARTESIAN_POINT('Ctrl Pts',(-0.482901662120687,1.,1.96792703422358));
#42951=CARTESIAN_POINT('Ctrl Pts',(-0.479349583074846,1.,1.96294933055938));
#42952=CARTESIAN_POINT('Ctrl Pts',(-0.475848034683172,1.,1.95796111148175));
#42953=CARTESIAN_POINT('Ctrl Pts',(-0.47239767226408,1.,1.95296148278136));
#42954=CARTESIAN_POINT('Ctrl Pts',(-0.468997482913158,1.,1.94794381136524));
#42955=CARTESIAN_POINT('Ctrl Pts',(-0.465645462026065,1.,1.94289794196205));
#42956=CARTESIAN_POINT('Ctrl Pts',(-0.462340031009087,1.,1.93781486640834));
#42957=CARTESIAN_POINT('Ctrl Pts',(-0.459081234547931,1.,1.93269066517936));
#42958=CARTESIAN_POINT('Ctrl Pts',(-0.455872005174335,1.,1.92753067150461));
#42959=CARTESIAN_POINT('Ctrl Pts',(-0.452719478359356,1.,1.9223538064847));
#42960=CARTESIAN_POINT('Ctrl Pts',(-0.449632260106572,1.,1.91718342555717));
#42961=CARTESIAN_POINT('Ctrl Pts',(-0.446617343485651,1.,1.91203699981095));
#42962=CARTESIAN_POINT('Ctrl Pts',(-0.44367755684917,1.,1.90691756144906));
#42963=CARTESIAN_POINT('Ctrl Pts',(-0.440807833704161,1.,1.90180124389137));
#42964=CARTESIAN_POINT('Ctrl Pts',(-0.437995003948443,1.,1.89663648956549));
#42965=CARTESIAN_POINT('Ctrl Pts',(-0.43522566096358,1.,1.89136993975585));
#42966=CARTESIAN_POINT('Ctrl Pts',(-0.432493038548833,1.,1.88596913666828));
#42967=CARTESIAN_POINT('Ctrl Pts',(-0.429803062482217,1.,1.88044229001778));
#42968=CARTESIAN_POINT('Ctrl Pts',(-0.427183828518743,1.,1.87486989291333));
#42969=CARTESIAN_POINT('Ctrl Pts',(-0.424678177290876,1.,1.8693780394412));
#42970=CARTESIAN_POINT('Ctrl Pts',(-0.422327307417885,1.,1.86408083333863));
#42971=CARTESIAN_POINT('Ctrl Pts',(-0.420157287975583,1.,1.8590328109667));
#42972=CARTESIAN_POINT('Ctrl Pts',(-0.418164129144045,1.,1.8541763285645));
#42973=CARTESIAN_POINT('Ctrl Pts',(-0.416300022039885,1.,1.84929312930314));
#42974=CARTESIAN_POINT('Ctrl Pts',(-0.414487438255542,1.,1.84405757074218));
#42975=CARTESIAN_POINT('Ctrl Pts',(-0.412633125322945,1.,1.8380895347617));
#42976=CARTESIAN_POINT('Ctrl Pts',(-0.410641256301276,1.,1.83100408895047));
#42977=CARTESIAN_POINT('Ctrl Pts',(-0.408428948106227,1.,1.82247022677562));
#42978=CARTESIAN_POINT('Ctrl Pts',(-0.405933518407175,1.,1.81223801812013));
#42979=CARTESIAN_POINT('Ctrl Pts',(-0.403107976163396,1.,1.80012077173238));
#42980=CARTESIAN_POINT('Ctrl Pts',(-0.399919403774155,1.,1.78598826343754));
#42981=CARTESIAN_POINT('Ctrl Pts',(-0.396346196110688,1.,1.76975560043442));
#42982=CARTESIAN_POINT('Ctrl Pts',(-0.392375812285395,1.,1.75137405310193));
#42983=CARTESIAN_POINT('Ctrl Pts',(-0.388877023502615,1.,1.73493170972829));
#42984=CARTESIAN_POINT('Ctrl Pts',(-0.386070790323281,1.,1.72162022244582));
#42985=CARTESIAN_POINT('Ctrl Pts',(-0.384119047314215,1.,1.71231062891398));
#42986=CARTESIAN_POINT('Ctrl Pts',(-0.383122945602004,1.,1.7075470150345));
#42987=CARTESIAN_POINT('',(-0.61342227326009,0.,2.11275013067528));
#42988=CARTESIAN_POINT('Origin',(-0.745574324794401,0.,2.0698113262342));
#42989=CARTESIAN_POINT('',(-0.745574324794401,1.,2.0698113262342));
#42990=CARTESIAN_POINT('',(-0.61342227326009,1.,2.11275013067528));
#42991=CARTESIAN_POINT('',(-0.745574324794401,0.,2.0698113262342));
#42992=CARTESIAN_POINT('Ctrl Pts',(-0.693717979106306,-1.,1.60662857109684));
#42993=CARTESIAN_POINT('Ctrl Pts',(-0.693717979106306,1.,1.60662857109684));
#42994=CARTESIAN_POINT('Ctrl Pts',(-0.695712097881194,-1.,1.61106790958151));
#42995=CARTESIAN_POINT('Ctrl Pts',(-0.695712097881194,1.,1.61106790958151));
#42996=CARTESIAN_POINT('Ctrl Pts',(-0.699605146405088,-1.,1.61974673472612));
#42997=CARTESIAN_POINT('Ctrl Pts',(-0.699605146405088,1.,1.61974673472612));
#42998=CARTESIAN_POINT('Ctrl Pts',(-0.705159151988319,-1.,1.63216541664676));
#42999=CARTESIAN_POINT('Ctrl Pts',(-0.705159151988319,1.,1.63216541664676));
#43000=CARTESIAN_POINT('Ctrl Pts',(-0.711993139355394,-1.,1.64752408832016));
#43001=CARTESIAN_POINT('Ctrl Pts',(-0.711993139355394,1.,1.64752408832016));
#43002=CARTESIAN_POINT('Ctrl Pts',(-0.719585433804282,-1.,1.6647288055568));
#43003=CARTESIAN_POINT('Ctrl Pts',(-0.719585433804282,1.,1.6647288055568));
#43004=CARTESIAN_POINT('Ctrl Pts',(-0.726235967997433,-1.,1.67996158455503));
#43005=CARTESIAN_POINT('Ctrl Pts',(-0.726235967997433,1.,1.67996158455503));
#43006=CARTESIAN_POINT('Ctrl Pts',(-0.731963238697195,-1.,1.69326921975743));
#43007=CARTESIAN_POINT('Ctrl Pts',(-0.731963238697195,1.,1.69326921975743));
#43008=CARTESIAN_POINT('Ctrl Pts',(-0.736799665724771,-1.,1.70473309006121));
#43009=CARTESIAN_POINT('Ctrl Pts',(-0.736799665724771,1.,1.70473309006121));
#43010=CARTESIAN_POINT('Ctrl Pts',(-0.740795162032088,-1.,1.71447789751927));
#43011=CARTESIAN_POINT('Ctrl Pts',(-0.740795162032088,1.,1.71447789751927));
#43012=CARTESIAN_POINT('Ctrl Pts',(-0.744021445433764,-1.,1.7226822991693));
#43013=CARTESIAN_POINT('Ctrl Pts',(-0.744021445433764,1.,1.7226822991693));
#43014=CARTESIAN_POINT('Ctrl Pts',(-0.746574710096436,-1.,1.72958533647399));
#43015=CARTESIAN_POINT('Ctrl Pts',(-0.746574710096436,1.,1.72958533647399));
#43016=CARTESIAN_POINT('Ctrl Pts',(-0.748582462954855,-1.,1.73550351679848));
#43017=CARTESIAN_POINT('Ctrl Pts',(-0.748582462954855,1.,1.73550351679848));
#43018=CARTESIAN_POINT('Ctrl Pts',(-0.75019343597954,-1.,1.74080458266705));
#43019=CARTESIAN_POINT('Ctrl Pts',(-0.75019343597954,1.,1.74080458266705));
#43020=CARTESIAN_POINT('Ctrl Pts',(-0.751555614163629,-1.,1.74585086852298));
#43021=CARTESIAN_POINT('Ctrl Pts',(-0.751555614163629,1.,1.74585086852298));
#43022=CARTESIAN_POINT('Ctrl Pts',(-0.752797683531377,-1.,1.75095139468809));
#43023=CARTESIAN_POINT('Ctrl Pts',(-0.752797683531377,1.,1.75095139468809));
#43024=CARTESIAN_POINT('Ctrl Pts',(-0.75400925402848,-1.,1.75631083600175));
#43025=CARTESIAN_POINT('Ctrl Pts',(-0.75400925402848,1.,1.75631083600175));
#43026=CARTESIAN_POINT('Ctrl Pts',(-0.755220979975262,-1.,1.7619781724032));
#43027=CARTESIAN_POINT('Ctrl Pts',(-0.755220979975262,1.,1.7619781724032));
#43028=CARTESIAN_POINT('Ctrl Pts',(-0.756421896028403,-1.,1.76789396003141));
#43029=CARTESIAN_POINT('Ctrl Pts',(-0.756421896028403,1.,1.76789396003141));
#43030=CARTESIAN_POINT('Ctrl Pts',(-0.757578264077238,-1.,1.77394167108342));
#43031=CARTESIAN_POINT('Ctrl Pts',(-0.757578264077238,1.,1.77394167108342));
#43032=CARTESIAN_POINT('Ctrl Pts',(-0.75865062667738,-1.,1.77999411220912));
#43033=CARTESIAN_POINT('Ctrl Pts',(-0.75865062667738,1.,1.77999411220912));
#43034=CARTESIAN_POINT('Ctrl Pts',(-0.759614401109868,-1.,1.78596964884526));
#43035=CARTESIAN_POINT('Ctrl Pts',(-0.759614401109868,1.,1.78596964884526));
#43036=CARTESIAN_POINT('Ctrl Pts',(-0.760469555880425,-1.,1.79185815610802));
#43037=CARTESIAN_POINT('Ctrl Pts',(-0.760469555880425,1.,1.79185815610802));
#43038=CARTESIAN_POINT('Ctrl Pts',(-0.761229695230359,-1.,1.79768986997735));
#43039=CARTESIAN_POINT('Ctrl Pts',(-0.761229695230359,1.,1.79768986997735));
#43040=CARTESIAN_POINT('Ctrl Pts',(-0.761915336443516,-1.,1.80351583877334));
#43041=CARTESIAN_POINT('Ctrl Pts',(-0.761915336443516,1.,1.80351583877334));
#43042=CARTESIAN_POINT('Ctrl Pts',(-0.762546129464036,-1.,1.80938551463989));
#43043=CARTESIAN_POINT('Ctrl Pts',(-0.762546129464036,1.,1.80938551463989));
#43044=CARTESIAN_POINT('Ctrl Pts',(-0.763132003836783,-1.,1.81532118405566));
#43045=CARTESIAN_POINT('Ctrl Pts',(-0.763132003836783,1.,1.81532118405566));
#43046=CARTESIAN_POINT('Ctrl Pts',(-0.763673465462854,-1.,1.82131873145297));
#43047=CARTESIAN_POINT('Ctrl Pts',(-0.763673465462854,1.,1.82131873145297));
#43048=CARTESIAN_POINT('Ctrl Pts',(-0.764165902606055,-1.,1.8273599120008));
#43049=CARTESIAN_POINT('Ctrl Pts',(-0.764165902606055,1.,1.8273599120008));
#43050=CARTESIAN_POINT('Ctrl Pts',(-0.764602549687845,-1.,1.8334207722714));
#43051=CARTESIAN_POINT('Ctrl Pts',(-0.764602549687845,1.,1.8334207722714));
#43052=CARTESIAN_POINT('Ctrl Pts',(-0.764978057881687,-1.,1.83948181064823));
#43053=CARTESIAN_POINT('Ctrl Pts',(-0.764978057881687,1.,1.83948181064823));
#43054=CARTESIAN_POINT('Ctrl Pts',(-0.765291664861971,-1.,1.8455369887591));
#43055=CARTESIAN_POINT('Ctrl Pts',(-0.765291664861971,1.,1.8455369887591));
#43056=CARTESIAN_POINT('Ctrl Pts',(-0.765545710619023,-1.,1.85158945130054));
#43057=CARTESIAN_POINT('Ctrl Pts',(-0.765545710619023,1.,1.85158945130054));
#43058=CARTESIAN_POINT('Ctrl Pts',(-0.765744212909305,-1.,1.85764741390391));
#43059=CARTESIAN_POINT('Ctrl Pts',(-0.765744212909305,1.,1.85764741390391));
#43060=CARTESIAN_POINT('Ctrl Pts',(-0.765891519092557,-1.,1.86372027063314));
#43061=CARTESIAN_POINT('Ctrl Pts',(-0.765891519092557,1.,1.86372027063314));
#43062=CARTESIAN_POINT('Ctrl Pts',(-0.765990708546111,-1.,1.86981398314345));
#43063=CARTESIAN_POINT('Ctrl Pts',(-0.765990708546111,1.,1.86981398314345));
#43064=CARTESIAN_POINT('Ctrl Pts',(-0.766042837036759,-1.,1.87592888967886));
#43065=CARTESIAN_POINT('Ctrl Pts',(-0.766042837036759,1.,1.87592888967886));
#43066=CARTESIAN_POINT('Ctrl Pts',(-0.766047794851869,-1.,1.88206215302561));
#43067=CARTESIAN_POINT('Ctrl Pts',(-0.766047794851869,1.,1.88206215302561));
#43068=CARTESIAN_POINT('Ctrl Pts',(-0.76600483706209,-1.,1.88820926433409));
#43069=CARTESIAN_POINT('Ctrl Pts',(-0.76600483706209,1.,1.88820926433409));
#43070=CARTESIAN_POINT('Ctrl Pts',(-0.765913193856979,-1.,1.89436577771389));
#43071=CARTESIAN_POINT('Ctrl Pts',(-0.765913193856979,1.,1.89436577771389));
#43072=CARTESIAN_POINT('Ctrl Pts',(-0.765772772593395,-1.,1.90052930393599));
#43073=CARTESIAN_POINT('Ctrl Pts',(-0.765772772593395,1.,1.90052930393599));
#43074=CARTESIAN_POINT('Ctrl Pts',(-0.765584196937936,-1.,1.90669961402362));
#43075=CARTESIAN_POINT('Ctrl Pts',(-0.765584196937936,1.,1.90669961402362));
#43076=CARTESIAN_POINT('Ctrl Pts',(-0.765348465884739,-1.,1.91287765805174));
#43077=CARTESIAN_POINT('Ctrl Pts',(-0.765348465884739,1.,1.91287765805174));
#43078=CARTESIAN_POINT('Ctrl Pts',(-0.765066729667095,-1.,1.91906491634197));
#43079=CARTESIAN_POINT('Ctrl Pts',(-0.765066729667095,1.,1.91906491634197));
#43080=CARTESIAN_POINT('Ctrl Pts',(-0.764740025488189,-1.,1.92526263537041));
#43081=CARTESIAN_POINT('Ctrl Pts',(-0.764740025488189,1.,1.92526263537041));
#43082=CARTESIAN_POINT('Ctrl Pts',(-0.764369010673889,-1.,1.93147105496367));
#43083=CARTESIAN_POINT('Ctrl Pts',(-0.764369010673889,1.,1.93147105496367));
#43084=CARTESIAN_POINT('Ctrl Pts',(-0.763954049121393,-1.,1.93768964875867));
#43085=CARTESIAN_POINT('Ctrl Pts',(-0.763954049121393,1.,1.93768964875867));
#43086=CARTESIAN_POINT('Ctrl Pts',(-0.76349533353858,-1.,1.94391746617626));
#43087=CARTESIAN_POINT('Ctrl Pts',(-0.76349533353858,1.,1.94391746617626));
#43088=CARTESIAN_POINT('Ctrl Pts',(-0.762992990878774,-1.,1.95015342590025));
#43089=CARTESIAN_POINT('Ctrl Pts',(-0.762992990878774,1.,1.95015342590025));
#43090=CARTESIAN_POINT('Ctrl Pts',(-0.762447203806263,-1.,1.95639665309893));
#43091=CARTESIAN_POINT('Ctrl Pts',(-0.762447203806263,1.,1.95639665309893));
#43092=CARTESIAN_POINT('Ctrl Pts',(-0.761858300014575,-1.,1.96264672744229));
#43093=CARTESIAN_POINT('Ctrl Pts',(-0.761858300014575,1.,1.96264672744229));
#43094=CARTESIAN_POINT('Ctrl Pts',(-0.761226690483986,-1.,1.96890351582545));
#43095=CARTESIAN_POINT('Ctrl Pts',(-0.761226690483986,1.,1.96890351582545));
#43096=CARTESIAN_POINT('Ctrl Pts',(-0.760552825409855,-1.,1.97516705321521));
#43097=CARTESIAN_POINT('Ctrl Pts',(-0.760552825409855,1.,1.97516705321521));
#43098=CARTESIAN_POINT('Ctrl Pts',(-0.759837147452135,-1.,1.98143741418156));
#43099=CARTESIAN_POINT('Ctrl Pts',(-0.759837147452135,1.,1.98143741418156));
#43100=CARTESIAN_POINT('Ctrl Pts',(-0.759080037802243,-1.,1.98771456680806));
#43101=CARTESIAN_POINT('Ctrl Pts',(-0.759080037802243,1.,1.98771456680806));
#43102=CARTESIAN_POINT('Ctrl Pts',(-0.758281796766377,-1.,1.9939983109871));
#43103=CARTESIAN_POINT('Ctrl Pts',(-0.758281796766377,1.,1.9939983109871));
#43104=CARTESIAN_POINT('Ctrl Pts',(-0.757442676862341,-1.,2.00028834739072));
#43105=CARTESIAN_POINT('Ctrl Pts',(-0.757442676862341,1.,2.00028834739072));
#43106=CARTESIAN_POINT('Ctrl Pts',(-0.756562904646496,-1.,2.00658431587682));
#43107=CARTESIAN_POINT('Ctrl Pts',(-0.756562904646496,1.,2.00658431587682));
#43108=CARTESIAN_POINT('Ctrl Pts',(-0.7556427049581,-1.,2.01288584328149));
#43109=CARTESIAN_POINT('Ctrl Pts',(-0.7556427049581,1.,2.01288584328149));
#43110=CARTESIAN_POINT('Ctrl Pts',(-0.75468233072352,-1.,2.01919259406003));
#43111=CARTESIAN_POINT('Ctrl Pts',(-0.75468233072352,1.,2.01919259406003));
#43112=CARTESIAN_POINT('Ctrl Pts',(-0.753682061113766,-1.,2.02550428623587));
#43113=CARTESIAN_POINT('Ctrl Pts',(-0.753682061113766,1.,2.02550428623587));
#43114=CARTESIAN_POINT('Ctrl Pts',(-0.752642180488104,-1.,2.03182068456467));
#43115=CARTESIAN_POINT('Ctrl Pts',(-0.752642180488104,1.,2.03182068456467));
#43116=CARTESIAN_POINT('Ctrl Pts',(-0.751562963361384,-1.,2.03814160092173));
#43117=CARTESIAN_POINT('Ctrl Pts',(-0.751562963361384,1.,2.03814160092173));
#43118=CARTESIAN_POINT('Ctrl Pts',(-0.750444657874758,-1.,2.04446689147754));
#43119=CARTESIAN_POINT('Ctrl Pts',(-0.750444657874758,1.,2.04446689147754));
#43120=CARTESIAN_POINT('Ctrl Pts',(-0.749287468663053,-1.,2.05079645591606));
#43121=CARTESIAN_POINT('Ctrl Pts',(-0.749287468663053,1.,2.05079645591606));
#43122=CARTESIAN_POINT('Ctrl Pts',(-0.748091554181101,-1.,2.05713023030263));
#43123=CARTESIAN_POINT('Ctrl Pts',(-0.748091554181101,1.,2.05713023030263));
#43124=CARTESIAN_POINT('Ctrl Pts',(-0.747103932785504,-1.,2.06220058927162));
#43125=CARTESIAN_POINT('Ctrl Pts',(-0.747103932785504,1.,2.06220058927162));
#43126=CARTESIAN_POINT('Ctrl Pts',(-0.746345871542696,-1.,2.06600523016401));
#43127=CARTESIAN_POINT('Ctrl Pts',(-0.746345871542696,1.,2.06600523016401));
#43128=CARTESIAN_POINT('Ctrl Pts',(-0.74583279137781,-1.,2.06854248895575));
#43129=CARTESIAN_POINT('Ctrl Pts',(-0.74583279137781,1.,2.06854248895575));
#43130=CARTESIAN_POINT('Ctrl Pts',(-0.745574324794401,-1.,2.0698113262342));
#43131=CARTESIAN_POINT('Ctrl Pts',(-0.745574324794401,1.,2.0698113262342));
#43132=CARTESIAN_POINT('',(-0.693717979106306,1.,1.60662857109684));
#43133=CARTESIAN_POINT('Ctrl Pts',(-0.693717979106306,1.,1.60662857109684));
#43134=CARTESIAN_POINT('Ctrl Pts',(-0.695712097881194,1.,1.61106790958151));
#43135=CARTESIAN_POINT('Ctrl Pts',(-0.699605146405088,1.,1.61974673472612));
#43136=CARTESIAN_POINT('Ctrl Pts',(-0.705159151988319,1.,1.63216541664676));
#43137=CARTESIAN_POINT('Ctrl Pts',(-0.711993139355394,1.,1.64752408832016));
#43138=CARTESIAN_POINT('Ctrl Pts',(-0.719585433804282,1.,1.6647288055568));
#43139=CARTESIAN_POINT('Ctrl Pts',(-0.726235967997433,1.,1.67996158455503));
#43140=CARTESIAN_POINT('Ctrl Pts',(-0.731963238697195,1.,1.69326921975743));
#43141=CARTESIAN_POINT('Ctrl Pts',(-0.736799665724771,1.,1.70473309006121));
#43142=CARTESIAN_POINT('Ctrl Pts',(-0.740795162032088,1.,1.71447789751927));
#43143=CARTESIAN_POINT('Ctrl Pts',(-0.744021445433764,1.,1.7226822991693));
#43144=CARTESIAN_POINT('Ctrl Pts',(-0.746574710096436,1.,1.72958533647399));
#43145=CARTESIAN_POINT('Ctrl Pts',(-0.748582462954855,1.,1.73550351679848));
#43146=CARTESIAN_POINT('Ctrl Pts',(-0.75019343597954,1.,1.74080458266705));
#43147=CARTESIAN_POINT('Ctrl Pts',(-0.751555614163629,1.,1.74585086852298));
#43148=CARTESIAN_POINT('Ctrl Pts',(-0.752797683531377,1.,1.75095139468809));
#43149=CARTESIAN_POINT('Ctrl Pts',(-0.75400925402848,1.,1.75631083600175));
#43150=CARTESIAN_POINT('Ctrl Pts',(-0.755220979975262,1.,1.7619781724032));
#43151=CARTESIAN_POINT('Ctrl Pts',(-0.756421896028403,1.,1.76789396003141));
#43152=CARTESIAN_POINT('Ctrl Pts',(-0.757578264077238,1.,1.77394167108342));
#43153=CARTESIAN_POINT('Ctrl Pts',(-0.75865062667738,1.,1.77999411220912));
#43154=CARTESIAN_POINT('Ctrl Pts',(-0.759614401109868,1.,1.78596964884526));
#43155=CARTESIAN_POINT('Ctrl Pts',(-0.760469555880425,1.,1.79185815610802));
#43156=CARTESIAN_POINT('Ctrl Pts',(-0.761229695230359,1.,1.79768986997735));
#43157=CARTESIAN_POINT('Ctrl Pts',(-0.761915336443516,1.,1.80351583877334));
#43158=CARTESIAN_POINT('Ctrl Pts',(-0.762546129464036,1.,1.80938551463989));
#43159=CARTESIAN_POINT('Ctrl Pts',(-0.763132003836783,1.,1.81532118405566));
#43160=CARTESIAN_POINT('Ctrl Pts',(-0.763673465462854,1.,1.82131873145297));
#43161=CARTESIAN_POINT('Ctrl Pts',(-0.764165902606055,1.,1.8273599120008));
#43162=CARTESIAN_POINT('Ctrl Pts',(-0.764602549687845,1.,1.8334207722714));
#43163=CARTESIAN_POINT('Ctrl Pts',(-0.764978057881687,1.,1.83948181064823));
#43164=CARTESIAN_POINT('Ctrl Pts',(-0.765291664861971,1.,1.8455369887591));
#43165=CARTESIAN_POINT('Ctrl Pts',(-0.765545710619023,1.,1.85158945130054));
#43166=CARTESIAN_POINT('Ctrl Pts',(-0.765744212909305,1.,1.85764741390391));
#43167=CARTESIAN_POINT('Ctrl Pts',(-0.765891519092557,1.,1.86372027063314));
#43168=CARTESIAN_POINT('Ctrl Pts',(-0.765990708546111,1.,1.86981398314345));
#43169=CARTESIAN_POINT('Ctrl Pts',(-0.766042837036759,1.,1.87592888967886));
#43170=CARTESIAN_POINT('Ctrl Pts',(-0.766047794851869,1.,1.88206215302561));
#43171=CARTESIAN_POINT('Ctrl Pts',(-0.76600483706209,1.,1.88820926433409));
#43172=CARTESIAN_POINT('Ctrl Pts',(-0.765913193856979,1.,1.89436577771389));
#43173=CARTESIAN_POINT('Ctrl Pts',(-0.765772772593395,1.,1.90052930393599));
#43174=CARTESIAN_POINT('Ctrl Pts',(-0.765584196937936,1.,1.90669961402362));
#43175=CARTESIAN_POINT('Ctrl Pts',(-0.765348465884739,1.,1.91287765805174));
#43176=CARTESIAN_POINT('Ctrl Pts',(-0.765066729667095,1.,1.91906491634197));
#43177=CARTESIAN_POINT('Ctrl Pts',(-0.764740025488189,1.,1.92526263537041));
#43178=CARTESIAN_POINT('Ctrl Pts',(-0.764369010673889,1.,1.93147105496367));
#43179=CARTESIAN_POINT('Ctrl Pts',(-0.763954049121393,1.,1.93768964875867));
#43180=CARTESIAN_POINT('Ctrl Pts',(-0.76349533353858,1.,1.94391746617626));
#43181=CARTESIAN_POINT('Ctrl Pts',(-0.762992990878774,1.,1.95015342590025));
#43182=CARTESIAN_POINT('Ctrl Pts',(-0.762447203806263,1.,1.95639665309893));
#43183=CARTESIAN_POINT('Ctrl Pts',(-0.761858300014575,1.,1.96264672744229));
#43184=CARTESIAN_POINT('Ctrl Pts',(-0.761226690483986,1.,1.96890351582545));
#43185=CARTESIAN_POINT('Ctrl Pts',(-0.760552825409855,1.,1.97516705321521));
#43186=CARTESIAN_POINT('Ctrl Pts',(-0.759837147452135,1.,1.98143741418156));
#43187=CARTESIAN_POINT('Ctrl Pts',(-0.759080037802243,1.,1.98771456680806));
#43188=CARTESIAN_POINT('Ctrl Pts',(-0.758281796766377,1.,1.9939983109871));
#43189=CARTESIAN_POINT('Ctrl Pts',(-0.757442676862341,1.,2.00028834739072));
#43190=CARTESIAN_POINT('Ctrl Pts',(-0.756562904646496,1.,2.00658431587682));
#43191=CARTESIAN_POINT('Ctrl Pts',(-0.7556427049581,1.,2.01288584328149));
#43192=CARTESIAN_POINT('Ctrl Pts',(-0.75468233072352,1.,2.01919259406003));
#43193=CARTESIAN_POINT('Ctrl Pts',(-0.753682061113766,1.,2.02550428623587));
#43194=CARTESIAN_POINT('Ctrl Pts',(-0.752642180488104,1.,2.03182068456467));
#43195=CARTESIAN_POINT('Ctrl Pts',(-0.751562963361384,1.,2.03814160092173));
#43196=CARTESIAN_POINT('Ctrl Pts',(-0.750444657874758,1.,2.04446689147754));
#43197=CARTESIAN_POINT('Ctrl Pts',(-0.749287468663053,1.,2.05079645591606));
#43198=CARTESIAN_POINT('Ctrl Pts',(-0.748091554181101,1.,2.05713023030263));
#43199=CARTESIAN_POINT('Ctrl Pts',(-0.747103932785504,1.,2.06220058927162));
#43200=CARTESIAN_POINT('Ctrl Pts',(-0.746345871542696,1.,2.06600523016401));
#43201=CARTESIAN_POINT('Ctrl Pts',(-0.74583279137781,1.,2.06854248895575));
#43202=CARTESIAN_POINT('Ctrl Pts',(-0.745574324794401,1.,2.0698113262342));
#43203=CARTESIAN_POINT('',(-0.693717979106306,0.,1.60662857109684));
#43204=CARTESIAN_POINT('Origin',(0.,0.,0.));
#43205=CARTESIAN_POINT('',(-0.892032620296855,1.,1.5055822144029));
#43206=CARTESIAN_POINT('Origin',(0.,1.,0.));
#43207=CARTESIAN_POINT('',(-0.892032620296855,0.,1.5055822144029));
#43208=CARTESIAN_POINT('Ctrl Pts',(-1.23627494547115,-1.,1.81978687191668));
#43209=CARTESIAN_POINT('Ctrl Pts',(-1.23627494547115,1.,1.81978687191668));
#43210=CARTESIAN_POINT('Ctrl Pts',(-1.23509651170476,-1.,1.81925017193666));
#43211=CARTESIAN_POINT('Ctrl Pts',(-1.23509651170476,1.,1.81925017193666));
#43212=CARTESIAN_POINT('Ctrl Pts',(-1.2327422452705,-1.,1.81817389921279));
#43213=CARTESIAN_POINT('Ctrl Pts',(-1.2327422452705,1.,1.81817389921279));
#43214=CARTESIAN_POINT('Ctrl Pts',(-1.2292186489137,-1.,1.8165508718364));
#43215=CARTESIAN_POINT('Ctrl Pts',(-1.2292186489137,1.,1.8165508718364));
#43216=CARTESIAN_POINT('Ctrl Pts',(-1.2245361330495,-1.,1.81436959210434));
#43217=CARTESIAN_POINT('Ctrl Pts',(-1.2245361330495,1.,1.81436959210434));
#43218=CARTESIAN_POINT('Ctrl Pts',(-1.21870906103557,-1.,1.81161420806656));
#43219=CARTESIAN_POINT('Ctrl Pts',(-1.21870906103557,1.,1.81161420806656));
#43220=CARTESIAN_POINT('Ctrl Pts',(-1.21290815708314,-1.,1.80882996917129));
#43221=CARTESIAN_POINT('Ctrl Pts',(-1.21290815708314,1.,1.80882996917129));
#43222=CARTESIAN_POINT('Ctrl Pts',(-1.20713356605475,-1.,1.80601678480707));
#43223=CARTESIAN_POINT('Ctrl Pts',(-1.20713356605475,1.,1.80601678480707));
#43224=CARTESIAN_POINT('Ctrl Pts',(-1.20138548938974,-1.,1.80317454838603));
#43225=CARTESIAN_POINT('Ctrl Pts',(-1.20138548938974,1.,1.80317454838603));
#43226=CARTESIAN_POINT('Ctrl Pts',(-1.19566418930242,-1.,1.80030314369879));
#43227=CARTESIAN_POINT('Ctrl Pts',(-1.19566418930242,1.,1.80030314369879));
#43228=CARTESIAN_POINT('Ctrl Pts',(-1.18996997934445,-1.,1.79740245923478));
#43229=CARTESIAN_POINT('Ctrl Pts',(-1.18996997934445,1.,1.79740245923478));
#43230=CARTESIAN_POINT('Ctrl Pts',(-1.18430321697432,-1.,1.79447240321515));
#43231=CARTESIAN_POINT('Ctrl Pts',(-1.18430321697432,1.,1.79447240321515));
#43232=CARTESIAN_POINT('Ctrl Pts',(-1.17866429440809,-1.,1.79151291552689));
#43233=CARTESIAN_POINT('Ctrl Pts',(-1.17866429440809,1.,1.79151291552689));
#43234=CARTESIAN_POINT('Ctrl Pts',(-1.17305363177328,-1.,1.78852398877616));
#43235=CARTESIAN_POINT('Ctrl Pts',(-1.17305363177328,1.,1.78852398877616));
#43236=CARTESIAN_POINT('Ctrl Pts',(-1.16747166312303,-1.,1.78550566040443));
#43237=CARTESIAN_POINT('Ctrl Pts',(-1.16747166312303,1.,1.78550566040443));
#43238=CARTESIAN_POINT('Ctrl Pts',(-1.16191881298499,-1.,1.78245795881009));
#43239=CARTESIAN_POINT('Ctrl Pts',(-1.16191881298499,1.,1.78245795881009));
#43240=CARTESIAN_POINT('Ctrl Pts',(-1.15639547194698,-1.,1.77938085564275));
#43241=CARTESIAN_POINT('Ctrl Pts',(-1.15639547194698,1.,1.77938085564275));
#43242=CARTESIAN_POINT('Ctrl Pts',(-1.15090197841515,-1.,1.7762742255701));
#43243=CARTESIAN_POINT('Ctrl Pts',(-1.15090197841515,1.,1.7762742255701));
#43244=CARTESIAN_POINT('Ctrl Pts',(-1.1454385822692,-1.,1.77313777896194));
#43245=CARTESIAN_POINT('Ctrl Pts',(-1.1454385822692,1.,1.77313777896194));
#43246=CARTESIAN_POINT('Ctrl Pts',(-1.14000548336975,-1.,1.76997111386769));
#43247=CARTESIAN_POINT('Ctrl Pts',(-1.14000548336975,1.,1.76997111386769));
#43248=CARTESIAN_POINT('Ctrl Pts',(-1.1346029180462,-1.,1.76677384551862));
#43249=CARTESIAN_POINT('Ctrl Pts',(-1.1346029180462,1.,1.76677384551862));
#43250=CARTESIAN_POINT('Ctrl Pts',(-1.12923123555075,-1.,1.7635457196617));
#43251=CARTESIAN_POINT('Ctrl Pts',(-1.12923123555075,1.,1.7635457196617));
#43252=CARTESIAN_POINT('Ctrl Pts',(-1.12389096855086,-1.,1.76028671825096));
#43253=CARTESIAN_POINT('Ctrl Pts',(-1.12389096855086,1.,1.76028671825096));
#43254=CARTESIAN_POINT('Ctrl Pts',(-1.11858293216763,-1.,1.75699720772105));
#43255=CARTESIAN_POINT('Ctrl Pts',(-1.11858293216763,1.,1.75699720772105));
#43256=CARTESIAN_POINT('Ctrl Pts',(-1.11330807582551,-1.,1.7536777209463));
#43257=CARTESIAN_POINT('Ctrl Pts',(-1.11330807582551,1.,1.7536777209463));
#43258=CARTESIAN_POINT('Ctrl Pts',(-1.10806728183007,-1.,1.7503286607592));
#43259=CARTESIAN_POINT('Ctrl Pts',(-1.10806728183007,1.,1.7503286607592));
#43260=CARTESIAN_POINT('Ctrl Pts',(-1.10286118991143,-1.,1.74695004214923));
#43261=CARTESIAN_POINT('Ctrl Pts',(-1.10286118991143,1.,1.74695004214923));
#43262=CARTESIAN_POINT('Ctrl Pts',(-1.09768999241225,-1.,1.74354119236208));
#43263=CARTESIAN_POINT('Ctrl Pts',(-1.09768999241225,1.,1.74354119236208));
#43264=CARTESIAN_POINT('Ctrl Pts',(-1.09255329056493,-1.,1.74010053962247));
#43265=CARTESIAN_POINT('Ctrl Pts',(-1.09255329056493,1.,1.74010053962247));
#43266=CARTESIAN_POINT('Ctrl Pts',(-1.08745056285427,-1.,1.73662628326091));
#43267=CARTESIAN_POINT('Ctrl Pts',(-1.08745056285427,1.,1.73662628326091));
#43268=CARTESIAN_POINT('Ctrl Pts',(-1.08238162784749,-1.,1.73311705663407));
#43269=CARTESIAN_POINT('Ctrl Pts',(-1.08238162784749,1.,1.73311705663407));
#43270=CARTESIAN_POINT('Ctrl Pts',(-1.0773470373727,-1.,1.72957248977424));
#43271=CARTESIAN_POINT('Ctrl Pts',(-1.0773470373727,1.,1.72957248977424));
#43272=CARTESIAN_POINT('Ctrl Pts',(-1.07234866990252,-1.,1.72599406198488));
#43273=CARTESIAN_POINT('Ctrl Pts',(-1.07234866990252,1.,1.72599406198488));
#43274=CARTESIAN_POINT('Ctrl Pts',(-1.06738966975462,-1.,1.72238500928453));
#43275=CARTESIAN_POINT('Ctrl Pts',(-1.06738966975462,1.,1.72238500928453));
#43276=CARTESIAN_POINT('Ctrl Pts',(-1.06247324680647,-1.,1.71874858456904));
#43277=CARTESIAN_POINT('Ctrl Pts',(-1.06247324680647,1.,1.71874858456904));
#43278=CARTESIAN_POINT('Ctrl Pts',(-1.05760163192479,-1.,1.7150865442702));
#43279=CARTESIAN_POINT('Ctrl Pts',(-1.05760163192479,1.,1.7150865442702));
#43280=CARTESIAN_POINT('Ctrl Pts',(-1.05277517202855,-1.,1.71139783543989));
#43281=CARTESIAN_POINT('Ctrl Pts',(-1.05277517202855,1.,1.71139783543989));
#43282=CARTESIAN_POINT('Ctrl Pts',(-1.04799085404995,-1.,1.70767646263649));
#43283=CARTESIAN_POINT('Ctrl Pts',(-1.04799085404995,1.,1.70767646263649));
#43284=CARTESIAN_POINT('Ctrl Pts',(-1.04324363334554,-1.,1.70391338707982));
#43285=CARTESIAN_POINT('Ctrl Pts',(-1.04324363334554,1.,1.70391338707982));
#43286=CARTESIAN_POINT('Ctrl Pts',(-1.03852922490789,-1.,1.70010052930962));
#43287=CARTESIAN_POINT('Ctrl Pts',(-1.03852922490789,1.,1.70010052930962));
#43288=CARTESIAN_POINT('Ctrl Pts',(-1.03384646003588,-1.,1.69623414782771));
#43289=CARTESIAN_POINT('Ctrl Pts',(-1.03384646003588,1.,1.69623414782771));
#43290=CARTESIAN_POINT('Ctrl Pts',(-1.02919977579147,-1.,1.69231840863458));
#43291=CARTESIAN_POINT('Ctrl Pts',(-1.02919977579147,1.,1.69231840863458));
#43292=CARTESIAN_POINT('Ctrl Pts',(-1.02460180535255,-1.,1.68836910178447));
#43293=CARTESIAN_POINT('Ctrl Pts',(-1.02460180535255,1.,1.68836910178447));
#43294=CARTESIAN_POINT('Ctrl Pts',(-1.02006795074201,-1.,1.68440578021706));
#43295=CARTESIAN_POINT('Ctrl Pts',(-1.02006795074201,1.,1.68440578021706));
#43296=CARTESIAN_POINT('Ctrl Pts',(-1.01561026162773,-1.,1.68044289894798));
#43297=CARTESIAN_POINT('Ctrl Pts',(-1.01561026162773,1.,1.68044289894798));
#43298=CARTESIAN_POINT('Ctrl Pts',(-1.01123236493511,-1.,1.67648246776464));
#43299=CARTESIAN_POINT('Ctrl Pts',(-1.01123236493511,1.,1.67648246776464));
#43300=CARTESIAN_POINT('Ctrl Pts',(-1.00692206696414,-1.,1.67250335383293));
#43301=CARTESIAN_POINT('Ctrl Pts',(-1.00692206696414,1.,1.67250335383293));
#43302=CARTESIAN_POINT('Ctrl Pts',(-1.00265091003727,-1.,1.66846059277303));
#43303=CARTESIAN_POINT('Ctrl Pts',(-1.00265091003727,1.,1.66846059277303));
#43304=CARTESIAN_POINT('Ctrl Pts',(-0.998389654952758,-1.,1.66430758030376));
#43305=CARTESIAN_POINT('Ctrl Pts',(-0.998389654952758,1.,1.66430758030376));
#43306=CARTESIAN_POINT('Ctrl Pts',(-0.994121836661306,-1.,1.66001553809947));
#43307=CARTESIAN_POINT('Ctrl Pts',(-0.994121836661306,1.,1.66001553809947));
#43308=CARTESIAN_POINT('Ctrl Pts',(-0.989855627854165,-1.,1.65559044289699));
#43309=CARTESIAN_POINT('Ctrl Pts',(-0.989855627854165,1.,1.65559044289699));
#43310=CARTESIAN_POINT('Ctrl Pts',(-0.985642622920821,-1.,1.65110016612638));
#43311=CARTESIAN_POINT('Ctrl Pts',(-0.985642622920821,1.,1.65110016612638));
#43312=CARTESIAN_POINT('Ctrl Pts',(-0.981562530939489,-1.,1.64665139190656));
#43313=CARTESIAN_POINT('Ctrl Pts',(-0.981562530939489,1.,1.64665139190656));
#43314=CARTESIAN_POINT('Ctrl Pts',(-0.977689794119416,-1.,1.64233990826687));
#43315=CARTESIAN_POINT('Ctrl Pts',(-0.977689794119416,1.,1.64233990826687));
#43316=CARTESIAN_POINT('Ctrl Pts',(-0.974066058287418,-1.,1.63820952658144));
#43317=CARTESIAN_POINT('Ctrl Pts',(-0.974066058287418,1.,1.63820952658144));
#43318=CARTESIAN_POINT('Ctrl Pts',(-0.970669715997509,-1.,1.63420665729798));
#43319=CARTESIAN_POINT('Ctrl Pts',(-0.970669715997509,1.,1.63420665729798));
#43320=CARTESIAN_POINT('Ctrl Pts',(-0.967387853230345,-1.,1.63013849959461));
#43321=CARTESIAN_POINT('Ctrl Pts',(-0.967387853230345,1.,1.63013849959461));
#43322=CARTESIAN_POINT('Ctrl Pts',(-0.964046107040536,-1.,1.62571930670187));
#43323=CARTESIAN_POINT('Ctrl Pts',(-0.964046107040536,1.,1.62571930670187));
#43324=CARTESIAN_POINT('Ctrl Pts',(-0.960438326101729,-1.,1.62061638140221));
#43325=CARTESIAN_POINT('Ctrl Pts',(-0.960438326101729,1.,1.62061638140221));
#43326=CARTESIAN_POINT('Ctrl Pts',(-0.956354422920671,-1.,1.61449324337085));
#43327=CARTESIAN_POINT('Ctrl Pts',(-0.956354422920671,1.,1.61449324337085));
#43328=CARTESIAN_POINT('Ctrl Pts',(-0.951613284356035,-1.,1.60706069896936));
#43329=CARTESIAN_POINT('Ctrl Pts',(-0.951613284356035,1.,1.60706069896936));
#43330=CARTESIAN_POINT('Ctrl Pts',(-0.946078063315257,-1.,1.59810042043673));
#43331=CARTESIAN_POINT('Ctrl Pts',(-0.946078063315257,1.,1.59810042043673));
#43332=CARTESIAN_POINT('Ctrl Pts',(-0.939646377893399,-1.,1.58744937487176));
#43333=CARTESIAN_POINT('Ctrl Pts',(-0.939646377893399,1.,1.58744937487176));
#43334=CARTESIAN_POINT('Ctrl Pts',(-0.932246680108685,-1.,1.57499388382243));
#43335=CARTESIAN_POINT('Ctrl Pts',(-0.932246680108685,1.,1.57499388382243));
#43336=CARTESIAN_POINT('Ctrl Pts',(-0.923832188944341,-1.,1.56065988578893));
#43337=CARTESIAN_POINT('Ctrl Pts',(-0.923832188944341,1.,1.56065988578893));
#43338=CARTESIAN_POINT('Ctrl Pts',(-0.914375919026456,-1.,1.54440491149498));
#43339=CARTESIAN_POINT('Ctrl Pts',(-0.914375919026456,1.,1.54440491149498));
#43340=CARTESIAN_POINT('Ctrl Pts',(-0.905967409625651,-1.,1.52984849887993));
#43341=CARTESIAN_POINT('Ctrl Pts',(-0.905967409625651,1.,1.52984849887993));
#43342=CARTESIAN_POINT('Ctrl Pts',(-0.899185047483511,-1.,1.51805569590094));
#43343=CARTESIAN_POINT('Ctrl Pts',(-0.899185047483511,1.,1.51805569590094));
#43344=CARTESIAN_POINT('Ctrl Pts',(-0.894452006964543,-1.,1.50980486806688));
#43345=CARTESIAN_POINT('Ctrl Pts',(-0.894452006964543,1.,1.50980486806688));
#43346=CARTESIAN_POINT('Ctrl Pts',(-0.892032620296855,-1.,1.5055822144029));
#43347=CARTESIAN_POINT('Ctrl Pts',(-0.892032620296855,1.,1.5055822144029));
#43348=CARTESIAN_POINT('',(-1.23627494547115,1.,1.81978687191668));
#43349=CARTESIAN_POINT('Ctrl Pts',(-1.23627494547115,1.,1.81978687191668));
#43350=CARTESIAN_POINT('Ctrl Pts',(-1.23509651170476,1.,1.81925017193666));
#43351=CARTESIAN_POINT('Ctrl Pts',(-1.2327422452705,1.,1.81817389921279));
#43352=CARTESIAN_POINT('Ctrl Pts',(-1.2292186489137,1.,1.8165508718364));
#43353=CARTESIAN_POINT('Ctrl Pts',(-1.2245361330495,1.,1.81436959210434));
#43354=CARTESIAN_POINT('Ctrl Pts',(-1.21870906103557,1.,1.81161420806656));
#43355=CARTESIAN_POINT('Ctrl Pts',(-1.21290815708314,1.,1.80882996917129));
#43356=CARTESIAN_POINT('Ctrl Pts',(-1.20713356605475,1.,1.80601678480707));
#43357=CARTESIAN_POINT('Ctrl Pts',(-1.20138548938974,1.,1.80317454838603));
#43358=CARTESIAN_POINT('Ctrl Pts',(-1.19566418930242,1.,1.80030314369879));
#43359=CARTESIAN_POINT('Ctrl Pts',(-1.18996997934445,1.,1.79740245923478));
#43360=CARTESIAN_POINT('Ctrl Pts',(-1.18430321697432,1.,1.79447240321515));
#43361=CARTESIAN_POINT('Ctrl Pts',(-1.17866429440809,1.,1.79151291552689));
#43362=CARTESIAN_POINT('Ctrl Pts',(-1.17305363177328,1.,1.78852398877616));
#43363=CARTESIAN_POINT('Ctrl Pts',(-1.16747166312303,1.,1.78550566040443));
#43364=CARTESIAN_POINT('Ctrl Pts',(-1.16191881298499,1.,1.78245795881009));
#43365=CARTESIAN_POINT('Ctrl Pts',(-1.15639547194698,1.,1.77938085564275));
#43366=CARTESIAN_POINT('Ctrl Pts',(-1.15090197841515,1.,1.7762742255701));
#43367=CARTESIAN_POINT('Ctrl Pts',(-1.1454385822692,1.,1.77313777896194));
#43368=CARTESIAN_POINT('Ctrl Pts',(-1.14000548336975,1.,1.76997111386769));
#43369=CARTESIAN_POINT('Ctrl Pts',(-1.1346029180462,1.,1.76677384551862));
#43370=CARTESIAN_POINT('Ctrl Pts',(-1.12923123555075,1.,1.7635457196617));
#43371=CARTESIAN_POINT('Ctrl Pts',(-1.12389096855086,1.,1.76028671825096));
#43372=CARTESIAN_POINT('Ctrl Pts',(-1.11858293216763,1.,1.75699720772105));
#43373=CARTESIAN_POINT('Ctrl Pts',(-1.11330807582551,1.,1.7536777209463));
#43374=CARTESIAN_POINT('Ctrl Pts',(-1.10806728183007,1.,1.7503286607592));
#43375=CARTESIAN_POINT('Ctrl Pts',(-1.10286118991143,1.,1.74695004214923));
#43376=CARTESIAN_POINT('Ctrl Pts',(-1.09768999241225,1.,1.74354119236208));
#43377=CARTESIAN_POINT('Ctrl Pts',(-1.09255329056493,1.,1.74010053962247));
#43378=CARTESIAN_POINT('Ctrl Pts',(-1.08745056285427,1.,1.73662628326091));
#43379=CARTESIAN_POINT('Ctrl Pts',(-1.08238162784749,1.,1.73311705663407));
#43380=CARTESIAN_POINT('Ctrl Pts',(-1.0773470373727,1.,1.72957248977424));
#43381=CARTESIAN_POINT('Ctrl Pts',(-1.07234866990252,1.,1.72599406198488));
#43382=CARTESIAN_POINT('Ctrl Pts',(-1.06738966975462,1.,1.72238500928453));
#43383=CARTESIAN_POINT('Ctrl Pts',(-1.06247324680647,1.,1.71874858456904));
#43384=CARTESIAN_POINT('Ctrl Pts',(-1.05760163192479,1.,1.7150865442702));
#43385=CARTESIAN_POINT('Ctrl Pts',(-1.05277517202855,1.,1.71139783543989));
#43386=CARTESIAN_POINT('Ctrl Pts',(-1.04799085404995,1.,1.70767646263649));
#43387=CARTESIAN_POINT('Ctrl Pts',(-1.04324363334554,1.,1.70391338707982));
#43388=CARTESIAN_POINT('Ctrl Pts',(-1.03852922490789,1.,1.70010052930962));
#43389=CARTESIAN_POINT('Ctrl Pts',(-1.03384646003588,1.,1.69623414782771));
#43390=CARTESIAN_POINT('Ctrl Pts',(-1.02919977579147,1.,1.69231840863458));
#43391=CARTESIAN_POINT('Ctrl Pts',(-1.02460180535255,1.,1.68836910178447));
#43392=CARTESIAN_POINT('Ctrl Pts',(-1.02006795074201,1.,1.68440578021706));
#43393=CARTESIAN_POINT('Ctrl Pts',(-1.01561026162773,1.,1.68044289894798));
#43394=CARTESIAN_POINT('Ctrl Pts',(-1.01123236493511,1.,1.67648246776464));
#43395=CARTESIAN_POINT('Ctrl Pts',(-1.00692206696414,1.,1.67250335383293));
#43396=CARTESIAN_POINT('Ctrl Pts',(-1.00265091003727,1.,1.66846059277303));
#43397=CARTESIAN_POINT('Ctrl Pts',(-0.998389654952758,1.,1.66430758030376));
#43398=CARTESIAN_POINT('Ctrl Pts',(-0.994121836661306,1.,1.66001553809947));
#43399=CARTESIAN_POINT('Ctrl Pts',(-0.989855627854165,1.,1.65559044289699));
#43400=CARTESIAN_POINT('Ctrl Pts',(-0.985642622920821,1.,1.65110016612638));
#43401=CARTESIAN_POINT('Ctrl Pts',(-0.981562530939489,1.,1.64665139190656));
#43402=CARTESIAN_POINT('Ctrl Pts',(-0.977689794119416,1.,1.64233990826687));
#43403=CARTESIAN_POINT('Ctrl Pts',(-0.974066058287418,1.,1.63820952658144));
#43404=CARTESIAN_POINT('Ctrl Pts',(-0.970669715997509,1.,1.63420665729798));
#43405=CARTESIAN_POINT('Ctrl Pts',(-0.967387853230345,1.,1.63013849959461));
#43406=CARTESIAN_POINT('Ctrl Pts',(-0.964046107040536,1.,1.62571930670187));
#43407=CARTESIAN_POINT('Ctrl Pts',(-0.960438326101729,1.,1.62061638140221));
#43408=CARTESIAN_POINT('Ctrl Pts',(-0.956354422920671,1.,1.61449324337085));
#43409=CARTESIAN_POINT('Ctrl Pts',(-0.951613284356035,1.,1.60706069896936));
#43410=CARTESIAN_POINT('Ctrl Pts',(-0.946078063315257,1.,1.59810042043673));
#43411=CARTESIAN_POINT('Ctrl Pts',(-0.939646377893399,1.,1.58744937487176));
#43412=CARTESIAN_POINT('Ctrl Pts',(-0.932246680108685,1.,1.57499388382243));
#43413=CARTESIAN_POINT('Ctrl Pts',(-0.923832188944341,1.,1.56065988578893));
#43414=CARTESIAN_POINT('Ctrl Pts',(-0.914375919026456,1.,1.54440491149498));
#43415=CARTESIAN_POINT('Ctrl Pts',(-0.905967409625651,1.,1.52984849887993));
#43416=CARTESIAN_POINT('Ctrl Pts',(-0.899185047483511,1.,1.51805569590094));
#43417=CARTESIAN_POINT('Ctrl Pts',(-0.894452006964543,1.,1.50980486806688));
#43418=CARTESIAN_POINT('Ctrl Pts',(-0.892032620296855,1.,1.5055822144029));
#43419=CARTESIAN_POINT('',(-1.23627494547115,0.,1.81978687191668));
#43420=CARTESIAN_POINT('Origin',(-1.34869019493419,0.,1.73811241238545));
#43421=CARTESIAN_POINT('',(-1.34869019493419,1.,1.73811241238545));
#43422=CARTESIAN_POINT('',(-1.23627494547115,1.,1.81978687191668));
#43423=CARTESIAN_POINT('',(-1.34869019493419,0.,1.73811241238545));
#43424=CARTESIAN_POINT('Ctrl Pts',(-1.15624053661742,-1.,1.31362392696032));
#43425=CARTESIAN_POINT('Ctrl Pts',(-1.15624053661742,1.,1.31362392696032));
#43426=CARTESIAN_POINT('Ctrl Pts',(-1.15950888730809,-1.,1.31722977216397));
#43427=CARTESIAN_POINT('Ctrl Pts',(-1.15950888730809,1.,1.31722977216397));
#43428=CARTESIAN_POINT('Ctrl Pts',(-1.16589330093588,-1.,1.32428080721772));
#43429=CARTESIAN_POINT('Ctrl Pts',(-1.16589330093588,1.,1.32428080721772));
#43430=CARTESIAN_POINT('Ctrl Pts',(-1.17501305789857,-1.,1.33437539347008));
#43431=CARTESIAN_POINT('Ctrl Pts',(-1.17501305789857,1.,1.33437539347008));
#43432=CARTESIAN_POINT('Ctrl Pts',(-1.18625865667441,-1.,1.34687054001093));
#43433=CARTESIAN_POINT('Ctrl Pts',(-1.18625865667441,1.,1.34687054001093));
#43434=CARTESIAN_POINT('Ctrl Pts',(-1.1987959077932,-1.,1.36088705043885));
#43435=CARTESIAN_POINT('Ctrl Pts',(-1.1987959077932,1.,1.36088705043885));
#43436=CARTESIAN_POINT('Ctrl Pts',(-1.20982812925645,-1.,1.37331915607905));
#43437=CARTESIAN_POINT('Ctrl Pts',(-1.20982812925645,1.,1.37331915607905));
#43438=CARTESIAN_POINT('Ctrl Pts',(-1.21938737280852,-1.,1.38420564527715));
#43439=CARTESIAN_POINT('Ctrl Pts',(-1.21938737280852,1.,1.38420564527715));
#43440=CARTESIAN_POINT('Ctrl Pts',(-1.22752961899387,-1.,1.39361389568796));
#43441=CARTESIAN_POINT('Ctrl Pts',(-1.22752961899387,1.,1.39361389568796));
#43442=CARTESIAN_POINT('Ctrl Pts',(-1.23434087290423,-1.,1.40164708206106));
#43443=CARTESIAN_POINT('Ctrl Pts',(-1.23434087290423,1.,1.40164708206106));
#43444=CARTESIAN_POINT('Ctrl Pts',(-1.23994455029534,-1.,1.40845295531283));
#43445=CARTESIAN_POINT('Ctrl Pts',(-1.23994455029534,1.,1.40845295531283));
#43446=CARTESIAN_POINT('Ctrl Pts',(-1.24450600513056,-1.,1.41422913175179));
#43447=CARTESIAN_POINT('Ctrl Pts',(-1.24450600513056,1.,1.41422913175179));
#43448=CARTESIAN_POINT('Ctrl Pts',(-1.24824430986571,-1.,1.41923722596025));
#43449=CARTESIAN_POINT('Ctrl Pts',(-1.24824430986571,1.,1.41923722596025));
#43450=CARTESIAN_POINT('Ctrl Pts',(-1.2514145557001,-1.,1.42378102115575));
#43451=CARTESIAN_POINT('Ctrl Pts',(-1.2514145557001,1.,1.42378102115575));
#43452=CARTESIAN_POINT('Ctrl Pts',(-1.25426945222639,-1.,1.42815938799387));
#43453=CARTESIAN_POINT('Ctrl Pts',(-1.25426945222639,1.,1.42815938799387));
#43454=CARTESIAN_POINT('Ctrl Pts',(-1.25702687965755,-1.,1.43262645609691));
#43455=CARTESIAN_POINT('Ctrl Pts',(-1.25702687965755,1.,1.43262645609691));
#43456=CARTESIAN_POINT('Ctrl Pts',(-1.25983531012005,-1.,1.43734919180848));
#43457=CARTESIAN_POINT('Ctrl Pts',(-1.25983531012005,1.,1.43734919180848));
#43458=CARTESIAN_POINT('Ctrl Pts',(-1.26273903323859,-1.,1.44236470511303));
#43459=CARTESIAN_POINT('Ctrl Pts',(-1.26273903323859,1.,1.44236470511303));
#43460=CARTESIAN_POINT('Ctrl Pts',(-1.26570925118868,-1.,1.44761985001662));
#43461=CARTESIAN_POINT('Ctrl Pts',(-1.26570925118868,1.,1.44761985001662));
#43462=CARTESIAN_POINT('Ctrl Pts',(-1.2686778680489,-1.,1.45301422764247));
#43463=CARTESIAN_POINT('Ctrl Pts',(-1.2686778680489,1.,1.45301422764247));
#43464=CARTESIAN_POINT('Ctrl Pts',(-1.27156805265289,-1.,1.45843906294697));
#43465=CARTESIAN_POINT('Ctrl Pts',(-1.27156805265289,1.,1.45843906294697));
#43466=CARTESIAN_POINT('Ctrl Pts',(-1.27433119897822,-1.,1.46382431332476));
#43467=CARTESIAN_POINT('Ctrl Pts',(-1.27433119897822,1.,1.46382431332476));
#43468=CARTESIAN_POINT('Ctrl Pts',(-1.27696414831089,-1.,1.46916035917133));
#43469=CARTESIAN_POINT('Ctrl Pts',(-1.27696414831089,1.,1.46916035917133));
#43470=CARTESIAN_POINT('Ctrl Pts',(-1.2794891824849,-1.,1.4744717526707));
#43471=CARTESIAN_POINT('Ctrl Pts',(-1.2794891824849,1.,1.4744717526707));
#43472=CARTESIAN_POINT('Ctrl Pts',(-1.28194158939517,-1.,1.47980070347095));
#43473=CARTESIAN_POINT('Ctrl Pts',(-1.28194158939517,1.,1.47980070347095));
#43474=CARTESIAN_POINT('Ctrl Pts',(-1.28435533880201,-1.,1.4851881711891));
#43475=CARTESIAN_POINT('Ctrl Pts',(-1.28435533880201,1.,1.4851881711891));
#43476=CARTESIAN_POINT('Ctrl Pts',(-1.2867467611644,-1.,1.4906522831278));
#43477=CARTESIAN_POINT('Ctrl Pts',(-1.2867467611644,1.,1.4906522831278));
#43478=CARTESIAN_POINT('Ctrl Pts',(-1.28911506584254,-1.,1.49618896881754));
#43479=CARTESIAN_POINT('Ctrl Pts',(-1.28911506584254,1.,1.49618896881754));
#43480=CARTESIAN_POINT('Ctrl Pts',(-1.29145022885181,-1.,1.50178230149776));
#43481=CARTESIAN_POINT('Ctrl Pts',(-1.29145022885181,1.,1.50178230149776));
#43482=CARTESIAN_POINT('Ctrl Pts',(-1.29373841372842,-1.,1.50741159078365));
#43483=CARTESIAN_POINT('Ctrl Pts',(-1.29373841372842,1.,1.50741159078365));
#43484=CARTESIAN_POINT('Ctrl Pts',(-1.29596850710509,-1.,1.51305994241402));
#43485=CARTESIAN_POINT('Ctrl Pts',(-1.29596850710509,1.,1.51305994241402));
#43486=CARTESIAN_POINT('Ctrl Pts',(-1.29813791800747,-1.,1.51872184912724));
#43487=CARTESIAN_POINT('Ctrl Pts',(-1.29813791800747,1.,1.51872184912724));
#43488=CARTESIAN_POINT('Ctrl Pts',(-1.30024984366328,-1.,1.52439957861062));
#43489=CARTESIAN_POINT('Ctrl Pts',(-1.30024984366328,1.,1.52439957861062));
#43490=CARTESIAN_POINT('Ctrl Pts',(-1.30231064395568,-1.,1.53009970283891));
#43491=CARTESIAN_POINT('Ctrl Pts',(-1.30231064395568,1.,1.53009970283891));
#43492=CARTESIAN_POINT('Ctrl Pts',(-1.30432735639489,-1.,1.53582981268977));
#43493=CARTESIAN_POINT('Ctrl Pts',(-1.30432735639489,1.,1.53582981268977));
#43494=CARTESIAN_POINT('Ctrl Pts',(-1.30630475189556,-1.,1.54159462645432));
#43495=CARTESIAN_POINT('Ctrl Pts',(-1.30630475189556,1.,1.54159462645432));
#43496=CARTESIAN_POINT('Ctrl Pts',(-1.30824393907473,-1.,1.54739413957185));
#43497=CARTESIAN_POINT('Ctrl Pts',(-1.30824393907473,1.,1.54739413957185));
#43498=CARTESIAN_POINT('Ctrl Pts',(-1.31014393684222,-1.,1.55322568759481));
#43499=CARTESIAN_POINT('Ctrl Pts',(-1.31014393684222,1.,1.55322568759481));
#43500=CARTESIAN_POINT('Ctrl Pts',(-1.31200264341696,-1.,1.55908521254821));
#43501=CARTESIAN_POINT('Ctrl Pts',(-1.31200264341696,1.,1.55908521254821));
#43502=CARTESIAN_POINT('Ctrl Pts',(-1.31381795281002,-1.,1.56496872402353));
#43503=CARTESIAN_POINT('Ctrl Pts',(-1.31381795281002,1.,1.56496872402353));
#43504=CARTESIAN_POINT('Ctrl Pts',(-1.31558903860016,-1.,1.57087397835723));
#43505=CARTESIAN_POINT('Ctrl Pts',(-1.31558903860016,1.,1.57087397835723));
#43506=CARTESIAN_POINT('Ctrl Pts',(-1.31731642317187,-1.,1.5768005650559));
#43507=CARTESIAN_POINT('Ctrl Pts',(-1.31731642317187,1.,1.5768005650559));
#43508=CARTESIAN_POINT('Ctrl Pts',(-1.31900135021432,-1.,1.58274907898834));
#43509=CARTESIAN_POINT('Ctrl Pts',(-1.31900135021432,1.,1.58274907898834));
#43510=CARTESIAN_POINT('Ctrl Pts',(-1.32064537110892,-1.,1.58872057258245));
#43511=CARTESIAN_POINT('Ctrl Pts',(-1.32064537110892,1.,1.58872057258245));
#43512=CARTESIAN_POINT('Ctrl Pts',(-1.32224985747682,-1.,1.59471591079403));
#43513=CARTESIAN_POINT('Ctrl Pts',(-1.32224985747682,1.,1.59471591079403));
#43514=CARTESIAN_POINT('Ctrl Pts',(-1.32381550858256,-1.,1.60073511858687));
#43515=CARTESIAN_POINT('Ctrl Pts',(-1.32381550858256,1.,1.60073511858687));
#43516=CARTESIAN_POINT('Ctrl Pts',(-1.32534250785782,-1.,1.60677758290954));
#43517=CARTESIAN_POINT('Ctrl Pts',(-1.32534250785782,1.,1.60677758290954));
#43518=CARTESIAN_POINT('Ctrl Pts',(-1.32683074483356,-1.,1.6128423401575));
#43519=CARTESIAN_POINT('Ctrl Pts',(-1.32683074483356,1.,1.6128423401575));
#43520=CARTESIAN_POINT('Ctrl Pts',(-1.32828000610449,-1.,1.61892832270724));
#43521=CARTESIAN_POINT('Ctrl Pts',(-1.32828000610449,1.,1.61892832270724));
#43522=CARTESIAN_POINT('Ctrl Pts',(-1.3296901950568,-1.,1.62503464209797));
#43523=CARTESIAN_POINT('Ctrl Pts',(-1.3296901950568,1.,1.62503464209797));
#43524=CARTESIAN_POINT('Ctrl Pts',(-1.33106149345645,-1.,1.63116079730923));
#43525=CARTESIAN_POINT('Ctrl Pts',(-1.33106149345645,1.,1.63116079730923));
#43526=CARTESIAN_POINT('Ctrl Pts',(-1.33239425103724,-1.,1.63730653475089));
#43527=CARTESIAN_POINT('Ctrl Pts',(-1.33239425103724,1.,1.63730653475089));
#43528=CARTESIAN_POINT('Ctrl Pts',(-1.33368890676572,-1.,1.6434717485603));
#43529=CARTESIAN_POINT('Ctrl Pts',(-1.33368890676572,1.,1.6434717485603));
#43530=CARTESIAN_POINT('Ctrl Pts',(-1.33494590467993,-1.,1.6496563728683));
#43531=CARTESIAN_POINT('Ctrl Pts',(-1.33494590467993,1.,1.6496563728683));
#43532=CARTESIAN_POINT('Ctrl Pts',(-1.33616559745172,-1.,1.65586025952593));
#43533=CARTESIAN_POINT('Ctrl Pts',(-1.33616559745172,1.,1.65586025952593));
#43534=CARTESIAN_POINT('Ctrl Pts',(-1.33734820885262,-1.,1.66208312541983));
#43535=CARTESIAN_POINT('Ctrl Pts',(-1.33734820885262,1.,1.66208312541983));
#43536=CARTESIAN_POINT('Ctrl Pts',(-1.33849388654388,-1.,1.66832460783989));
#43537=CARTESIAN_POINT('Ctrl Pts',(-1.33849388654388,1.,1.66832460783989));
#43538=CARTESIAN_POINT('Ctrl Pts',(-1.3396027347034,-1.,1.67458429426086));
#43539=CARTESIAN_POINT('Ctrl Pts',(-1.3396027347034,1.,1.67458429426086));
#43540=CARTESIAN_POINT('Ctrl Pts',(-1.34067485185203,-1.,1.68086176030362));
#43541=CARTESIAN_POINT('Ctrl Pts',(-1.34067485185203,1.,1.68086176030362));
#43542=CARTESIAN_POINT('Ctrl Pts',(-1.341710374848,-1.,1.68715660868764));
#43543=CARTESIAN_POINT('Ctrl Pts',(-1.341710374848,1.,1.68715660868764));
#43544=CARTESIAN_POINT('Ctrl Pts',(-1.34270948206319,-1.,1.6934684849687));
#43545=CARTESIAN_POINT('Ctrl Pts',(-1.34270948206319,1.,1.6934684849687));
#43546=CARTESIAN_POINT('Ctrl Pts',(-1.34367237124483,-1.,1.69979707754427));
#43547=CARTESIAN_POINT('Ctrl Pts',(-1.34367237124483,1.,1.69979707754427));
#43548=CARTESIAN_POINT('Ctrl Pts',(-1.34459924533831,-1.,1.70614212266738));
#43549=CARTESIAN_POINT('Ctrl Pts',(-1.34459924533831,1.,1.70614212266738));
#43550=CARTESIAN_POINT('Ctrl Pts',(-1.34549029589416,-1.,1.71250340686822));
#43551=CARTESIAN_POINT('Ctrl Pts',(-1.34549029589416,1.,1.71250340686822));
#43552=CARTESIAN_POINT('Ctrl Pts',(-1.34634568653227,-1.,1.7188807715049));
#43553=CARTESIAN_POINT('Ctrl Pts',(-1.34634568653227,1.,1.7188807715049));
#43554=CARTESIAN_POINT('Ctrl Pts',(-1.34716554819527,-1.,1.72527410680674));
#43555=CARTESIAN_POINT('Ctrl Pts',(-1.34716554819527,1.,1.72527410680674));
#43556=CARTESIAN_POINT('Ctrl Pts',(-1.34779309152035,-1.,1.7304014965394));
#43557=CARTESIAN_POINT('Ctrl Pts',(-1.34779309152035,1.,1.7304014965394));
#43558=CARTESIAN_POINT('Ctrl Pts',(-1.34824783112887,-1.,1.73425417885907));
#43559=CARTESIAN_POINT('Ctrl Pts',(-1.34824783112887,1.,1.73425417885907));
#43560=CARTESIAN_POINT('Ctrl Pts',(-1.34854391898045,-1.,1.73682580585691));
#43561=CARTESIAN_POINT('Ctrl Pts',(-1.34854391898045,1.,1.73682580585691));
#43562=CARTESIAN_POINT('Ctrl Pts',(-1.34869019493419,-1.,1.73811241238545));
#43563=CARTESIAN_POINT('Ctrl Pts',(-1.34869019493419,1.,1.73811241238545));
#43564=CARTESIAN_POINT('',(-1.15624053661742,1.,1.31362392696032));
#43565=CARTESIAN_POINT('Ctrl Pts',(-1.15624053661742,1.,1.31362392696032));
#43566=CARTESIAN_POINT('Ctrl Pts',(-1.15950888730809,1.,1.31722977216397));
#43567=CARTESIAN_POINT('Ctrl Pts',(-1.16589330093588,1.,1.32428080721772));
#43568=CARTESIAN_POINT('Ctrl Pts',(-1.17501305789857,1.,1.33437539347008));
#43569=CARTESIAN_POINT('Ctrl Pts',(-1.18625865667441,1.,1.34687054001093));
#43570=CARTESIAN_POINT('Ctrl Pts',(-1.1987959077932,1.,1.36088705043885));
#43571=CARTESIAN_POINT('Ctrl Pts',(-1.20982812925645,1.,1.37331915607905));
#43572=CARTESIAN_POINT('Ctrl Pts',(-1.21938737280852,1.,1.38420564527715));
#43573=CARTESIAN_POINT('Ctrl Pts',(-1.22752961899387,1.,1.39361389568796));
#43574=CARTESIAN_POINT('Ctrl Pts',(-1.23434087290423,1.,1.40164708206106));
#43575=CARTESIAN_POINT('Ctrl Pts',(-1.23994455029534,1.,1.40845295531283));
#43576=CARTESIAN_POINT('Ctrl Pts',(-1.24450600513056,1.,1.41422913175179));
#43577=CARTESIAN_POINT('Ctrl Pts',(-1.24824430986571,1.,1.41923722596025));
#43578=CARTESIAN_POINT('Ctrl Pts',(-1.2514145557001,1.,1.42378102115575));
#43579=CARTESIAN_POINT('Ctrl Pts',(-1.25426945222639,1.,1.42815938799387));
#43580=CARTESIAN_POINT('Ctrl Pts',(-1.25702687965755,1.,1.43262645609691));
#43581=CARTESIAN_POINT('Ctrl Pts',(-1.25983531012005,1.,1.43734919180848));
#43582=CARTESIAN_POINT('Ctrl Pts',(-1.26273903323859,1.,1.44236470511303));
#43583=CARTESIAN_POINT('Ctrl Pts',(-1.26570925118868,1.,1.44761985001662));
#43584=CARTESIAN_POINT('Ctrl Pts',(-1.2686778680489,1.,1.45301422764247));
#43585=CARTESIAN_POINT('Ctrl Pts',(-1.27156805265289,1.,1.45843906294697));
#43586=CARTESIAN_POINT('Ctrl Pts',(-1.27433119897822,1.,1.46382431332476));
#43587=CARTESIAN_POINT('Ctrl Pts',(-1.27696414831089,1.,1.46916035917133));
#43588=CARTESIAN_POINT('Ctrl Pts',(-1.2794891824849,1.,1.4744717526707));
#43589=CARTESIAN_POINT('Ctrl Pts',(-1.28194158939517,1.,1.47980070347095));
#43590=CARTESIAN_POINT('Ctrl Pts',(-1.28435533880201,1.,1.4851881711891));
#43591=CARTESIAN_POINT('Ctrl Pts',(-1.2867467611644,1.,1.4906522831278));
#43592=CARTESIAN_POINT('Ctrl Pts',(-1.28911506584254,1.,1.49618896881754));
#43593=CARTESIAN_POINT('Ctrl Pts',(-1.29145022885181,1.,1.50178230149776));
#43594=CARTESIAN_POINT('Ctrl Pts',(-1.29373841372842,1.,1.50741159078365));
#43595=CARTESIAN_POINT('Ctrl Pts',(-1.29596850710509,1.,1.51305994241402));
#43596=CARTESIAN_POINT('Ctrl Pts',(-1.29813791800747,1.,1.51872184912724));
#43597=CARTESIAN_POINT('Ctrl Pts',(-1.30024984366328,1.,1.52439957861062));
#43598=CARTESIAN_POINT('Ctrl Pts',(-1.30231064395568,1.,1.53009970283891));
#43599=CARTESIAN_POINT('Ctrl Pts',(-1.30432735639489,1.,1.53582981268977));
#43600=CARTESIAN_POINT('Ctrl Pts',(-1.30630475189556,1.,1.54159462645432));
#43601=CARTESIAN_POINT('Ctrl Pts',(-1.30824393907473,1.,1.54739413957185));
#43602=CARTESIAN_POINT('Ctrl Pts',(-1.31014393684222,1.,1.55322568759481));
#43603=CARTESIAN_POINT('Ctrl Pts',(-1.31200264341696,1.,1.55908521254821));
#43604=CARTESIAN_POINT('Ctrl Pts',(-1.31381795281002,1.,1.56496872402353));
#43605=CARTESIAN_POINT('Ctrl Pts',(-1.31558903860016,1.,1.57087397835723));
#43606=CARTESIAN_POINT('Ctrl Pts',(-1.31731642317187,1.,1.5768005650559));
#43607=CARTESIAN_POINT('Ctrl Pts',(-1.31900135021432,1.,1.58274907898834));
#43608=CARTESIAN_POINT('Ctrl Pts',(-1.32064537110892,1.,1.58872057258245));
#43609=CARTESIAN_POINT('Ctrl Pts',(-1.32224985747682,1.,1.59471591079403));
#43610=CARTESIAN_POINT('Ctrl Pts',(-1.32381550858256,1.,1.60073511858687));
#43611=CARTESIAN_POINT('Ctrl Pts',(-1.32534250785782,1.,1.60677758290954));
#43612=CARTESIAN_POINT('Ctrl Pts',(-1.32683074483356,1.,1.6128423401575));
#43613=CARTESIAN_POINT('Ctrl Pts',(-1.32828000610449,1.,1.61892832270724));
#43614=CARTESIAN_POINT('Ctrl Pts',(-1.3296901950568,1.,1.62503464209797));
#43615=CARTESIAN_POINT('Ctrl Pts',(-1.33106149345645,1.,1.63116079730923));
#43616=CARTESIAN_POINT('Ctrl Pts',(-1.33239425103724,1.,1.63730653475089));
#43617=CARTESIAN_POINT('Ctrl Pts',(-1.33368890676572,1.,1.6434717485603));
#43618=CARTESIAN_POINT('Ctrl Pts',(-1.33494590467993,1.,1.6496563728683));
#43619=CARTESIAN_POINT('Ctrl Pts',(-1.33616559745172,1.,1.65586025952593));
#43620=CARTESIAN_POINT('Ctrl Pts',(-1.33734820885262,1.,1.66208312541983));
#43621=CARTESIAN_POINT('Ctrl Pts',(-1.33849388654388,1.,1.66832460783989));
#43622=CARTESIAN_POINT('Ctrl Pts',(-1.3396027347034,1.,1.67458429426086));
#43623=CARTESIAN_POINT('Ctrl Pts',(-1.34067485185203,1.,1.68086176030362));
#43624=CARTESIAN_POINT('Ctrl Pts',(-1.341710374848,1.,1.68715660868764));
#43625=CARTESIAN_POINT('Ctrl Pts',(-1.34270948206319,1.,1.6934684849687));
#43626=CARTESIAN_POINT('Ctrl Pts',(-1.34367237124483,1.,1.69979707754427));
#43627=CARTESIAN_POINT('Ctrl Pts',(-1.34459924533831,1.,1.70614212266738));
#43628=CARTESIAN_POINT('Ctrl Pts',(-1.34549029589416,1.,1.71250340686822));
#43629=CARTESIAN_POINT('Ctrl Pts',(-1.34634568653227,1.,1.7188807715049));
#43630=CARTESIAN_POINT('Ctrl Pts',(-1.34716554819527,1.,1.72527410680674));
#43631=CARTESIAN_POINT('Ctrl Pts',(-1.34779309152035,1.,1.7304014965394));
#43632=CARTESIAN_POINT('Ctrl Pts',(-1.34824783112887,1.,1.73425417885907));
#43633=CARTESIAN_POINT('Ctrl Pts',(-1.34854391898045,1.,1.73682580585691));
#43634=CARTESIAN_POINT('Ctrl Pts',(-1.34869019493419,1.,1.73811241238545));
#43635=CARTESIAN_POINT('',(-1.15624053661742,0.,1.31362392696032));
#43636=CARTESIAN_POINT('Origin',(0.,0.,0.));
#43637=CARTESIAN_POINT('',(-1.31362392696033,1.,1.15624053661742));
#43638=CARTESIAN_POINT('Origin',(0.,1.,0.));
#43639=CARTESIAN_POINT('',(-1.31362392696033,0.,1.15624053661742));
#43640=CARTESIAN_POINT('Ctrl Pts',(-1.73811241238545,-1.,1.34869019493419));
#43641=CARTESIAN_POINT('Ctrl Pts',(-1.73811241238545,1.,1.34869019493419));
#43642=CARTESIAN_POINT('Ctrl Pts',(-1.73682580585819,-1.,1.34854391898145));
#43643=CARTESIAN_POINT('Ctrl Pts',(-1.73682580585819,1.,1.34854391898145));
#43644=CARTESIAN_POINT('Ctrl Pts',(-1.73425417886255,-1.,1.34824783113158));
#43645=CARTESIAN_POINT('Ctrl Pts',(-1.73425417886255,1.,1.34824783113158));
#43646=CARTESIAN_POINT('Ctrl Pts',(-1.73040149654497,-1.,1.3477930915247));
#43647=CARTESIAN_POINT('Ctrl Pts',(-1.73040149654497,1.,1.3477930915247));
#43648=CARTESIAN_POINT('Ctrl Pts',(-1.72527410681298,-1.,1.34716554820013));
#43649=CARTESIAN_POINT('Ctrl Pts',(-1.72527410681298,1.,1.34716554820013));
#43650=CARTESIAN_POINT('Ctrl Pts',(-1.7188807715095,-1.,1.34634568653586));
#43651=CARTESIAN_POINT('Ctrl Pts',(-1.7188807715095,1.,1.34634568653586));
#43652=CARTESIAN_POINT('Ctrl Pts',(-1.71250340687011,-1.,1.34549029589563));
#43653=CARTESIAN_POINT('Ctrl Pts',(-1.71250340687011,1.,1.34549029589563));
#43654=CARTESIAN_POINT('Ctrl Pts',(-1.70614212266676,-1.,1.34459924533783));
#43655=CARTESIAN_POINT('Ctrl Pts',(-1.70614212266676,1.,1.34459924533783));
#43656=CARTESIAN_POINT('Ctrl Pts',(-1.69979707754221,-1.,1.34367237124322));
#43657=CARTESIAN_POINT('Ctrl Pts',(-1.69979707754221,1.,1.34367237124322));
#43658=CARTESIAN_POINT('Ctrl Pts',(-1.6934684849664,-1.,1.34270948206139));
#43659=CARTESIAN_POINT('Ctrl Pts',(-1.6934684849664,1.,1.34270948206139));
#43660=CARTESIAN_POINT('Ctrl Pts',(-1.68715660868602,-1.,1.34171037484673));
#43661=CARTESIAN_POINT('Ctrl Pts',(-1.68715660868602,1.,1.34171037484673));
#43662=CARTESIAN_POINT('Ctrl Pts',(-1.68086176030308,-1.,1.3406748518516));
#43663=CARTESIAN_POINT('Ctrl Pts',(-1.68086176030308,1.,1.3406748518516));
#43664=CARTESIAN_POINT('Ctrl Pts',(-1.67458429426126,-1.,1.33960273470372));
#43665=CARTESIAN_POINT('Ctrl Pts',(-1.67458429426126,1.,1.33960273470372));
#43666=CARTESIAN_POINT('Ctrl Pts',(-1.66832460784078,-1.,1.33849388654458));
#43667=CARTESIAN_POINT('Ctrl Pts',(-1.66832460784078,1.,1.33849388654458));
#43668=CARTESIAN_POINT('Ctrl Pts',(-1.66208312542073,-1.,1.33734820885331));
#43669=CARTESIAN_POINT('Ctrl Pts',(-1.66208312542073,1.,1.33734820885331));
#43670=CARTESIAN_POINT('Ctrl Pts',(-1.65586025952651,-1.,1.33616559745217));
#43671=CARTESIAN_POINT('Ctrl Pts',(-1.65586025952651,1.,1.33616559745217));
#43672=CARTESIAN_POINT('Ctrl Pts',(-1.64965637286843,-1.,1.33494590468003));
#43673=CARTESIAN_POINT('Ctrl Pts',(-1.64965637286843,1.,1.33494590468003));
#43674=CARTESIAN_POINT('Ctrl Pts',(-1.64347174856007,-1.,1.33368890676554));
#43675=CARTESIAN_POINT('Ctrl Pts',(-1.64347174856007,1.,1.33368890676554));
#43676=CARTESIAN_POINT('Ctrl Pts',(-1.6373065347505,-1.,1.33239425103694));
#43677=CARTESIAN_POINT('Ctrl Pts',(-1.6373065347505,1.,1.33239425103694));
#43678=CARTESIAN_POINT('Ctrl Pts',(-1.63116079730887,-1.,1.33106149345618));
#43679=CARTESIAN_POINT('Ctrl Pts',(-1.63116079730887,1.,1.33106149345618));
#43680=CARTESIAN_POINT('Ctrl Pts',(-1.62503464209777,-1.,1.32969019505665));
#43681=CARTESIAN_POINT('Ctrl Pts',(-1.62503464209777,1.,1.32969019505665));
#43682=CARTESIAN_POINT('Ctrl Pts',(-1.61892832270723,-1.,1.32828000610448));
#43683=CARTESIAN_POINT('Ctrl Pts',(-1.61892832270723,1.,1.32828000610448));
#43684=CARTESIAN_POINT('Ctrl Pts',(-1.61284234015762,-1.,1.32683074483365));
#43685=CARTESIAN_POINT('Ctrl Pts',(-1.61284234015762,1.,1.32683074483365));
#43686=CARTESIAN_POINT('Ctrl Pts',(-1.6067775829097,-1.,1.32534250785794));
#43687=CARTESIAN_POINT('Ctrl Pts',(-1.6067775829097,1.,1.32534250785794));
#43688=CARTESIAN_POINT('Ctrl Pts',(-1.600735118587,-1.,1.32381550858266));
#43689=CARTESIAN_POINT('Ctrl Pts',(-1.600735118587,1.,1.32381550858266));
#43690=CARTESIAN_POINT('Ctrl Pts',(-1.59471591079408,-1.,1.32224985747686));
#43691=CARTESIAN_POINT('Ctrl Pts',(-1.59471591079408,1.,1.32224985747686));
#43692=CARTESIAN_POINT('Ctrl Pts',(-1.58872057258244,-1.,1.32064537110891));
#43693=CARTESIAN_POINT('Ctrl Pts',(-1.58872057258244,1.,1.32064537110891));
#43694=CARTESIAN_POINT('Ctrl Pts',(-1.58274907898829,-1.,1.31900135021428));
#43695=CARTESIAN_POINT('Ctrl Pts',(-1.58274907898829,1.,1.31900135021428));
#43696=CARTESIAN_POINT('Ctrl Pts',(-1.57680056505585,-1.,1.31731642317183));
#43697=CARTESIAN_POINT('Ctrl Pts',(-1.57680056505585,1.,1.31731642317183));
#43698=CARTESIAN_POINT('Ctrl Pts',(-1.57087397835721,-1.,1.31558903860015));
#43699=CARTESIAN_POINT('Ctrl Pts',(-1.57087397835721,1.,1.31558903860015));
#43700=CARTESIAN_POINT('Ctrl Pts',(-1.56496872402352,-1.,1.31381795281002));
#43701=CARTESIAN_POINT('Ctrl Pts',(-1.56496872402352,1.,1.31381795281002));
#43702=CARTESIAN_POINT('Ctrl Pts',(-1.55908521254822,-1.,1.31200264341696));
#43703=CARTESIAN_POINT('Ctrl Pts',(-1.55908521254822,1.,1.31200264341696));
#43704=CARTESIAN_POINT('Ctrl Pts',(-1.55322568759481,-1.,1.31014393684221));
#43705=CARTESIAN_POINT('Ctrl Pts',(-1.55322568759481,1.,1.31014393684221));
#43706=CARTESIAN_POINT('Ctrl Pts',(-1.54739413957183,-1.,1.30824393907471));
#43707=CARTESIAN_POINT('Ctrl Pts',(-1.54739413957183,1.,1.30824393907471));
#43708=CARTESIAN_POINT('Ctrl Pts',(-1.54159462645428,-1.,1.30630475189553));
#43709=CARTESIAN_POINT('Ctrl Pts',(-1.54159462645428,1.,1.30630475189553));
#43710=CARTESIAN_POINT('Ctrl Pts',(-1.53582981268976,-1.,1.30432735639487));
#43711=CARTESIAN_POINT('Ctrl Pts',(-1.53582981268976,1.,1.30432735639487));
#43712=CARTESIAN_POINT('Ctrl Pts',(-1.53009970283893,-1.,1.3023106439557));
#43713=CARTESIAN_POINT('Ctrl Pts',(-1.53009970283893,1.,1.3023106439557));
#43714=CARTESIAN_POINT('Ctrl Pts',(-1.5243995786107,-1.,1.30024984366334));
#43715=CARTESIAN_POINT('Ctrl Pts',(-1.5243995786107,1.,1.30024984366334));
#43716=CARTESIAN_POINT('Ctrl Pts',(-1.51872184912735,-1.,1.29813791800757));
#43717=CARTESIAN_POINT('Ctrl Pts',(-1.51872184912735,1.,1.29813791800757));
#43718=CARTESIAN_POINT('Ctrl Pts',(-1.51305994241412,-1.,1.29596850710518));
#43719=CARTESIAN_POINT('Ctrl Pts',(-1.51305994241412,1.,1.29596850710518));
#43720=CARTESIAN_POINT('Ctrl Pts',(-1.50741159078367,-1.,1.29373841372843));
#43721=CARTESIAN_POINT('Ctrl Pts',(-1.50741159078367,1.,1.29373841372843));
#43722=CARTESIAN_POINT('Ctrl Pts',(-1.50178230149764,-1.,1.29145022885171));
#43723=CARTESIAN_POINT('Ctrl Pts',(-1.50178230149764,1.,1.29145022885171));
#43724=CARTESIAN_POINT('Ctrl Pts',(-1.49618896881729,-1.,1.28911506584232));
#43725=CARTESIAN_POINT('Ctrl Pts',(-1.49618896881729,1.,1.28911506584232));
#43726=CARTESIAN_POINT('Ctrl Pts',(-1.4906522831275,-1.,1.28674676116415));
#43727=CARTESIAN_POINT('Ctrl Pts',(-1.4906522831275,1.,1.28674676116415));
#43728=CARTESIAN_POINT('Ctrl Pts',(-1.48518817118891,-1.,1.28435533880184));
#43729=CARTESIAN_POINT('Ctrl Pts',(-1.48518817118891,1.,1.28435533880184));
#43730=CARTESIAN_POINT('Ctrl Pts',(-1.47980070347102,-1.,1.28194158939522));
#43731=CARTESIAN_POINT('Ctrl Pts',(-1.47980070347102,1.,1.28194158939522));
#43732=CARTESIAN_POINT('Ctrl Pts',(-1.4744717526711,-1.,1.27948918248524));
#43733=CARTESIAN_POINT('Ctrl Pts',(-1.4744717526711,1.,1.27948918248524));
#43734=CARTESIAN_POINT('Ctrl Pts',(-1.46916035917197,-1.,1.27696414831144));
#43735=CARTESIAN_POINT('Ctrl Pts',(-1.46916035917197,1.,1.27696414831144));
#43736=CARTESIAN_POINT('Ctrl Pts',(-1.4638243133254,-1.,1.27433119897877));
#43737=CARTESIAN_POINT('Ctrl Pts',(-1.4638243133254,1.,1.27433119897877));
#43738=CARTESIAN_POINT('Ctrl Pts',(-1.45843906294725,-1.,1.27156805265312));
#43739=CARTESIAN_POINT('Ctrl Pts',(-1.45843906294725,1.,1.27156805265312));
#43740=CARTESIAN_POINT('Ctrl Pts',(-1.45301422764205,-1.,1.26867786804854));
#43741=CARTESIAN_POINT('Ctrl Pts',(-1.45301422764205,1.,1.26867786804854));
#43742=CARTESIAN_POINT('Ctrl Pts',(-1.44761985001544,-1.,1.26570925118767));
#43743=CARTESIAN_POINT('Ctrl Pts',(-1.44761985001544,1.,1.26570925118767));
#43744=CARTESIAN_POINT('Ctrl Pts',(-1.44236470511145,-1.,1.26273903323723));
#43745=CARTESIAN_POINT('Ctrl Pts',(-1.44236470511145,1.,1.26273903323723));
#43746=CARTESIAN_POINT('Ctrl Pts',(-1.43734919180719,-1.,1.25983531011894));
#43747=CARTESIAN_POINT('Ctrl Pts',(-1.43734919180719,1.,1.25983531011894));
#43748=CARTESIAN_POINT('Ctrl Pts',(-1.43262645609679,-1.,1.25702687965744));
#43749=CARTESIAN_POINT('Ctrl Pts',(-1.43262645609679,1.,1.25702687965744));
#43750=CARTESIAN_POINT('Ctrl Pts',(-1.42815938799555,-1.,1.25426945222783));
#43751=CARTESIAN_POINT('Ctrl Pts',(-1.42815938799555,1.,1.25426945222783));
#43752=CARTESIAN_POINT('Ctrl Pts',(-1.42378102115911,-1.,1.25141455570299));
#43753=CARTESIAN_POINT('Ctrl Pts',(-1.42378102115911,1.,1.25141455570299));
#43754=CARTESIAN_POINT('Ctrl Pts',(-1.41923722596421,-1.,1.24824430986911));
#43755=CARTESIAN_POINT('Ctrl Pts',(-1.41923722596421,1.,1.24824430986911));
#43756=CARTESIAN_POINT('Ctrl Pts',(-1.41422913175437,-1.,1.24450600513278));
#43757=CARTESIAN_POINT('Ctrl Pts',(-1.41422913175437,1.,1.24450600513278));
#43758=CARTESIAN_POINT('Ctrl Pts',(-1.40845295531151,-1.,1.23994455029421));
#43759=CARTESIAN_POINT('Ctrl Pts',(-1.40845295531151,1.,1.23994455029421));
#43760=CARTESIAN_POINT('Ctrl Pts',(-1.40164708205345,-1.,1.23434087289768));
#43761=CARTESIAN_POINT('Ctrl Pts',(-1.40164708205345,1.,1.23434087289768));
#43762=CARTESIAN_POINT('Ctrl Pts',(-1.39361389567257,-1.,1.22752961898063));
#43763=CARTESIAN_POINT('Ctrl Pts',(-1.39361389567257,1.,1.22752961898063));
#43764=CARTESIAN_POINT('Ctrl Pts',(-1.38420564525391,-1.,1.21938737278853));
#43765=CARTESIAN_POINT('Ctrl Pts',(-1.38420564525391,1.,1.21938737278853));
#43766=CARTESIAN_POINT('Ctrl Pts',(-1.37331915604962,-1.,1.20982812923113));
#43767=CARTESIAN_POINT('Ctrl Pts',(-1.37331915604962,1.,1.20982812923113));
#43768=CARTESIAN_POINT('Ctrl Pts',(-1.36088705040677,-1.,1.1987959077656));
#43769=CARTESIAN_POINT('Ctrl Pts',(-1.36088705040677,1.,1.1987959077656));
#43770=CARTESIAN_POINT('Ctrl Pts',(-1.34687053998157,-1.,1.18625865664915));
#43771=CARTESIAN_POINT('Ctrl Pts',(-1.34687053998157,1.,1.18625865664915));
#43772=CARTESIAN_POINT('Ctrl Pts',(-1.33437539344842,-1.,1.17501305787994));
#43773=CARTESIAN_POINT('Ctrl Pts',(-1.33437539344842,1.,1.17501305787994));
#43774=CARTESIAN_POINT('Ctrl Pts',(-1.32428080720544,-1.,1.16589330092532));
#43775=CARTESIAN_POINT('Ctrl Pts',(-1.32428080720544,1.,1.16589330092532));
#43776=CARTESIAN_POINT('Ctrl Pts',(-1.3172297721596,-1.,1.15950888730433));
#43777=CARTESIAN_POINT('Ctrl Pts',(-1.3172297721596,1.,1.15950888730433));
#43778=CARTESIAN_POINT('Ctrl Pts',(-1.31362392696033,-1.,1.15624053661742));
#43779=CARTESIAN_POINT('Ctrl Pts',(-1.31362392696033,1.,1.15624053661742));
#43780=CARTESIAN_POINT('',(-1.73811241238545,1.,1.34869019493419));
#43781=CARTESIAN_POINT('Ctrl Pts',(-1.73811241238545,1.,1.34869019493419));
#43782=CARTESIAN_POINT('Ctrl Pts',(-1.73682580585819,1.,1.34854391898145));
#43783=CARTESIAN_POINT('Ctrl Pts',(-1.73425417886255,1.,1.34824783113158));
#43784=CARTESIAN_POINT('Ctrl Pts',(-1.73040149654497,1.,1.3477930915247));
#43785=CARTESIAN_POINT('Ctrl Pts',(-1.72527410681298,1.,1.34716554820013));
#43786=CARTESIAN_POINT('Ctrl Pts',(-1.7188807715095,1.,1.34634568653586));
#43787=CARTESIAN_POINT('Ctrl Pts',(-1.71250340687011,1.,1.34549029589563));
#43788=CARTESIAN_POINT('Ctrl Pts',(-1.70614212266676,1.,1.34459924533783));
#43789=CARTESIAN_POINT('Ctrl Pts',(-1.69979707754221,1.,1.34367237124322));
#43790=CARTESIAN_POINT('Ctrl Pts',(-1.6934684849664,1.,1.34270948206139));
#43791=CARTESIAN_POINT('Ctrl Pts',(-1.68715660868602,1.,1.34171037484673));
#43792=CARTESIAN_POINT('Ctrl Pts',(-1.68086176030308,1.,1.3406748518516));
#43793=CARTESIAN_POINT('Ctrl Pts',(-1.67458429426126,1.,1.33960273470372));
#43794=CARTESIAN_POINT('Ctrl Pts',(-1.66832460784078,1.,1.33849388654458));
#43795=CARTESIAN_POINT('Ctrl Pts',(-1.66208312542073,1.,1.33734820885331));
#43796=CARTESIAN_POINT('Ctrl Pts',(-1.65586025952651,1.,1.33616559745217));
#43797=CARTESIAN_POINT('Ctrl Pts',(-1.64965637286843,1.,1.33494590468003));
#43798=CARTESIAN_POINT('Ctrl Pts',(-1.64347174856007,1.,1.33368890676554));
#43799=CARTESIAN_POINT('Ctrl Pts',(-1.6373065347505,1.,1.33239425103694));
#43800=CARTESIAN_POINT('Ctrl Pts',(-1.63116079730887,1.,1.33106149345618));
#43801=CARTESIAN_POINT('Ctrl Pts',(-1.62503464209777,1.,1.32969019505665));
#43802=CARTESIAN_POINT('Ctrl Pts',(-1.61892832270723,1.,1.32828000610448));
#43803=CARTESIAN_POINT('Ctrl Pts',(-1.61284234015762,1.,1.32683074483365));
#43804=CARTESIAN_POINT('Ctrl Pts',(-1.6067775829097,1.,1.32534250785794));
#43805=CARTESIAN_POINT('Ctrl Pts',(-1.600735118587,1.,1.32381550858266));
#43806=CARTESIAN_POINT('Ctrl Pts',(-1.59471591079408,1.,1.32224985747686));
#43807=CARTESIAN_POINT('Ctrl Pts',(-1.58872057258244,1.,1.32064537110891));
#43808=CARTESIAN_POINT('Ctrl Pts',(-1.58274907898829,1.,1.31900135021428));
#43809=CARTESIAN_POINT('Ctrl Pts',(-1.57680056505585,1.,1.31731642317183));
#43810=CARTESIAN_POINT('Ctrl Pts',(-1.57087397835721,1.,1.31558903860015));
#43811=CARTESIAN_POINT('Ctrl Pts',(-1.56496872402352,1.,1.31381795281002));
#43812=CARTESIAN_POINT('Ctrl Pts',(-1.55908521254822,1.,1.31200264341696));
#43813=CARTESIAN_POINT('Ctrl Pts',(-1.55322568759481,1.,1.31014393684221));
#43814=CARTESIAN_POINT('Ctrl Pts',(-1.54739413957183,1.,1.30824393907471));
#43815=CARTESIAN_POINT('Ctrl Pts',(-1.54159462645428,1.,1.30630475189553));
#43816=CARTESIAN_POINT('Ctrl Pts',(-1.53582981268976,1.,1.30432735639487));
#43817=CARTESIAN_POINT('Ctrl Pts',(-1.53009970283893,1.,1.3023106439557));
#43818=CARTESIAN_POINT('Ctrl Pts',(-1.5243995786107,1.,1.30024984366334));
#43819=CARTESIAN_POINT('Ctrl Pts',(-1.51872184912735,1.,1.29813791800757));
#43820=CARTESIAN_POINT('Ctrl Pts',(-1.51305994241412,1.,1.29596850710518));
#43821=CARTESIAN_POINT('Ctrl Pts',(-1.50741159078367,1.,1.29373841372843));
#43822=CARTESIAN_POINT('Ctrl Pts',(-1.50178230149764,1.,1.29145022885171));
#43823=CARTESIAN_POINT('Ctrl Pts',(-1.49618896881729,1.,1.28911506584232));
#43824=CARTESIAN_POINT('Ctrl Pts',(-1.4906522831275,1.,1.28674676116415));
#43825=CARTESIAN_POINT('Ctrl Pts',(-1.48518817118891,1.,1.28435533880184));
#43826=CARTESIAN_POINT('Ctrl Pts',(-1.47980070347102,1.,1.28194158939522));
#43827=CARTESIAN_POINT('Ctrl Pts',(-1.4744717526711,1.,1.27948918248524));
#43828=CARTESIAN_POINT('Ctrl Pts',(-1.46916035917197,1.,1.27696414831144));
#43829=CARTESIAN_POINT('Ctrl Pts',(-1.4638243133254,1.,1.27433119897877));
#43830=CARTESIAN_POINT('Ctrl Pts',(-1.45843906294725,1.,1.27156805265312));
#43831=CARTESIAN_POINT('Ctrl Pts',(-1.45301422764205,1.,1.26867786804854));
#43832=CARTESIAN_POINT('Ctrl Pts',(-1.44761985001544,1.,1.26570925118767));
#43833=CARTESIAN_POINT('Ctrl Pts',(-1.44236470511145,1.,1.26273903323723));
#43834=CARTESIAN_POINT('Ctrl Pts',(-1.43734919180719,1.,1.25983531011894));
#43835=CARTESIAN_POINT('Ctrl Pts',(-1.43262645609679,1.,1.25702687965744));
#43836=CARTESIAN_POINT('Ctrl Pts',(-1.42815938799555,1.,1.25426945222783));
#43837=CARTESIAN_POINT('Ctrl Pts',(-1.42378102115911,1.,1.25141455570299));
#43838=CARTESIAN_POINT('Ctrl Pts',(-1.41923722596421,1.,1.24824430986911));
#43839=CARTESIAN_POINT('Ctrl Pts',(-1.41422913175437,1.,1.24450600513278));
#43840=CARTESIAN_POINT('Ctrl Pts',(-1.40845295531151,1.,1.23994455029421));
#43841=CARTESIAN_POINT('Ctrl Pts',(-1.40164708205345,1.,1.23434087289768));
#43842=CARTESIAN_POINT('Ctrl Pts',(-1.39361389567257,1.,1.22752961898063));
#43843=CARTESIAN_POINT('Ctrl Pts',(-1.38420564525391,1.,1.21938737278853));
#43844=CARTESIAN_POINT('Ctrl Pts',(-1.37331915604962,1.,1.20982812923113));
#43845=CARTESIAN_POINT('Ctrl Pts',(-1.36088705040677,1.,1.1987959077656));
#43846=CARTESIAN_POINT('Ctrl Pts',(-1.34687053998157,1.,1.18625865664915));
#43847=CARTESIAN_POINT('Ctrl Pts',(-1.33437539344842,1.,1.17501305787994));
#43848=CARTESIAN_POINT('Ctrl Pts',(-1.32428080720544,1.,1.16589330092532));
#43849=CARTESIAN_POINT('Ctrl Pts',(-1.3172297721596,1.,1.15950888730433));
#43850=CARTESIAN_POINT('Ctrl Pts',(-1.31362392696033,1.,1.15624053661742));
#43851=CARTESIAN_POINT('',(-1.73811241238545,0.,1.34869019493419));
#43852=CARTESIAN_POINT('Origin',(-1.81978687191668,0.,1.23627494547115));
#43853=CARTESIAN_POINT('',(-1.81978687191668,1.,1.23627494547115));
#43854=CARTESIAN_POINT('',(-1.73811241238545,1.,1.34869019493419));
#43855=CARTESIAN_POINT('',(-1.81978687191668,0.,1.23627494547115));
#43856=CARTESIAN_POINT('Ctrl Pts',(-1.5055822144029,-1.,0.892032620296855));
#43857=CARTESIAN_POINT('Ctrl Pts',(-1.5055822144029,1.,0.892032620296855));
#43858=CARTESIAN_POINT('Ctrl Pts',(-1.50980486807181,-1.,0.894452006967538));
#43859=CARTESIAN_POINT('Ctrl Pts',(-1.50980486807181,1.,0.894452006967538));
#43860=CARTESIAN_POINT('Ctrl Pts',(-1.51805569591479,-1.,0.89918504749193));
#43861=CARTESIAN_POINT('Ctrl Pts',(-1.51805569591479,1.,0.89918504749193));
#43862=CARTESIAN_POINT('Ctrl Pts',(-1.52984849890434,-1.,0.905967409640499));
#43863=CARTESIAN_POINT('Ctrl Pts',(-1.52984849890434,1.,0.905967409640499));
#43864=CARTESIAN_POINT('Ctrl Pts',(-1.54440491152808,-1.,0.91437591904658));
#43865=CARTESIAN_POINT('Ctrl Pts',(-1.54440491152808,1.,0.91437591904658));
#43866=CARTESIAN_POINT('Ctrl Pts',(-1.56065988582509,-1.,0.923832188966322));
#43867=CARTESIAN_POINT('Ctrl Pts',(-1.56065988582509,1.,0.923832188966322));
#43868=CARTESIAN_POINT('Ctrl Pts',(-1.57499388385561,-1.,0.932246680128849));
#43869=CARTESIAN_POINT('Ctrl Pts',(-1.57499388385561,1.,0.932246680128849));
#43870=CARTESIAN_POINT('Ctrl Pts',(-1.58744937489796,-1.,0.939646377909319));
#43871=CARTESIAN_POINT('Ctrl Pts',(-1.58744937489796,1.,0.939646377909319));
#43872=CARTESIAN_POINT('Ctrl Pts',(-1.59810042045408,-1.,0.946078063325796));
#43873=CARTESIAN_POINT('Ctrl Pts',(-1.59810042045408,1.,0.946078063325796));
#43874=CARTESIAN_POINT('Ctrl Pts',(-1.60706069897794,-1.,0.951613284361248));
#43875=CARTESIAN_POINT('Ctrl Pts',(-1.60706069897794,1.,0.951613284361248));
#43876=CARTESIAN_POINT('Ctrl Pts',(-1.61449324337233,-1.,0.956354422921573));
#43877=CARTESIAN_POINT('Ctrl Pts',(-1.61449324337233,1.,0.956354422921573));
#43878=CARTESIAN_POINT('Ctrl Pts',(-1.62061638139929,-1.,0.960438326099958));
#43879=CARTESIAN_POINT('Ctrl Pts',(-1.62061638139929,1.,0.960438326099958));
#43880=CARTESIAN_POINT('Ctrl Pts',(-1.6257193066974,-1.,0.964046107037821));
#43881=CARTESIAN_POINT('Ctrl Pts',(-1.6257193066974,1.,0.964046107037821));
#43882=CARTESIAN_POINT('Ctrl Pts',(-1.63013849959083,-1.,0.967387853228041));
#43883=CARTESIAN_POINT('Ctrl Pts',(-1.63013849959083,1.,0.967387853228041));
#43884=CARTESIAN_POINT('Ctrl Pts',(-1.63420665729609,-1.,0.970669715996356));
#43885=CARTESIAN_POINT('Ctrl Pts',(-1.63420665729609,1.,0.970669715996356));
#43886=CARTESIAN_POINT('Ctrl Pts',(-1.63820952658157,-1.,0.974066058287501));
#43887=CARTESIAN_POINT('Ctrl Pts',(-1.63820952658157,1.,0.974066058287501));
#43888=CARTESIAN_POINT('Ctrl Pts',(-1.64233990826831,-1.,0.977689794120297));
#43889=CARTESIAN_POINT('Ctrl Pts',(-1.64233990826831,1.,0.977689794120297));
#43890=CARTESIAN_POINT('Ctrl Pts',(-1.64665139190834,-1.,0.981562530940574));
#43891=CARTESIAN_POINT('Ctrl Pts',(-1.64665139190834,1.,0.981562530940574));
#43892=CARTESIAN_POINT('Ctrl Pts',(-1.6511001661277,-1.,0.985642622921626));
#43893=CARTESIAN_POINT('Ctrl Pts',(-1.6511001661277,1.,0.985642622921626));
#43894=CARTESIAN_POINT('Ctrl Pts',(-1.65559044289746,-1.,0.98985562785445));
#43895=CARTESIAN_POINT('Ctrl Pts',(-1.65559044289746,1.,0.98985562785445));
#43896=CARTESIAN_POINT('Ctrl Pts',(-1.66001553809916,-1.,0.994121836661116));
#43897=CARTESIAN_POINT('Ctrl Pts',(-1.66001553809916,1.,0.994121836661116));
#43898=CARTESIAN_POINT('Ctrl Pts',(-1.66430758030304,-1.,0.998389654952317));
#43899=CARTESIAN_POINT('Ctrl Pts',(-1.66430758030304,1.,0.998389654952317));
#43900=CARTESIAN_POINT('Ctrl Pts',(-1.66846059277231,-1.,1.00265091003682));
#43901=CARTESIAN_POINT('Ctrl Pts',(-1.66846059277231,1.,1.00265091003682));
#43902=CARTESIAN_POINT('Ctrl Pts',(-1.67250335383248,-1.,1.00692206696387));
#43903=CARTESIAN_POINT('Ctrl Pts',(-1.67250335383248,1.,1.00692206696387));
#43904=CARTESIAN_POINT('Ctrl Pts',(-1.67648246776457,-1.,1.01123236493507));
#43905=CARTESIAN_POINT('Ctrl Pts',(-1.67648246776457,1.,1.01123236493507));
#43906=CARTESIAN_POINT('Ctrl Pts',(-1.6804428989482,-1.,1.01561026162787));
#43907=CARTESIAN_POINT('Ctrl Pts',(-1.6804428989482,1.,1.01561026162787));
#43908=CARTESIAN_POINT('Ctrl Pts',(-1.68440578021739,-1.,1.02006795074222));
#43909=CARTESIAN_POINT('Ctrl Pts',(-1.68440578021739,1.,1.02006795074222));
#43910=CARTESIAN_POINT('Ctrl Pts',(-1.68836910178475,-1.,1.02460180535272));
#43911=CARTESIAN_POINT('Ctrl Pts',(-1.68836910178475,1.,1.02460180535272));
#43912=CARTESIAN_POINT('Ctrl Pts',(-1.69231840863471,-1.,1.02919977579155));
#43913=CARTESIAN_POINT('Ctrl Pts',(-1.69231840863471,1.,1.02919977579155));
#43914=CARTESIAN_POINT('Ctrl Pts',(-1.69623414782769,-1.,1.03384646003587));
#43915=CARTESIAN_POINT('Ctrl Pts',(-1.69623414782769,1.,1.03384646003587));
#43916=CARTESIAN_POINT('Ctrl Pts',(-1.70010052930951,-1.,1.03852922490782));
#43917=CARTESIAN_POINT('Ctrl Pts',(-1.70010052930951,1.,1.03852922490782));
#43918=CARTESIAN_POINT('Ctrl Pts',(-1.70391338707969,-1.,1.04324363334546));
#43919=CARTESIAN_POINT('Ctrl Pts',(-1.70391338707969,1.,1.04324363334546));
#43920=CARTESIAN_POINT('Ctrl Pts',(-1.70767646263641,-1.,1.0479908540499));
#43921=CARTESIAN_POINT('Ctrl Pts',(-1.70767646263641,1.,1.0479908540499));
#43922=CARTESIAN_POINT('Ctrl Pts',(-1.71139783543986,-1.,1.05277517202854));
#43923=CARTESIAN_POINT('Ctrl Pts',(-1.71139783543986,1.,1.05277517202854));
#43924=CARTESIAN_POINT('Ctrl Pts',(-1.71508654427022,-1.,1.05760163192481));
#43925=CARTESIAN_POINT('Ctrl Pts',(-1.71508654427022,1.,1.05760163192481));
#43926=CARTESIAN_POINT('Ctrl Pts',(-1.71874858456908,-1.,1.0624732468065));
#43927=CARTESIAN_POINT('Ctrl Pts',(-1.71874858456908,1.,1.0624732468065));
#43928=CARTESIAN_POINT('Ctrl Pts',(-1.72238500928456,-1.,1.06738966975463));
#43929=CARTESIAN_POINT('Ctrl Pts',(-1.72238500928456,1.,1.06738966975463));
#43930=CARTESIAN_POINT('Ctrl Pts',(-1.72599406198489,-1.,1.07234866990252));
#43931=CARTESIAN_POINT('Ctrl Pts',(-1.72599406198489,1.,1.07234866990252));
#43932=CARTESIAN_POINT('Ctrl Pts',(-1.72957248977424,-1.,1.0773470373727));
#43933=CARTESIAN_POINT('Ctrl Pts',(-1.72957248977424,1.,1.0773470373727));
#43934=CARTESIAN_POINT('Ctrl Pts',(-1.73311705663407,-1.,1.08238162784749));
#43935=CARTESIAN_POINT('Ctrl Pts',(-1.73311705663407,1.,1.08238162784749));
#43936=CARTESIAN_POINT('Ctrl Pts',(-1.73662628326093,-1.,1.08745056285429));
#43937=CARTESIAN_POINT('Ctrl Pts',(-1.73662628326093,1.,1.08745056285429));
#43938=CARTESIAN_POINT('Ctrl Pts',(-1.74010053962252,-1.,1.09255329056496));
#43939=CARTESIAN_POINT('Ctrl Pts',(-1.74010053962252,1.,1.09255329056496));
#43940=CARTESIAN_POINT('Ctrl Pts',(-1.74354119236212,-1.,1.09768999241229));
#43941=CARTESIAN_POINT('Ctrl Pts',(-1.74354119236212,1.,1.09768999241229));
#43942=CARTESIAN_POINT('Ctrl Pts',(-1.74695004214924,-1.,1.10286118991144));
#43943=CARTESIAN_POINT('Ctrl Pts',(-1.74695004214924,1.,1.10286118991144));
#43944=CARTESIAN_POINT('Ctrl Pts',(-1.75032866075914,-1.,1.10806728183003));
#43945=CARTESIAN_POINT('Ctrl Pts',(-1.75032866075914,1.,1.10806728183003));
#43946=CARTESIAN_POINT('Ctrl Pts',(-1.75367772094617,-1.,1.11330807582542));
#43947=CARTESIAN_POINT('Ctrl Pts',(-1.75367772094617,1.,1.11330807582542));
#43948=CARTESIAN_POINT('Ctrl Pts',(-1.75699720772089,-1.,1.11858293216752));
#43949=CARTESIAN_POINT('Ctrl Pts',(-1.75699720772089,1.,1.11858293216752));
#43950=CARTESIAN_POINT('Ctrl Pts',(-1.76028671825084,-1.,1.12389096855078));
#43951=CARTESIAN_POINT('Ctrl Pts',(-1.76028671825084,1.,1.12389096855078));
#43952=CARTESIAN_POINT('Ctrl Pts',(-1.76354571966171,-1.,1.12923123555076));
#43953=CARTESIAN_POINT('Ctrl Pts',(-1.76354571966171,1.,1.12923123555076));
#43954=CARTESIAN_POINT('Ctrl Pts',(-1.76677384551883,-1.,1.13460291804635));
#43955=CARTESIAN_POINT('Ctrl Pts',(-1.76677384551883,1.,1.13460291804635));
#43956=CARTESIAN_POINT('Ctrl Pts',(-1.76997111386806,-1.,1.14000548337));
#43957=CARTESIAN_POINT('Ctrl Pts',(-1.76997111386806,1.,1.14000548337));
#43958=CARTESIAN_POINT('Ctrl Pts',(-1.77313777896234,-1.,1.14543858226948));
#43959=CARTESIAN_POINT('Ctrl Pts',(-1.77313777896234,1.,1.14543858226948));
#43960=CARTESIAN_POINT('Ctrl Pts',(-1.77627422557034,-1.,1.15090197841531));
#43961=CARTESIAN_POINT('Ctrl Pts',(-1.77627422557034,1.,1.15090197841531));
#43962=CARTESIAN_POINT('Ctrl Pts',(-1.77938085564261,-1.,1.15639547194689));
#43963=CARTESIAN_POINT('Ctrl Pts',(-1.77938085564261,1.,1.15639547194689));
#43964=CARTESIAN_POINT('Ctrl Pts',(-1.78245795880949,-1.,1.16191881298458));
#43965=CARTESIAN_POINT('Ctrl Pts',(-1.78245795880949,1.,1.16191881298458));
#43966=CARTESIAN_POINT('Ctrl Pts',(-1.78550566040349,-1.,1.16747166312239));
#43967=CARTESIAN_POINT('Ctrl Pts',(-1.78550566040349,1.,1.16747166312239));
#43968=CARTESIAN_POINT('Ctrl Pts',(-1.78852398877523,-1.,1.17305363177265));
#43969=CARTESIAN_POINT('Ctrl Pts',(-1.78852398877523,1.,1.17305363177265));
#43970=CARTESIAN_POINT('Ctrl Pts',(-1.79151291552646,-1.,1.17866429440781));
#43971=CARTESIAN_POINT('Ctrl Pts',(-1.79151291552646,1.,1.17866429440781));
#43972=CARTESIAN_POINT('Ctrl Pts',(-1.79447240321572,-1.,1.18430321697471));
#43973=CARTESIAN_POINT('Ctrl Pts',(-1.79447240321572,1.,1.18430321697471));
#43974=CARTESIAN_POINT('Ctrl Pts',(-1.79740245923649,-1.,1.1899699793456));
#43975=CARTESIAN_POINT('Ctrl Pts',(-1.79740245923649,1.,1.1899699793456));
#43976=CARTESIAN_POINT('Ctrl Pts',(-1.80030314370121,-1.,1.19566418930405));
#43977=CARTESIAN_POINT('Ctrl Pts',(-1.80030314370121,1.,1.19566418930405));
#43978=CARTESIAN_POINT('Ctrl Pts',(-1.8031745483882,-1.,1.2013854893912));
#43979=CARTESIAN_POINT('Ctrl Pts',(-1.8031745483882,1.,1.2013854893912));
#43980=CARTESIAN_POINT('Ctrl Pts',(-1.80601678480772,-1.,1.20713356605519));
#43981=CARTESIAN_POINT('Ctrl Pts',(-1.80601678480772,1.,1.20713356605519));
#43982=CARTESIAN_POINT('Ctrl Pts',(-1.80882996916931,-1.,1.2129081570818));
#43983=CARTESIAN_POINT('Ctrl Pts',(-1.80882996916931,1.,1.2129081570818));
#43984=CARTESIAN_POINT('Ctrl Pts',(-1.81161420806172,-1.,1.2187090610323));
#43985=CARTESIAN_POINT('Ctrl Pts',(-1.81161420806172,1.,1.2187090610323));
#43986=CARTESIAN_POINT('Ctrl Pts',(-1.81436959209778,-1.,1.22453613304507));
#43987=CARTESIAN_POINT('Ctrl Pts',(-1.81436959209778,1.,1.22453613304507));
#43988=CARTESIAN_POINT('Ctrl Pts',(-1.81655087183054,-1.,1.22921864890975));
#43989=CARTESIAN_POINT('Ctrl Pts',(-1.81655087183054,1.,1.22921864890975));
#43990=CARTESIAN_POINT('Ctrl Pts',(-1.81817389920914,-1.,1.23274224526804));
#43991=CARTESIAN_POINT('Ctrl Pts',(-1.81817389920914,1.,1.23274224526804));
#43992=CARTESIAN_POINT('Ctrl Pts',(-1.81925017193531,-1.,1.23509651170384));
#43993=CARTESIAN_POINT('Ctrl Pts',(-1.81925017193531,1.,1.23509651170384));
#43994=CARTESIAN_POINT('Ctrl Pts',(-1.81978687191668,-1.,1.23627494547115));
#43995=CARTESIAN_POINT('Ctrl Pts',(-1.81978687191668,1.,1.23627494547115));
#43996=CARTESIAN_POINT('',(-1.5055822144029,1.,0.892032620296855));
#43997=CARTESIAN_POINT('Ctrl Pts',(-1.5055822144029,1.,0.892032620296855));
#43998=CARTESIAN_POINT('Ctrl Pts',(-1.50980486807181,1.,0.894452006967538));
#43999=CARTESIAN_POINT('Ctrl Pts',(-1.51805569591479,1.,0.89918504749193));
#44000=CARTESIAN_POINT('Ctrl Pts',(-1.52984849890434,1.,0.905967409640499));
#44001=CARTESIAN_POINT('Ctrl Pts',(-1.54440491152808,1.,0.91437591904658));
#44002=CARTESIAN_POINT('Ctrl Pts',(-1.56065988582509,1.,0.923832188966322));
#44003=CARTESIAN_POINT('Ctrl Pts',(-1.57499388385561,1.,0.932246680128849));
#44004=CARTESIAN_POINT('Ctrl Pts',(-1.58744937489796,1.,0.939646377909319));
#44005=CARTESIAN_POINT('Ctrl Pts',(-1.59810042045408,1.,0.946078063325796));
#44006=CARTESIAN_POINT('Ctrl Pts',(-1.60706069897794,1.,0.951613284361248));
#44007=CARTESIAN_POINT('Ctrl Pts',(-1.61449324337233,1.,0.956354422921573));
#44008=CARTESIAN_POINT('Ctrl Pts',(-1.62061638139929,1.,0.960438326099958));
#44009=CARTESIAN_POINT('Ctrl Pts',(-1.6257193066974,1.,0.964046107037821));
#44010=CARTESIAN_POINT('Ctrl Pts',(-1.63013849959083,1.,0.967387853228041));
#44011=CARTESIAN_POINT('Ctrl Pts',(-1.63420665729609,1.,0.970669715996356));
#44012=CARTESIAN_POINT('Ctrl Pts',(-1.63820952658157,1.,0.974066058287501));
#44013=CARTESIAN_POINT('Ctrl Pts',(-1.64233990826831,1.,0.977689794120297));
#44014=CARTESIAN_POINT('Ctrl Pts',(-1.64665139190834,1.,0.981562530940574));
#44015=CARTESIAN_POINT('Ctrl Pts',(-1.6511001661277,1.,0.985642622921626));
#44016=CARTESIAN_POINT('Ctrl Pts',(-1.65559044289746,1.,0.98985562785445));
#44017=CARTESIAN_POINT('Ctrl Pts',(-1.66001553809916,1.,0.994121836661116));
#44018=CARTESIAN_POINT('Ctrl Pts',(-1.66430758030304,1.,0.998389654952317));
#44019=CARTESIAN_POINT('Ctrl Pts',(-1.66846059277231,1.,1.00265091003682));
#44020=CARTESIAN_POINT('Ctrl Pts',(-1.67250335383248,1.,1.00692206696387));
#44021=CARTESIAN_POINT('Ctrl Pts',(-1.67648246776457,1.,1.01123236493507));
#44022=CARTESIAN_POINT('Ctrl Pts',(-1.6804428989482,1.,1.01561026162787));
#44023=CARTESIAN_POINT('Ctrl Pts',(-1.68440578021739,1.,1.02006795074222));
#44024=CARTESIAN_POINT('Ctrl Pts',(-1.68836910178475,1.,1.02460180535272));
#44025=CARTESIAN_POINT('Ctrl Pts',(-1.69231840863471,1.,1.02919977579155));
#44026=CARTESIAN_POINT('Ctrl Pts',(-1.69623414782769,1.,1.03384646003587));
#44027=CARTESIAN_POINT('Ctrl Pts',(-1.70010052930951,1.,1.03852922490782));
#44028=CARTESIAN_POINT('Ctrl Pts',(-1.70391338707969,1.,1.04324363334546));
#44029=CARTESIAN_POINT('Ctrl Pts',(-1.70767646263641,1.,1.0479908540499));
#44030=CARTESIAN_POINT('Ctrl Pts',(-1.71139783543986,1.,1.05277517202854));
#44031=CARTESIAN_POINT('Ctrl Pts',(-1.71508654427022,1.,1.05760163192481));
#44032=CARTESIAN_POINT('Ctrl Pts',(-1.71874858456908,1.,1.0624732468065));
#44033=CARTESIAN_POINT('Ctrl Pts',(-1.72238500928456,1.,1.06738966975463));
#44034=CARTESIAN_POINT('Ctrl Pts',(-1.72599406198489,1.,1.07234866990252));
#44035=CARTESIAN_POINT('Ctrl Pts',(-1.72957248977424,1.,1.0773470373727));
#44036=CARTESIAN_POINT('Ctrl Pts',(-1.73311705663407,1.,1.08238162784749));
#44037=CARTESIAN_POINT('Ctrl Pts',(-1.73662628326093,1.,1.08745056285429));
#44038=CARTESIAN_POINT('Ctrl Pts',(-1.74010053962252,1.,1.09255329056496));
#44039=CARTESIAN_POINT('Ctrl Pts',(-1.74354119236212,1.,1.09768999241229));
#44040=CARTESIAN_POINT('Ctrl Pts',(-1.74695004214924,1.,1.10286118991144));
#44041=CARTESIAN_POINT('Ctrl Pts',(-1.75032866075914,1.,1.10806728183003));
#44042=CARTESIAN_POINT('Ctrl Pts',(-1.75367772094617,1.,1.11330807582542));
#44043=CARTESIAN_POINT('Ctrl Pts',(-1.75699720772089,1.,1.11858293216752));
#44044=CARTESIAN_POINT('Ctrl Pts',(-1.76028671825084,1.,1.12389096855078));
#44045=CARTESIAN_POINT('Ctrl Pts',(-1.76354571966171,1.,1.12923123555076));
#44046=CARTESIAN_POINT('Ctrl Pts',(-1.76677384551883,1.,1.13460291804635));
#44047=CARTESIAN_POINT('Ctrl Pts',(-1.76997111386806,1.,1.14000548337));
#44048=CARTESIAN_POINT('Ctrl Pts',(-1.77313777896234,1.,1.14543858226948));
#44049=CARTESIAN_POINT('Ctrl Pts',(-1.77627422557034,1.,1.15090197841531));
#44050=CARTESIAN_POINT('Ctrl Pts',(-1.77938085564261,1.,1.15639547194689));
#44051=CARTESIAN_POINT('Ctrl Pts',(-1.78245795880949,1.,1.16191881298458));
#44052=CARTESIAN_POINT('Ctrl Pts',(-1.78550566040349,1.,1.16747166312239));
#44053=CARTESIAN_POINT('Ctrl Pts',(-1.78852398877523,1.,1.17305363177265));
#44054=CARTESIAN_POINT('Ctrl Pts',(-1.79151291552646,1.,1.17866429440781));
#44055=CARTESIAN_POINT('Ctrl Pts',(-1.79447240321572,1.,1.18430321697471));
#44056=CARTESIAN_POINT('Ctrl Pts',(-1.79740245923649,1.,1.1899699793456));
#44057=CARTESIAN_POINT('Ctrl Pts',(-1.80030314370121,1.,1.19566418930405));
#44058=CARTESIAN_POINT('Ctrl Pts',(-1.8031745483882,1.,1.2013854893912));
#44059=CARTESIAN_POINT('Ctrl Pts',(-1.80601678480772,1.,1.20713356605519));
#44060=CARTESIAN_POINT('Ctrl Pts',(-1.80882996916931,1.,1.2129081570818));
#44061=CARTESIAN_POINT('Ctrl Pts',(-1.81161420806172,1.,1.2187090610323));
#44062=CARTESIAN_POINT('Ctrl Pts',(-1.81436959209778,1.,1.22453613304507));
#44063=CARTESIAN_POINT('Ctrl Pts',(-1.81655087183054,1.,1.22921864890975));
#44064=CARTESIAN_POINT('Ctrl Pts',(-1.81817389920914,1.,1.23274224526804));
#44065=CARTESIAN_POINT('Ctrl Pts',(-1.81925017193531,1.,1.23509651170384));
#44066=CARTESIAN_POINT('Ctrl Pts',(-1.81978687191668,1.,1.23627494547115));
#44067=CARTESIAN_POINT('',(-1.5055822144029,0.,0.892032620296856));
#44068=CARTESIAN_POINT('Origin',(0.,0.,0.));
#44069=CARTESIAN_POINT('',(-1.60662857109684,1.,0.693717979106305));
#44070=CARTESIAN_POINT('Origin',(0.,1.,0.));
#44071=CARTESIAN_POINT('',(-1.60662857109684,0.,0.693717979106306));
#44072=CARTESIAN_POINT('Ctrl Pts',(-2.0698113262342,-1.,0.7455743247944));
#44073=CARTESIAN_POINT('Ctrl Pts',(-2.0698113262342,1.,0.7455743247944));
#44074=CARTESIAN_POINT('Ctrl Pts',(-2.06854248895728,-1.,0.745832791378367));
#44075=CARTESIAN_POINT('Ctrl Pts',(-2.06854248895728,1.,0.745832791378367));
#44076=CARTESIAN_POINT('Ctrl Pts',(-2.06600523016815,-1.,0.7463458715442));
#44077=CARTESIAN_POINT('Ctrl Pts',(-2.06600523016815,1.,0.7463458715442));
#44078=CARTESIAN_POINT('Ctrl Pts',(-2.06220058927826,-1.,0.747103932787919));
#44079=CARTESIAN_POINT('Ctrl Pts',(-2.06220058927826,1.,0.747103932787919));
#44080=CARTESIAN_POINT('Ctrl Pts',(-2.05713023031006,-1.,0.748091554183802));
#44081=CARTESIAN_POINT('Ctrl Pts',(-2.05713023031006,1.,0.748091554183802));
#44082=CARTESIAN_POINT('Ctrl Pts',(-2.05079645592154,-1.,0.749287468665046));
#44083=CARTESIAN_POINT('Ctrl Pts',(-2.05079645592154,1.,0.749287468665046));
#44084=CARTESIAN_POINT('Ctrl Pts',(-2.04446689147979,-1.,0.750444657875576));
#44085=CARTESIAN_POINT('Ctrl Pts',(-2.04446689147979,1.,0.750444657875576));
#44086=CARTESIAN_POINT('Ctrl Pts',(-2.03814160092099,-1.,0.751562963361115));
#44087=CARTESIAN_POINT('Ctrl Pts',(-2.03814160092099,1.,0.751562963361115));
#44088=CARTESIAN_POINT('Ctrl Pts',(-2.03182068456221,-1.,0.752642180487211));
#44089=CARTESIAN_POINT('Ctrl Pts',(-2.03182068456221,1.,0.752642180487211));
#44090=CARTESIAN_POINT('Ctrl Pts',(-2.02550428623313,-1.,0.753682061112768));
#44091=CARTESIAN_POINT('Ctrl Pts',(-2.02550428623313,1.,0.753682061112768));
#44092=CARTESIAN_POINT('Ctrl Pts',(-2.01919259405809,-1.,0.754682330722816));
#44093=CARTESIAN_POINT('Ctrl Pts',(-2.01919259405809,1.,0.754682330722816));
#44094=CARTESIAN_POINT('Ctrl Pts',(-2.01288584328084,-1.,0.755642704957865));
#44095=CARTESIAN_POINT('Ctrl Pts',(-2.01288584328084,1.,0.755642704957865));
#44096=CARTESIAN_POINT('Ctrl Pts',(-2.0065843158773,-1.,0.75656290464667));
#44097=CARTESIAN_POINT('Ctrl Pts',(-2.0065843158773,1.,0.75656290464667));
#44098=CARTESIAN_POINT('Ctrl Pts',(-2.00028834739178,-1.,0.757442676862724));
#44099=CARTESIAN_POINT('Ctrl Pts',(-2.00028834739178,1.,0.757442676862724));
#44100=CARTESIAN_POINT('Ctrl Pts',(-1.99399831098817,-1.,0.758281796766761));
#44101=CARTESIAN_POINT('Ctrl Pts',(-1.99399831098817,1.,0.758281796766761));
#44102=CARTESIAN_POINT('Ctrl Pts',(-1.98771456680874,-1.,0.759080037802488));
#44103=CARTESIAN_POINT('Ctrl Pts',(-1.98771456680874,1.,0.759080037802488));
#44104=CARTESIAN_POINT('Ctrl Pts',(-1.98143741418172,-1.,0.75983714745219));
#44105=CARTESIAN_POINT('Ctrl Pts',(-1.98143741418172,1.,0.75983714745219));
#44106=CARTESIAN_POINT('Ctrl Pts',(-1.97516705321494,-1.,0.760552825409757));
#44107=CARTESIAN_POINT('Ctrl Pts',(-1.97516705321494,1.,0.760552825409757));
#44108=CARTESIAN_POINT('Ctrl Pts',(-1.96890351582499,-1.,0.76122669048382));
#44109=CARTESIAN_POINT('Ctrl Pts',(-1.96890351582499,1.,0.76122669048382));
#44110=CARTESIAN_POINT('Ctrl Pts',(-1.96264672744186,-1.,0.761858300014423));
#44111=CARTESIAN_POINT('Ctrl Pts',(-1.96264672744186,1.,0.761858300014423));
#44112=CARTESIAN_POINT('Ctrl Pts',(-1.95639665309869,-1.,0.762447203806179));
#44113=CARTESIAN_POINT('Ctrl Pts',(-1.95639665309869,1.,0.762447203806179));
#44114=CARTESIAN_POINT('Ctrl Pts',(-1.95015342590024,-1.,0.762992990878769));
#44115=CARTESIAN_POINT('Ctrl Pts',(-1.95015342590024,1.,0.762992990878769));
#44116=CARTESIAN_POINT('Ctrl Pts',(-1.9439174661764,-1.,0.763495333538629));
#44117=CARTESIAN_POINT('Ctrl Pts',(-1.9439174661764,1.,0.763495333538629));
#44118=CARTESIAN_POINT('Ctrl Pts',(-1.93768964875886,-1.,0.763954049121458));
#44119=CARTESIAN_POINT('Ctrl Pts',(-1.93768964875886,1.,0.763954049121458));
#44120=CARTESIAN_POINT('Ctrl Pts',(-1.93147105496382,-1.,0.76436901067394));
#44121=CARTESIAN_POINT('Ctrl Pts',(-1.93147105496382,1.,0.76436901067394));
#44122=CARTESIAN_POINT('Ctrl Pts',(-1.92526263537048,-1.,0.764740025488211));
#44123=CARTESIAN_POINT('Ctrl Pts',(-1.92526263537048,1.,0.764740025488211));
#44124=CARTESIAN_POINT('Ctrl Pts',(-1.91906491634196,-1.,0.765066729667088));
#44125=CARTESIAN_POINT('Ctrl Pts',(-1.91906491634196,1.,0.765066729667088));
#44126=CARTESIAN_POINT('Ctrl Pts',(-1.91287765805169,-1.,0.765348465884722));
#44127=CARTESIAN_POINT('Ctrl Pts',(-1.91287765805169,1.,0.765348465884722));
#44128=CARTESIAN_POINT('Ctrl Pts',(-1.90669961402356,-1.,0.765584196937919));
#44129=CARTESIAN_POINT('Ctrl Pts',(-1.90669961402356,1.,0.765584196937919));
#44130=CARTESIAN_POINT('Ctrl Pts',(-1.90052930393596,-1.,0.765772772593386));
#44131=CARTESIAN_POINT('Ctrl Pts',(-1.90052930393596,1.,0.765772772593386));
#44132=CARTESIAN_POINT('Ctrl Pts',(-1.89436577771388,-1.,0.765913193856978));
#44133=CARTESIAN_POINT('Ctrl Pts',(-1.89436577771388,1.,0.765913193856978));
#44134=CARTESIAN_POINT('Ctrl Pts',(-1.88820926433409,-1.,0.766004837062091));
#44135=CARTESIAN_POINT('Ctrl Pts',(-1.88820926433409,1.,0.766004837062091));
#44136=CARTESIAN_POINT('Ctrl Pts',(-1.88206215302561,-1.,0.766047794851864));
#44137=CARTESIAN_POINT('Ctrl Pts',(-1.88206215302561,1.,0.766047794851864));
#44138=CARTESIAN_POINT('Ctrl Pts',(-1.87592888967883,-1.,0.766042837036744));
#44139=CARTESIAN_POINT('Ctrl Pts',(-1.87592888967883,1.,0.766042837036744));
#44140=CARTESIAN_POINT('Ctrl Pts',(-1.86981398314341,-1.,0.765990708546091));
#44141=CARTESIAN_POINT('Ctrl Pts',(-1.86981398314341,1.,0.765990708546091));
#44142=CARTESIAN_POINT('Ctrl Pts',(-1.86372027063312,-1.,0.765891519092547));
#44143=CARTESIAN_POINT('Ctrl Pts',(-1.86372027063312,1.,0.765891519092547));
#44144=CARTESIAN_POINT('Ctrl Pts',(-1.85764741390394,-1.,0.765744212909318));
#44145=CARTESIAN_POINT('Ctrl Pts',(-1.85764741390394,1.,0.765744212909318));
#44146=CARTESIAN_POINT('Ctrl Pts',(-1.85158945130063,-1.,0.765545710619062));
#44147=CARTESIAN_POINT('Ctrl Pts',(-1.85158945130063,1.,0.765545710619062));
#44148=CARTESIAN_POINT('Ctrl Pts',(-1.84553698875924,-1.,0.765291664862029));
#44149=CARTESIAN_POINT('Ctrl Pts',(-1.84553698875924,1.,0.765291664862029));
#44150=CARTESIAN_POINT('Ctrl Pts',(-1.83948181064835,-1.,0.764978057881737));
#44151=CARTESIAN_POINT('Ctrl Pts',(-1.83948181064835,1.,0.764978057881737));
#44152=CARTESIAN_POINT('Ctrl Pts',(-1.83342077227142,-1.,0.764602549687853));
#44153=CARTESIAN_POINT('Ctrl Pts',(-1.83342077227142,1.,0.764602549687853));
#44154=CARTESIAN_POINT('Ctrl Pts',(-1.82735991200065,-1.,0.764165902605995));
#44155=CARTESIAN_POINT('Ctrl Pts',(-1.82735991200065,1.,0.764165902605995));
#44156=CARTESIAN_POINT('Ctrl Pts',(-1.82131873145266,-1.,0.763673465462726));
#44157=CARTESIAN_POINT('Ctrl Pts',(-1.82131873145266,1.,0.763673465462726));
#44158=CARTESIAN_POINT('Ctrl Pts',(-1.8153211840553,-1.,0.763132003836634));
#44159=CARTESIAN_POINT('Ctrl Pts',(-1.8153211840553,1.,0.763132003836634));
#44160=CARTESIAN_POINT('Ctrl Pts',(-1.80938551463965,-1.,0.762546129463938));
#44161=CARTESIAN_POINT('Ctrl Pts',(-1.80938551463965,1.,0.762546129463938));
#44162=CARTESIAN_POINT('Ctrl Pts',(-1.80351583877342,-1.,0.761915336443547));
#44163=CARTESIAN_POINT('Ctrl Pts',(-1.80351583877342,1.,0.761915336443547));
#44164=CARTESIAN_POINT('Ctrl Pts',(-1.79768986997783,-1.,0.761229695230558));
#44165=CARTESIAN_POINT('Ctrl Pts',(-1.79768986997783,1.,0.761229695230558));
#44166=CARTESIAN_POINT('Ctrl Pts',(-1.7918581561088,-1.,0.760469555880749));
#44167=CARTESIAN_POINT('Ctrl Pts',(-1.7918581561088,1.,0.760469555880749));
#44168=CARTESIAN_POINT('Ctrl Pts',(-1.78596964884604,-1.,0.759614401110189));
#44169=CARTESIAN_POINT('Ctrl Pts',(-1.78596964884604,1.,0.759614401110189));
#44170=CARTESIAN_POINT('Ctrl Pts',(-1.77999411220945,-1.,0.758650626677518));
#44171=CARTESIAN_POINT('Ctrl Pts',(-1.77999411220945,1.,0.758650626677518));
#44172=CARTESIAN_POINT('Ctrl Pts',(-1.77394167108292,-1.,0.757578264077029));
#44173=CARTESIAN_POINT('Ctrl Pts',(-1.77394167108292,1.,0.757578264077029));
#44174=CARTESIAN_POINT('Ctrl Pts',(-1.76789396002998,-1.,0.75642189602781));
#44175=CARTESIAN_POINT('Ctrl Pts',(-1.76789396002998,1.,0.75642189602781));
#44176=CARTESIAN_POINT('Ctrl Pts',(-1.76197817240128,-1.,0.755220979974461));
#44177=CARTESIAN_POINT('Ctrl Pts',(-1.76197817240128,1.,0.755220979974461));
#44178=CARTESIAN_POINT('Ctrl Pts',(-1.75631083600019,-1.,0.754009254027829));
#44179=CARTESIAN_POINT('Ctrl Pts',(-1.75631083600019,1.,0.754009254027829));
#44180=CARTESIAN_POINT('Ctrl Pts',(-1.75095139468794,-1.,0.752797683531314));
#44181=CARTESIAN_POINT('Ctrl Pts',(-1.75095139468794,1.,0.752797683531314));
#44182=CARTESIAN_POINT('Ctrl Pts',(-1.74585086852502,-1.,0.751555614164482));
#44183=CARTESIAN_POINT('Ctrl Pts',(-1.74585086852502,1.,0.751555614164482));
#44184=CARTESIAN_POINT('Ctrl Pts',(-1.74080458267114,-1.,0.750193435981249));
#44185=CARTESIAN_POINT('Ctrl Pts',(-1.74080458267114,1.,0.750193435981249));
#44186=CARTESIAN_POINT('Ctrl Pts',(-1.7355035168033,-1.,0.74858246295687));
#44187=CARTESIAN_POINT('Ctrl Pts',(-1.7355035168033,1.,0.74858246295687));
#44188=CARTESIAN_POINT('Ctrl Pts',(-1.72958533647714,-1.,0.746574710097752));
#44189=CARTESIAN_POINT('Ctrl Pts',(-1.72958533647714,1.,0.746574710097752));
#44190=CARTESIAN_POINT('Ctrl Pts',(-1.72268229916769,-1.,0.744021445433093));
#44191=CARTESIAN_POINT('Ctrl Pts',(-1.72268229916769,1.,0.744021445433093));
#44192=CARTESIAN_POINT('Ctrl Pts',(-1.71447789751001,-1.,0.74079516202821));
#44193=CARTESIAN_POINT('Ctrl Pts',(-1.71447789751001,1.,0.74079516202821));
#44194=CARTESIAN_POINT('Ctrl Pts',(-1.70473309004249,-1.,0.736799665716932));
#44195=CARTESIAN_POINT('Ctrl Pts',(-1.70473309004249,1.,0.736799665716932));
#44196=CARTESIAN_POINT('Ctrl Pts',(-1.69326921972915,-1.,0.731963238685357));
#44197=CARTESIAN_POINT('Ctrl Pts',(-1.69326921972915,1.,0.731963238685357));
#44198=CARTESIAN_POINT('Ctrl Pts',(-1.67996158451922,-1.,0.726235967982445));
#44199=CARTESIAN_POINT('Ctrl Pts',(-1.67996158451922,1.,0.726235967982445));
#44200=CARTESIAN_POINT('Ctrl Pts',(-1.66472880551777,-1.,0.71958543378795));
#44201=CARTESIAN_POINT('Ctrl Pts',(-1.66472880551777,1.,0.71958543378795));
#44202=CARTESIAN_POINT('Ctrl Pts',(-1.64752408828442,-1.,0.711993139340447));
#44203=CARTESIAN_POINT('Ctrl Pts',(-1.64752408828442,1.,0.711993139340447));
#44204=CARTESIAN_POINT('Ctrl Pts',(-1.6321654166204,-1.,0.705159151977294));
#44205=CARTESIAN_POINT('Ctrl Pts',(-1.6321654166204,1.,0.705159151977294));
#44206=CARTESIAN_POINT('Ctrl Pts',(-1.61974673471117,-1.,0.699605146398837));
#44207=CARTESIAN_POINT('Ctrl Pts',(-1.61974673471117,1.,0.699605146398837));
#44208=CARTESIAN_POINT('Ctrl Pts',(-1.61106790957619,-1.,0.69571209787897));
#44209=CARTESIAN_POINT('Ctrl Pts',(-1.61106790957619,1.,0.69571209787897));
#44210=CARTESIAN_POINT('Ctrl Pts',(-1.60662857109684,-1.,0.693717979106305));
#44211=CARTESIAN_POINT('Ctrl Pts',(-1.60662857109684,1.,0.693717979106305));
#44212=CARTESIAN_POINT('',(-2.0698113262342,1.,0.7455743247944));
#44213=CARTESIAN_POINT('Ctrl Pts',(-2.0698113262342,1.,0.7455743247944));
#44214=CARTESIAN_POINT('Ctrl Pts',(-2.06854248895728,1.,0.745832791378367));
#44215=CARTESIAN_POINT('Ctrl Pts',(-2.06600523016815,1.,0.7463458715442));
#44216=CARTESIAN_POINT('Ctrl Pts',(-2.06220058927826,1.,0.747103932787919));
#44217=CARTESIAN_POINT('Ctrl Pts',(-2.05713023031006,1.,0.748091554183802));
#44218=CARTESIAN_POINT('Ctrl Pts',(-2.05079645592154,1.,0.749287468665046));
#44219=CARTESIAN_POINT('Ctrl Pts',(-2.04446689147979,1.,0.750444657875576));
#44220=CARTESIAN_POINT('Ctrl Pts',(-2.03814160092099,1.,0.751562963361115));
#44221=CARTESIAN_POINT('Ctrl Pts',(-2.03182068456221,1.,0.752642180487211));
#44222=CARTESIAN_POINT('Ctrl Pts',(-2.02550428623313,1.,0.753682061112768));
#44223=CARTESIAN_POINT('Ctrl Pts',(-2.01919259405809,1.,0.754682330722816));
#44224=CARTESIAN_POINT('Ctrl Pts',(-2.01288584328084,1.,0.755642704957865));
#44225=CARTESIAN_POINT('Ctrl Pts',(-2.0065843158773,1.,0.75656290464667));
#44226=CARTESIAN_POINT('Ctrl Pts',(-2.00028834739178,1.,0.757442676862724));
#44227=CARTESIAN_POINT('Ctrl Pts',(-1.99399831098817,1.,0.758281796766761));
#44228=CARTESIAN_POINT('Ctrl Pts',(-1.98771456680874,1.,0.759080037802488));
#44229=CARTESIAN_POINT('Ctrl Pts',(-1.98143741418172,1.,0.75983714745219));
#44230=CARTESIAN_POINT('Ctrl Pts',(-1.97516705321494,1.,0.760552825409757));
#44231=CARTESIAN_POINT('Ctrl Pts',(-1.96890351582499,1.,0.76122669048382));
#44232=CARTESIAN_POINT('Ctrl Pts',(-1.96264672744186,1.,0.761858300014423));
#44233=CARTESIAN_POINT('Ctrl Pts',(-1.95639665309869,1.,0.762447203806179));
#44234=CARTESIAN_POINT('Ctrl Pts',(-1.95015342590024,1.,0.762992990878769));
#44235=CARTESIAN_POINT('Ctrl Pts',(-1.9439174661764,1.,0.763495333538629));
#44236=CARTESIAN_POINT('Ctrl Pts',(-1.93768964875886,1.,0.763954049121458));
#44237=CARTESIAN_POINT('Ctrl Pts',(-1.93147105496382,1.,0.76436901067394));
#44238=CARTESIAN_POINT('Ctrl Pts',(-1.92526263537048,1.,0.764740025488211));
#44239=CARTESIAN_POINT('Ctrl Pts',(-1.91906491634196,1.,0.765066729667088));
#44240=CARTESIAN_POINT('Ctrl Pts',(-1.91287765805169,1.,0.765348465884722));
#44241=CARTESIAN_POINT('Ctrl Pts',(-1.90669961402356,1.,0.765584196937919));
#44242=CARTESIAN_POINT('Ctrl Pts',(-1.90052930393596,1.,0.765772772593386));
#44243=CARTESIAN_POINT('Ctrl Pts',(-1.89436577771388,1.,0.765913193856978));
#44244=CARTESIAN_POINT('Ctrl Pts',(-1.88820926433409,1.,0.766004837062091));
#44245=CARTESIAN_POINT('Ctrl Pts',(-1.88206215302561,1.,0.766047794851864));
#44246=CARTESIAN_POINT('Ctrl Pts',(-1.87592888967883,1.,0.766042837036744));
#44247=CARTESIAN_POINT('Ctrl Pts',(-1.86981398314341,1.,0.765990708546091));
#44248=CARTESIAN_POINT('Ctrl Pts',(-1.86372027063312,1.,0.765891519092547));
#44249=CARTESIAN_POINT('Ctrl Pts',(-1.85764741390394,1.,0.765744212909318));
#44250=CARTESIAN_POINT('Ctrl Pts',(-1.85158945130063,1.,0.765545710619062));
#44251=CARTESIAN_POINT('Ctrl Pts',(-1.84553698875924,1.,0.765291664862029));
#44252=CARTESIAN_POINT('Ctrl Pts',(-1.83948181064835,1.,0.764978057881737));
#44253=CARTESIAN_POINT('Ctrl Pts',(-1.83342077227142,1.,0.764602549687853));
#44254=CARTESIAN_POINT('Ctrl Pts',(-1.82735991200065,1.,0.764165902605995));
#44255=CARTESIAN_POINT('Ctrl Pts',(-1.82131873145266,1.,0.763673465462726));
#44256=CARTESIAN_POINT('Ctrl Pts',(-1.8153211840553,1.,0.763132003836634));
#44257=CARTESIAN_POINT('Ctrl Pts',(-1.80938551463965,1.,0.762546129463938));
#44258=CARTESIAN_POINT('Ctrl Pts',(-1.80351583877342,1.,0.761915336443547));
#44259=CARTESIAN_POINT('Ctrl Pts',(-1.79768986997783,1.,0.761229695230558));
#44260=CARTESIAN_POINT('Ctrl Pts',(-1.7918581561088,1.,0.760469555880749));
#44261=CARTESIAN_POINT('Ctrl Pts',(-1.78596964884604,1.,0.759614401110189));
#44262=CARTESIAN_POINT('Ctrl Pts',(-1.77999411220945,1.,0.758650626677518));
#44263=CARTESIAN_POINT('Ctrl Pts',(-1.77394167108292,1.,0.757578264077029));
#44264=CARTESIAN_POINT('Ctrl Pts',(-1.76789396002998,1.,0.75642189602781));
#44265=CARTESIAN_POINT('Ctrl Pts',(-1.76197817240128,1.,0.755220979974461));
#44266=CARTESIAN_POINT('Ctrl Pts',(-1.75631083600019,1.,0.754009254027829));
#44267=CARTESIAN_POINT('Ctrl Pts',(-1.75095139468794,1.,0.752797683531314));
#44268=CARTESIAN_POINT('Ctrl Pts',(-1.74585086852502,1.,0.751555614164482));
#44269=CARTESIAN_POINT('Ctrl Pts',(-1.74080458267114,1.,0.750193435981249));
#44270=CARTESIAN_POINT('Ctrl Pts',(-1.7355035168033,1.,0.74858246295687));
#44271=CARTESIAN_POINT('Ctrl Pts',(-1.72958533647714,1.,0.746574710097752));
#44272=CARTESIAN_POINT('Ctrl Pts',(-1.72268229916769,1.,0.744021445433093));
#44273=CARTESIAN_POINT('Ctrl Pts',(-1.71447789751001,1.,0.74079516202821));
#44274=CARTESIAN_POINT('Ctrl Pts',(-1.70473309004249,1.,0.736799665716932));
#44275=CARTESIAN_POINT('Ctrl Pts',(-1.69326921972915,1.,0.731963238685357));
#44276=CARTESIAN_POINT('Ctrl Pts',(-1.67996158451922,1.,0.726235967982445));
#44277=CARTESIAN_POINT('Ctrl Pts',(-1.66472880551777,1.,0.71958543378795));
#44278=CARTESIAN_POINT('Ctrl Pts',(-1.64752408828442,1.,0.711993139340447));
#44279=CARTESIAN_POINT('Ctrl Pts',(-1.6321654166204,1.,0.705159151977294));
#44280=CARTESIAN_POINT('Ctrl Pts',(-1.61974673471117,1.,0.699605146398837));
#44281=CARTESIAN_POINT('Ctrl Pts',(-1.61106790957619,1.,0.69571209787897));
#44282=CARTESIAN_POINT('Ctrl Pts',(-1.60662857109684,1.,0.693717979106305));
#44283=CARTESIAN_POINT('',(-2.0698113262342,0.,0.7455743247944));
#44284=CARTESIAN_POINT('Origin',(-2.11275013067528,0.,0.61342227326009));
#44285=CARTESIAN_POINT('',(-2.11275013067528,1.,0.61342227326009));
#44286=CARTESIAN_POINT('',(-2.0698113262342,1.,0.7455743247944));
#44287=CARTESIAN_POINT('',(-2.11275013067528,0.,0.61342227326009));
#44288=CARTESIAN_POINT('Ctrl Pts',(-1.7075470150345,-1.,0.383122945602004));
#44289=CARTESIAN_POINT('Ctrl Pts',(-1.7075470150345,1.,0.383122945602004));
#44290=CARTESIAN_POINT('Ctrl Pts',(-1.71231062891958,-1.,0.384119047315542));
#44291=CARTESIAN_POINT('Ctrl Pts',(-1.71231062891958,1.,0.384119047315542));
#44292=CARTESIAN_POINT('Ctrl Pts',(-1.72162022246158,-1.,0.38607079032701));
#44293=CARTESIAN_POINT('Ctrl Pts',(-1.72162022246158,1.,0.38607079032701));
#44294=CARTESIAN_POINT('Ctrl Pts',(-1.7349317097561,-1.,0.388877023509191));
#44295=CARTESIAN_POINT('Ctrl Pts',(-1.7349317097561,1.,0.388877023509191));
#44296=CARTESIAN_POINT('Ctrl Pts',(-1.75137405313962,-1.,0.392375812294307));
#44297=CARTESIAN_POINT('Ctrl Pts',(-1.75137405313962,1.,0.392375812294307));
#44298=CARTESIAN_POINT('Ctrl Pts',(-1.7697556004756,-1.,0.39634619612042));
#44299=CARTESIAN_POINT('Ctrl Pts',(-1.7697556004756,1.,0.39634619612042));
#44300=CARTESIAN_POINT('Ctrl Pts',(-1.78598826347533,-1.,0.39991940378308));
#44301=CARTESIAN_POINT('Ctrl Pts',(-1.78598826347533,1.,0.39991940378308));
#44302=CARTESIAN_POINT('Ctrl Pts',(-1.80012077176221,-1.,0.403107976170441));
#44303=CARTESIAN_POINT('Ctrl Pts',(-1.80012077176221,1.,0.403107976170441));
#44304=CARTESIAN_POINT('Ctrl Pts',(-1.81223801813988,-1.,0.405933518411838));
#44305=CARTESIAN_POINT('Ctrl Pts',(-1.81223801813988,1.,0.405933518411838));
#44306=CARTESIAN_POINT('Ctrl Pts',(-1.8224702267854,-1.,0.408428948108533));
#44307=CARTESIAN_POINT('Ctrl Pts',(-1.8224702267854,1.,0.408428948108533));
#44308=CARTESIAN_POINT('Ctrl Pts',(-1.83100408895216,-1.,0.410641256301675));
#44309=CARTESIAN_POINT('Ctrl Pts',(-1.83100408895216,1.,0.410641256301675));
#44310=CARTESIAN_POINT('Ctrl Pts',(-1.83808953475839,-1.,0.412633125322161));
#44311=CARTESIAN_POINT('Ctrl Pts',(-1.83808953475839,1.,0.412633125322161));
#44312=CARTESIAN_POINT('Ctrl Pts',(-1.8440575707371,-1.,0.41448743825434));
#44313=CARTESIAN_POINT('Ctrl Pts',(-1.8440575707371,1.,0.41448743825434));
#44314=CARTESIAN_POINT('Ctrl Pts',(-1.84929312929882,-1.,0.416300022038864));
#44315=CARTESIAN_POINT('Ctrl Pts',(-1.84929312929882,1.,0.416300022038864));
#44316=CARTESIAN_POINT('Ctrl Pts',(-1.85417632856234,-1.,0.418164129143534));
#44317=CARTESIAN_POINT('Ctrl Pts',(-1.85417632856234,1.,0.418164129143534));
#44318=CARTESIAN_POINT('Ctrl Pts',(-1.85903281096686,-1.,0.420157287975619));
#44319=CARTESIAN_POINT('Ctrl Pts',(-1.85903281096686,1.,0.420157287975619));
#44320=CARTESIAN_POINT('Ctrl Pts',(-1.86408083334028,-1.,0.422327307418275));
#44321=CARTESIAN_POINT('Ctrl Pts',(-1.86408083334028,1.,0.422327307418275));
#44322=CARTESIAN_POINT('Ctrl Pts',(-1.86937803944323,-1.,0.424678177291359));
#44323=CARTESIAN_POINT('Ctrl Pts',(-1.86937803944323,1.,0.424678177291359));
#44324=CARTESIAN_POINT('Ctrl Pts',(-1.87486989291484,-1.,0.427183828519102));
#44325=CARTESIAN_POINT('Ctrl Pts',(-1.87486989291484,1.,0.427183828519102));
#44326=CARTESIAN_POINT('Ctrl Pts',(-1.88044229001832,-1.,0.429803062482344));
#44327=CARTESIAN_POINT('Ctrl Pts',(-1.88044229001832,1.,0.429803062482344));
#44328=CARTESIAN_POINT('Ctrl Pts',(-1.88596913666793,-1.,0.432493038548748));
#44329=CARTESIAN_POINT('Ctrl Pts',(-1.88596913666793,1.,0.432493038548748));
#44330=CARTESIAN_POINT('Ctrl Pts',(-1.89136993975504,-1.,0.435225660963383));
#44331=CARTESIAN_POINT('Ctrl Pts',(-1.89136993975504,1.,0.435225660963383));
#44332=CARTESIAN_POINT('Ctrl Pts',(-1.89663648956466,-1.,0.437995003948244));
#44333=CARTESIAN_POINT('Ctrl Pts',(-1.89663648956466,1.,0.437995003948244));
#44334=CARTESIAN_POINT('Ctrl Pts',(-1.90180124389086,-1.,0.440807833704038));
#44335=CARTESIAN_POINT('Ctrl Pts',(-1.90180124389086,1.,0.440807833704038));
#44336=CARTESIAN_POINT('Ctrl Pts',(-1.90691756144898,-1.,0.44367755684915));
#44337=CARTESIAN_POINT('Ctrl Pts',(-1.90691756144898,1.,0.44367755684915));
#44338=CARTESIAN_POINT('Ctrl Pts',(-1.9120369998112,-1.,0.446617343485711));
#44339=CARTESIAN_POINT('Ctrl Pts',(-1.9120369998112,1.,0.446617343485711));
#44340=CARTESIAN_POINT('Ctrl Pts',(-1.91718342555755,-1.,0.449632260106662));
#44341=CARTESIAN_POINT('Ctrl Pts',(-1.91718342555755,1.,0.449632260106662));
#44342=CARTESIAN_POINT('Ctrl Pts',(-1.92235380648502,-1.,0.452719478359432));
#44343=CARTESIAN_POINT('Ctrl Pts',(-1.92235380648502,1.,0.452719478359432));
#44344=CARTESIAN_POINT('Ctrl Pts',(-1.92753067150476,-1.,0.455872005174371));
#44345=CARTESIAN_POINT('Ctrl Pts',(-1.92753067150476,1.,0.455872005174371));
#44346=CARTESIAN_POINT('Ctrl Pts',(-1.93269066517934,-1.,0.459081234547926));
#44347=CARTESIAN_POINT('Ctrl Pts',(-1.93269066517934,1.,0.459081234547926));
#44348=CARTESIAN_POINT('Ctrl Pts',(-1.93781486640821,-1.,0.462340031009056));
#44349=CARTESIAN_POINT('Ctrl Pts',(-1.93781486640821,1.,0.462340031009056));
#44350=CARTESIAN_POINT('Ctrl Pts',(-1.9428979419619,-1.,0.46564546202603));
#44351=CARTESIAN_POINT('Ctrl Pts',(-1.9428979419619,1.,0.46564546202603));
#44352=CARTESIAN_POINT('Ctrl Pts',(-1.94794381136514,-1.,0.468997482913135));
#44353=CARTESIAN_POINT('Ctrl Pts',(-1.94794381136514,1.,0.468997482913135));
#44354=CARTESIAN_POINT('Ctrl Pts',(-1.95296148278133,-1.,0.472397672264072));
#44355=CARTESIAN_POINT('Ctrl Pts',(-1.95296148278133,1.,0.472397672264072));
#44356=CARTESIAN_POINT('Ctrl Pts',(-1.95796111148177,-1.,0.475848034683176));
#44357=CARTESIAN_POINT('Ctrl Pts',(-1.95796111148177,1.,0.475848034683176));
#44358=CARTESIAN_POINT('Ctrl Pts',(-1.96294933055943,-1.,0.479349583074855));
#44359=CARTESIAN_POINT('Ctrl Pts',(-1.96294933055943,1.,0.479349583074855));
#44360=CARTESIAN_POINT('Ctrl Pts',(-1.96792703422362,-1.,0.48290166212069));
#44361=CARTESIAN_POINT('Ctrl Pts',(-1.96792703422362,1.,0.48290166212069));
#44362=CARTESIAN_POINT('Ctrl Pts',(-1.97289186263272,-1.,0.486502692907659));
#44363=CARTESIAN_POINT('Ctrl Pts',(-1.97289186263272,1.,0.486502692907659));
#44364=CARTESIAN_POINT('Ctrl Pts',(-1.97783973019229,-1.,0.490150627860952));
#44365=CARTESIAN_POINT('Ctrl Pts',(-1.97783973019229,1.,0.490150627860952));
#44366=CARTESIAN_POINT('Ctrl Pts',(-1.98276658761821,-1.,0.493843476541494));
#44367=CARTESIAN_POINT('Ctrl Pts',(-1.98276658761821,1.,0.493843476541494));
#44368=CARTESIAN_POINT('Ctrl Pts',(-1.98767044752932,-1.,0.497579909545574));
#44369=CARTESIAN_POINT('Ctrl Pts',(-1.98767044752932,1.,0.497579909545574));
#44370=CARTESIAN_POINT('Ctrl Pts',(-1.99255149126155,-1.,0.501359287727146));
#44371=CARTESIAN_POINT('Ctrl Pts',(-1.99255149126155,1.,0.501359287727146));
#44372=CARTESIAN_POINT('Ctrl Pts',(-1.99741107463572,-1.,0.505181361323026));
#44373=CARTESIAN_POINT('Ctrl Pts',(-1.99741107463572,1.,0.505181361323026));
#44374=CARTESIAN_POINT('Ctrl Pts',(-2.00225107134734,-1.,0.509046069886157));
#44375=CARTESIAN_POINT('Ctrl Pts',(-2.00225107134734,1.,0.509046069886157));
#44376=CARTESIAN_POINT('Ctrl Pts',(-2.00707309946949,-1.,0.512953306961792));
#44377=CARTESIAN_POINT('Ctrl Pts',(-2.00707309946949,1.,0.512953306961792));
#44378=CARTESIAN_POINT('Ctrl Pts',(-2.01187773939242,-1.,0.516902681728687));
#44379=CARTESIAN_POINT('Ctrl Pts',(-2.01187773939242,1.,0.516902681728687));
#44380=CARTESIAN_POINT('Ctrl Pts',(-2.01666477917286,-1.,0.52089359039937));
#44381=CARTESIAN_POINT('Ctrl Pts',(-2.01666477917286,1.,0.52089359039937));
#44382=CARTESIAN_POINT('Ctrl Pts',(-2.02143356304698,-1.,0.524925318333476));
#44383=CARTESIAN_POINT('Ctrl Pts',(-2.02143356304698,1.,0.524925318333476));
#44384=CARTESIAN_POINT('Ctrl Pts',(-2.0261832908329,-1.,0.528997127241914));
#44385=CARTESIAN_POINT('Ctrl Pts',(-2.0261832908329,1.,0.528997127241914));
#44386=CARTESIAN_POINT('Ctrl Pts',(-2.03091336214426,-1.,0.533108355132976));
#44387=CARTESIAN_POINT('Ctrl Pts',(-2.03091336214426,1.,0.533108355132976));
#44388=CARTESIAN_POINT('Ctrl Pts',(-2.03562362954037,-1.,0.537258489833262));
#44389=CARTESIAN_POINT('Ctrl Pts',(-2.03562362954037,1.,0.537258489833262));
#44390=CARTESIAN_POINT('Ctrl Pts',(-2.04031422690527,-1.,0.541447120615659));
#44391=CARTESIAN_POINT('Ctrl Pts',(-2.04031422690527,1.,0.541447120615659));
#44392=CARTESIAN_POINT('Ctrl Pts',(-2.04498544714588,-1.,0.54567390381743));
#44393=CARTESIAN_POINT('Ctrl Pts',(-2.04498544714588,1.,0.54567390381743));
#44394=CARTESIAN_POINT('Ctrl Pts',(-2.04963761077958,-1.,0.549938525150295));
#44395=CARTESIAN_POINT('Ctrl Pts',(-2.04963761077958,1.,0.549938525150295));
#44396=CARTESIAN_POINT('Ctrl Pts',(-2.05427091604413,-1.,0.554240657463906));
#44397=CARTESIAN_POINT('Ctrl Pts',(-2.05427091604413,1.,0.554240657463906));
#44398=CARTESIAN_POINT('Ctrl Pts',(-2.05888537756462,-1.,0.558579940185151));
#44399=CARTESIAN_POINT('Ctrl Pts',(-2.05888537756462,1.,0.558579940185151));
#44400=CARTESIAN_POINT('Ctrl Pts',(-2.06348090160589,-1.,0.562955993082261));
#44401=CARTESIAN_POINT('Ctrl Pts',(-2.06348090160589,1.,0.562955993082261));
#44402=CARTESIAN_POINT('Ctrl Pts',(-2.06805732997334,-1.,0.567368421181087));
#44403=CARTESIAN_POINT('Ctrl Pts',(-2.06805732997334,1.,0.567368421181087));
#44404=CARTESIAN_POINT('Ctrl Pts',(-2.07261449292824,-1.,0.571816823242603));
#44405=CARTESIAN_POINT('Ctrl Pts',(-2.07261449292824,1.,0.571816823242603));
#44406=CARTESIAN_POINT('Ctrl Pts',(-2.07715226767559,-1.,0.576300797416844));
#44407=CARTESIAN_POINT('Ctrl Pts',(-2.07715226767559,1.,0.576300797416844));
#44408=CARTESIAN_POINT('Ctrl Pts',(-2.08167059018418,-1.,0.580819952108063));
#44409=CARTESIAN_POINT('Ctrl Pts',(-2.08167059018418,1.,0.580819952108063));
#44410=CARTESIAN_POINT('Ctrl Pts',(-2.08616943727951,-1.,0.585373918991617));
#44411=CARTESIAN_POINT('Ctrl Pts',(-2.08616943727951,1.,0.585373918991617));
#44412=CARTESIAN_POINT('Ctrl Pts',(-2.09064881812129,-1.,0.589962365403406));
#44413=CARTESIAN_POINT('Ctrl Pts',(-2.09064881812129,1.,0.589962365403406));
#44414=CARTESIAN_POINT('Ctrl Pts',(-2.0951087622027,-1.,0.594585006052162));
#44415=CARTESIAN_POINT('Ctrl Pts',(-2.0951087622027,1.,0.594585006052162));
#44416=CARTESIAN_POINT('Ctrl Pts',(-2.0995493086477,-1.,0.599241616420533));
#44417=CARTESIAN_POINT('Ctrl Pts',(-2.0995493086477,1.,0.599241616420533));
#44418=CARTESIAN_POINT('Ctrl Pts',(-2.10397049886949,-1.,0.60393203073603));
#44419=CARTESIAN_POINT('Ctrl Pts',(-2.10397049886949,1.,0.60393203073603));
#44420=CARTESIAN_POINT('Ctrl Pts',(-2.1074919961518,-1.,0.607711315454876));
#44421=CARTESIAN_POINT('Ctrl Pts',(-2.1074919961518,1.,0.607711315454876));
#44422=CARTESIAN_POINT('Ctrl Pts',(-2.11012443807238,-1.,0.610560911689899));
#44423=CARTESIAN_POINT('Ctrl Pts',(-2.11012443807238,1.,0.610560911689899));
#44424=CARTESIAN_POINT('Ctrl Pts',(-2.11187554259986,-1.,0.6124673655618));
#44425=CARTESIAN_POINT('Ctrl Pts',(-2.11187554259986,1.,0.6124673655618));
#44426=CARTESIAN_POINT('Ctrl Pts',(-2.11275013067528,-1.,0.61342227326009));
#44427=CARTESIAN_POINT('Ctrl Pts',(-2.11275013067528,1.,0.61342227326009));
#44428=CARTESIAN_POINT('',(-1.7075470150345,1.,0.383122945602004));
#44429=CARTESIAN_POINT('Ctrl Pts',(-1.7075470150345,1.,0.383122945602004));
#44430=CARTESIAN_POINT('Ctrl Pts',(-1.71231062891958,1.,0.384119047315542));
#44431=CARTESIAN_POINT('Ctrl Pts',(-1.72162022246158,1.,0.38607079032701));
#44432=CARTESIAN_POINT('Ctrl Pts',(-1.7349317097561,1.,0.388877023509191));
#44433=CARTESIAN_POINT('Ctrl Pts',(-1.75137405313962,1.,0.392375812294307));
#44434=CARTESIAN_POINT('Ctrl Pts',(-1.7697556004756,1.,0.39634619612042));
#44435=CARTESIAN_POINT('Ctrl Pts',(-1.78598826347533,1.,0.39991940378308));
#44436=CARTESIAN_POINT('Ctrl Pts',(-1.80012077176221,1.,0.403107976170441));
#44437=CARTESIAN_POINT('Ctrl Pts',(-1.81223801813988,1.,0.405933518411838));
#44438=CARTESIAN_POINT('Ctrl Pts',(-1.8224702267854,1.,0.408428948108533));
#44439=CARTESIAN_POINT('Ctrl Pts',(-1.83100408895216,1.,0.410641256301675));
#44440=CARTESIAN_POINT('Ctrl Pts',(-1.83808953475839,1.,0.412633125322161));
#44441=CARTESIAN_POINT('Ctrl Pts',(-1.8440575707371,1.,0.41448743825434));
#44442=CARTESIAN_POINT('Ctrl Pts',(-1.84929312929882,1.,0.416300022038864));
#44443=CARTESIAN_POINT('Ctrl Pts',(-1.85417632856234,1.,0.418164129143534));
#44444=CARTESIAN_POINT('Ctrl Pts',(-1.85903281096686,1.,0.420157287975619));
#44445=CARTESIAN_POINT('Ctrl Pts',(-1.86408083334028,1.,0.422327307418275));
#44446=CARTESIAN_POINT('Ctrl Pts',(-1.86937803944323,1.,0.424678177291359));
#44447=CARTESIAN_POINT('Ctrl Pts',(-1.87486989291484,1.,0.427183828519102));
#44448=CARTESIAN_POINT('Ctrl Pts',(-1.88044229001832,1.,0.429803062482344));
#44449=CARTESIAN_POINT('Ctrl Pts',(-1.88596913666793,1.,0.432493038548748));
#44450=CARTESIAN_POINT('Ctrl Pts',(-1.89136993975504,1.,0.435225660963383));
#44451=CARTESIAN_POINT('Ctrl Pts',(-1.89663648956466,1.,0.437995003948244));
#44452=CARTESIAN_POINT('Ctrl Pts',(-1.90180124389086,1.,0.440807833704038));
#44453=CARTESIAN_POINT('Ctrl Pts',(-1.90691756144898,1.,0.44367755684915));
#44454=CARTESIAN_POINT('Ctrl Pts',(-1.9120369998112,1.,0.446617343485711));
#44455=CARTESIAN_POINT('Ctrl Pts',(-1.91718342555755,1.,0.449632260106662));
#44456=CARTESIAN_POINT('Ctrl Pts',(-1.92235380648502,1.,0.452719478359432));
#44457=CARTESIAN_POINT('Ctrl Pts',(-1.92753067150476,1.,0.455872005174371));
#44458=CARTESIAN_POINT('Ctrl Pts',(-1.93269066517934,1.,0.459081234547926));
#44459=CARTESIAN_POINT('Ctrl Pts',(-1.93781486640821,1.,0.462340031009056));
#44460=CARTESIAN_POINT('Ctrl Pts',(-1.9428979419619,1.,0.46564546202603));
#44461=CARTESIAN_POINT('Ctrl Pts',(-1.94794381136514,1.,0.468997482913135));
#44462=CARTESIAN_POINT('Ctrl Pts',(-1.95296148278133,1.,0.472397672264072));
#44463=CARTESIAN_POINT('Ctrl Pts',(-1.95796111148177,1.,0.475848034683176));
#44464=CARTESIAN_POINT('Ctrl Pts',(-1.96294933055943,1.,0.479349583074855));
#44465=CARTESIAN_POINT('Ctrl Pts',(-1.96792703422362,1.,0.48290166212069));
#44466=CARTESIAN_POINT('Ctrl Pts',(-1.97289186263272,1.,0.486502692907659));
#44467=CARTESIAN_POINT('Ctrl Pts',(-1.97783973019229,1.,0.490150627860952));
#44468=CARTESIAN_POINT('Ctrl Pts',(-1.98276658761821,1.,0.493843476541494));
#44469=CARTESIAN_POINT('Ctrl Pts',(-1.98767044752932,1.,0.497579909545574));
#44470=CARTESIAN_POINT('Ctrl Pts',(-1.99255149126155,1.,0.501359287727146));
#44471=CARTESIAN_POINT('Ctrl Pts',(-1.99741107463572,1.,0.505181361323026));
#44472=CARTESIAN_POINT('Ctrl Pts',(-2.00225107134734,1.,0.509046069886157));
#44473=CARTESIAN_POINT('Ctrl Pts',(-2.00707309946949,1.,0.512953306961792));
#44474=CARTESIAN_POINT('Ctrl Pts',(-2.01187773939242,1.,0.516902681728687));
#44475=CARTESIAN_POINT('Ctrl Pts',(-2.01666477917286,1.,0.52089359039937));
#44476=CARTESIAN_POINT('Ctrl Pts',(-2.02143356304698,1.,0.524925318333476));
#44477=CARTESIAN_POINT('Ctrl Pts',(-2.0261832908329,1.,0.528997127241914));
#44478=CARTESIAN_POINT('Ctrl Pts',(-2.03091336214426,1.,0.533108355132976));
#44479=CARTESIAN_POINT('Ctrl Pts',(-2.03562362954037,1.,0.537258489833262));
#44480=CARTESIAN_POINT('Ctrl Pts',(-2.04031422690527,1.,0.541447120615659));
#44481=CARTESIAN_POINT('Ctrl Pts',(-2.04498544714588,1.,0.54567390381743));
#44482=CARTESIAN_POINT('Ctrl Pts',(-2.04963761077958,1.,0.549938525150295));
#44483=CARTESIAN_POINT('Ctrl Pts',(-2.05427091604413,1.,0.554240657463906));
#44484=CARTESIAN_POINT('Ctrl Pts',(-2.05888537756462,1.,0.558579940185151));
#44485=CARTESIAN_POINT('Ctrl Pts',(-2.06348090160589,1.,0.562955993082261));
#44486=CARTESIAN_POINT('Ctrl Pts',(-2.06805732997334,1.,0.567368421181087));
#44487=CARTESIAN_POINT('Ctrl Pts',(-2.07261449292824,1.,0.571816823242603));
#44488=CARTESIAN_POINT('Ctrl Pts',(-2.07715226767559,1.,0.576300797416844));
#44489=CARTESIAN_POINT('Ctrl Pts',(-2.08167059018418,1.,0.580819952108063));
#44490=CARTESIAN_POINT('Ctrl Pts',(-2.08616943727951,1.,0.585373918991617));
#44491=CARTESIAN_POINT('Ctrl Pts',(-2.09064881812129,1.,0.589962365403406));
#44492=CARTESIAN_POINT('Ctrl Pts',(-2.0951087622027,1.,0.594585006052162));
#44493=CARTESIAN_POINT('Ctrl Pts',(-2.0995493086477,1.,0.599241616420533));
#44494=CARTESIAN_POINT('Ctrl Pts',(-2.10397049886949,1.,0.60393203073603));
#44495=CARTESIAN_POINT('Ctrl Pts',(-2.1074919961518,1.,0.607711315454876));
#44496=CARTESIAN_POINT('Ctrl Pts',(-2.11012443807238,1.,0.610560911689899));
#44497=CARTESIAN_POINT('Ctrl Pts',(-2.11187554259986,1.,0.6124673655618));
#44498=CARTESIAN_POINT('Ctrl Pts',(-2.11275013067528,1.,0.61342227326009));
#44499=CARTESIAN_POINT('',(-1.7075470150345,0.,0.383122945602003));
#44500=CARTESIAN_POINT('Origin',(0.,0.,0.));
#44501=CARTESIAN_POINT('',(-1.74236521665491,1.,0.163289472382896));
#44502=CARTESIAN_POINT('Origin',(0.,1.,0.));
#44503=CARTESIAN_POINT('',(-1.74236521665491,0.,0.163289472382896));
#44504=CARTESIAN_POINT('Ctrl Pts',(-2.19890268624765,-1.,0.069476445021958));
#44505=CARTESIAN_POINT('Ctrl Pts',(-2.19890268624765,1.,0.069476445021958));
#44506=CARTESIAN_POINT('Ctrl Pts',(-2.19777582085423,-1.,0.0701143536325489));
#44507=CARTESIAN_POINT('Ctrl Pts',(-2.19777582085423,1.,0.0701143536325489));
#44508=CARTESIAN_POINT('Ctrl Pts',(-2.19552129484002,-1.,0.0713863779526153));
#44509=CARTESIAN_POINT('Ctrl Pts',(-2.19552129484002,1.,0.0713863779526153));
#44510=CARTESIAN_POINT('Ctrl Pts',(-2.19213712013662,-1.,0.0732830357306724));
#44511=CARTESIAN_POINT('Ctrl Pts',(-2.19213712013662,1.,0.0732830357306724));
#44512=CARTESIAN_POINT('Ctrl Pts',(-2.1876201139953,-1.,0.0757891465836146));
#44513=CARTESIAN_POINT('Ctrl Pts',(-2.1876201139953,1.,0.0757891465836146));
#44514=CARTESIAN_POINT('Ctrl Pts',(-2.18196589448887,-1.,0.0788837727685241));
#44515=CARTESIAN_POINT('Ctrl Pts',(-2.18196589448887,1.,0.0788837727685241));
#44516=CARTESIAN_POINT('Ctrl Pts',(-2.176303712113,-1.,0.0819402680872764));
#44517=CARTESIAN_POINT('Ctrl Pts',(-2.176303712113,1.,0.0819402680872764));
#44518=CARTESIAN_POINT('Ctrl Pts',(-2.17063357870952,-1.,0.0849584620835371));
#44519=CARTESIAN_POINT('Ctrl Pts',(-2.17063357870952,1.,0.0849584620835371));
#44520=CARTESIAN_POINT('Ctrl Pts',(-2.16495552645014,-1.,0.0879381291386921));
#44521=CARTESIAN_POINT('Ctrl Pts',(-2.16495552645014,1.,0.0879381291386921));
#44522=CARTESIAN_POINT('Ctrl Pts',(-2.15926961544516,-1.,0.0908789888107264));
#44523=CARTESIAN_POINT('Ctrl Pts',(-2.15926961544516,1.,0.0908789888107264));
#44524=CARTESIAN_POINT('Ctrl Pts',(-2.1535759397817,-1.,0.0937807218867642));
#44525=CARTESIAN_POINT('Ctrl Pts',(-2.1535759397817,1.,0.0937807218867642));
#44526=CARTESIAN_POINT('Ctrl Pts',(-2.14787463531795,-1.,0.0966429852305457));
#44527=CARTESIAN_POINT('Ctrl Pts',(-2.14787463531795,1.,0.0966429852305457));
#44528=CARTESIAN_POINT('Ctrl Pts',(-2.14216588396025,-1.,0.0994654261990914));
#44529=CARTESIAN_POINT('Ctrl Pts',(-2.14216588396025,1.,0.0994654261990914));
#44530=CARTESIAN_POINT('Ctrl Pts',(-2.13644992667165,-1.,0.1022477005561));
#44531=CARTESIAN_POINT('Ctrl Pts',(-2.13644992667165,1.,0.1022477005561));
#44532=CARTESIAN_POINT('Ctrl Pts',(-2.13072704887293,-1.,0.104989479152739));
#44533=CARTESIAN_POINT('Ctrl Pts',(-2.13072704887293,1.,0.104989479152739));
#44534=CARTESIAN_POINT('Ctrl Pts',(-2.12499752307,-1.,0.10769043523109));
#44535=CARTESIAN_POINT('Ctrl Pts',(-2.12499752307,1.,0.10769043523109));
#44536=CARTESIAN_POINT('Ctrl Pts',(-2.11926155590865,-1.,0.110350236135025));
#44537=CARTESIAN_POINT('Ctrl Pts',(-2.11926155590865,1.,0.110350236135025));
#44538=CARTESIAN_POINT('Ctrl Pts',(-2.11351924490306,-1.,0.112968534419737));
#44539=CARTESIAN_POINT('Ctrl Pts',(-2.11351924490306,1.,0.112968534419737));
#44540=CARTESIAN_POINT('Ctrl Pts',(-2.10777050261309,-1.,0.115544957687926));
#44541=CARTESIAN_POINT('Ctrl Pts',(-2.10777050261309,1.,0.115544957687926));
#44542=CARTESIAN_POINT('Ctrl Pts',(-2.102015121329,-1.,0.118079107988355));
#44543=CARTESIAN_POINT('Ctrl Pts',(-2.102015121329,1.,0.118079107988355));
#44544=CARTESIAN_POINT('Ctrl Pts',(-2.0962529286773,-1.,0.120570567965122));
#44545=CARTESIAN_POINT('Ctrl Pts',(-2.0962529286773,1.,0.120570567965122));
#44546=CARTESIAN_POINT('Ctrl Pts',(-2.09048392424825,-1.,0.123018905621083));
#44547=CARTESIAN_POINT('Ctrl Pts',(-2.09048392424825,1.,0.123018905621083));
#44548=CARTESIAN_POINT('Ctrl Pts',(-2.08470840653643,-1.,0.125423679412061));
#44549=CARTESIAN_POINT('Ctrl Pts',(-2.08470840653643,1.,0.125423679412061));
#44550=CARTESIAN_POINT('Ctrl Pts',(-2.07892715110987,-1.,0.12778444527612));
#44551=CARTESIAN_POINT('Ctrl Pts',(-2.07892715110987,1.,0.12778444527612));
#44552=CARTESIAN_POINT('Ctrl Pts',(-2.07314114713063,-1.,0.130100748328403));
#44553=CARTESIAN_POINT('Ctrl Pts',(-2.07314114713063,1.,0.130100748328403));
#44554=CARTESIAN_POINT('Ctrl Pts',(-2.06735123910326,-1.,0.13237211154771));
#44555=CARTESIAN_POINT('Ctrl Pts',(-2.06735123910326,1.,0.13237211154771));
#44556=CARTESIAN_POINT('Ctrl Pts',(-2.06155781517842,-1.,0.134598026192106));
#44557=CARTESIAN_POINT('Ctrl Pts',(-2.06155781517842,1.,0.134598026192106));
#44558=CARTESIAN_POINT('Ctrl Pts',(-2.05576044414264,-1.,0.136777941218043));
#44559=CARTESIAN_POINT('Ctrl Pts',(-2.05576044414264,1.,0.136777941218043));
#44560=CARTESIAN_POINT('Ctrl Pts',(-2.04995762001328,-1.,0.138911255368966));
#44561=CARTESIAN_POINT('Ctrl Pts',(-2.04995762001328,1.,0.138911255368966));
#44562=CARTESIAN_POINT('Ctrl Pts',(-2.04414757947916,-1.,0.140997332152546));
#44563=CARTESIAN_POINT('Ctrl Pts',(-2.04414757947916,1.,0.140997332152546));
#44564=CARTESIAN_POINT('Ctrl Pts',(-2.03832911025912,-1.,0.143035515058209));
#44565=CARTESIAN_POINT('Ctrl Pts',(-2.03832911025912,1.,0.143035515058209));
#44566=CARTESIAN_POINT('Ctrl Pts',(-2.03250223739942,-1.,0.145025140186057));
#44567=CARTESIAN_POINT('Ctrl Pts',(-2.03250223739942,1.,0.145025140186057));
#44568=CARTESIAN_POINT('Ctrl Pts',(-2.02666926182017,-1.,0.146965557332583));
#44569=CARTESIAN_POINT('Ctrl Pts',(-2.02666926182017,1.,0.146965557332583));
#44570=CARTESIAN_POINT('Ctrl Pts',(-2.02083464969894,-1.,0.148856124775337));
#44571=CARTESIAN_POINT('Ctrl Pts',(-2.02083464969894,1.,0.148856124775337));
#44572=CARTESIAN_POINT('Ctrl Pts',(-2.01500291940238,-1.,0.150696157673078));
#44573=CARTESIAN_POINT('Ctrl Pts',(-2.01500291940238,1.,0.150696157673078));
#44574=CARTESIAN_POINT('Ctrl Pts',(-2.00917680318424,-1.,0.15248488362145));
#44575=CARTESIAN_POINT('Ctrl Pts',(-2.00917680318424,1.,0.15248488362145));
#44576=CARTESIAN_POINT('Ctrl Pts',(-2.00335565310543,-1.,0.154221403049722));
#44577=CARTESIAN_POINT('Ctrl Pts',(-2.00335565310543,1.,0.154221403049722));
#44578=CARTESIAN_POINT('Ctrl Pts',(-1.99753284771497,-1.,0.155904629548783));
#44579=CARTESIAN_POINT('Ctrl Pts',(-1.99753284771497,1.,0.155904629548783));
#44580=CARTESIAN_POINT('Ctrl Pts',(-1.99169810931908,-1.,0.157533331459227));
#44581=CARTESIAN_POINT('Ctrl Pts',(-1.99169810931908,1.,0.157533331459227));
#44582=CARTESIAN_POINT('Ctrl Pts',(-1.98584238283292,-1.,0.159106226437299));
#44583=CARTESIAN_POINT('Ctrl Pts',(-1.98584238283292,1.,0.159106226437299));
#44584=CARTESIAN_POINT('Ctrl Pts',(-1.97996195437559,-1.,0.160622060784611));
#44585=CARTESIAN_POINT('Ctrl Pts',(-1.97996195437559,1.,0.160622060784611));
#44586=CARTESIAN_POINT('Ctrl Pts',(-1.97406280235188,-1.,0.162079693556288));
#44587=CARTESIAN_POINT('Ctrl Pts',(-1.97406280235188,1.,0.162079693556288));
#44588=CARTESIAN_POINT('Ctrl Pts',(-1.96816512677967,-1.,0.163478185457734));
#44589=CARTESIAN_POINT('Ctrl Pts',(-1.96816512677967,1.,0.163478185457734));
#44590=CARTESIAN_POINT('Ctrl Pts',(-1.96229379940136,-1.,0.164816568920269));
#44591=CARTESIAN_POINT('Ctrl Pts',(-1.96229379940136,1.,0.164816568920269));
#44592=CARTESIAN_POINT('Ctrl Pts',(-1.9564675971873,-1.,0.166093592002812));
#44593=CARTESIAN_POINT('Ctrl Pts',(-1.9564675971873,1.,0.166093592002812));
#44594=CARTESIAN_POINT('Ctrl Pts',(-1.95069027794294,-1.,0.167307501784475));
#44595=CARTESIAN_POINT('Ctrl Pts',(-1.95069027794294,1.,0.167307501784475));
#44596=CARTESIAN_POINT('Ctrl Pts',(-1.94493757756931,-1.,0.168455741607556));
#44597=CARTESIAN_POINT('Ctrl Pts',(-1.94493757756931,1.,0.168455741607556));
#44598=CARTESIAN_POINT('Ctrl Pts',(-1.93915639211581,-1.,0.169534904817491));
#44599=CARTESIAN_POINT('Ctrl Pts',(-1.93915639211581,1.,0.169534904817491));
#44600=CARTESIAN_POINT('Ctrl Pts',(-1.93329183155539,-1.,0.170541253116201));
#44601=CARTESIAN_POINT('Ctrl Pts',(-1.93329183155539,1.,0.170541253116201));
#44602=CARTESIAN_POINT('Ctrl Pts',(-1.92731093582036,-1.,0.171471191532988));
#44603=CARTESIAN_POINT('Ctrl Pts',(-1.92731093582036,1.,0.171471191532988));
#44604=CARTESIAN_POINT('Ctrl Pts',(-1.9212233439798,-1.,0.172321621259514));
#44605=CARTESIAN_POINT('Ctrl Pts',(-1.9212233439798,1.,0.172321621259514));
#44606=CARTESIAN_POINT('Ctrl Pts',(-1.91511429159527,-1.,0.173090695383496));
#44607=CARTESIAN_POINT('Ctrl Pts',(-1.91511429159527,1.,0.173090695383496));
#44608=CARTESIAN_POINT('Ctrl Pts',(-1.90911693975267,-1.,0.173776635257817));
#44609=CARTESIAN_POINT('Ctrl Pts',(-1.90911693975267,1.,0.173776635257817));
#44610=CARTESIAN_POINT('Ctrl Pts',(-1.90335253862834,-1.,0.174375518661085));
#44611=CARTESIAN_POINT('Ctrl Pts',(-1.90335253862834,1.,0.174375518661085));
#44612=CARTESIAN_POINT('Ctrl Pts',(-1.89788101117132,-1.,0.174879405091263));
#44613=CARTESIAN_POINT('Ctrl Pts',(-1.89788101117132,1.,0.174879405091263));
#44614=CARTESIAN_POINT('Ctrl Pts',(-1.892646301985,-1.,0.175274276190844));
#44615=CARTESIAN_POINT('Ctrl Pts',(-1.892646301985,1.,0.175274276190844));
#44616=CARTESIAN_POINT('Ctrl Pts',(-1.88742606273259,-1.,0.175538155840648));
#44617=CARTESIAN_POINT('Ctrl Pts',(-1.88742606273259,1.,0.175538155840648));
#44618=CARTESIAN_POINT('Ctrl Pts',(-1.88188663145367,-1.,0.175644148889698));
#44619=CARTESIAN_POINT('Ctrl Pts',(-1.88188663145367,1.,0.175644148889698));
#44620=CARTESIAN_POINT('Ctrl Pts',(-1.87563767773588,-1.,0.175563480746485));
#44621=CARTESIAN_POINT('Ctrl Pts',(-1.87563767773588,1.,0.175563480746485));
#44622=CARTESIAN_POINT('Ctrl Pts',(-1.86828349694799,-1.,0.175268337590758));
#44623=CARTESIAN_POINT('Ctrl Pts',(-1.86828349694799,1.,0.175268337590758));
#44624=CARTESIAN_POINT('Ctrl Pts',(-1.85948367088837,-1.,0.17473525927603));
#44625=CARTESIAN_POINT('Ctrl Pts',(-1.85948367088837,1.,0.17473525927603));
#44626=CARTESIAN_POINT('Ctrl Pts',(-1.8489811319852,-1.,0.173946627587731));
#44627=CARTESIAN_POINT('Ctrl Pts',(-1.8489811319852,1.,0.173946627587731));
#44628=CARTESIAN_POINT('Ctrl Pts',(-1.83658380527692,-1.,0.1728894428919));
#44629=CARTESIAN_POINT('Ctrl Pts',(-1.83658380527692,1.,0.1728894428919));
#44630=CARTESIAN_POINT('Ctrl Pts',(-1.82215766811545,-1.,0.171554770204119));
#44631=CARTESIAN_POINT('Ctrl Pts',(-1.82215766811545,1.,0.171554770204119));
#44632=CARTESIAN_POINT('Ctrl Pts',(-1.80561530629706,-1.,0.169936923904608));
#44633=CARTESIAN_POINT('Ctrl Pts',(-1.80561530629706,1.,0.169936923904608));
#44634=CARTESIAN_POINT('Ctrl Pts',(-1.7869064998507,-1.,0.168032772805197));
#44635=CARTESIAN_POINT('Ctrl Pts',(-1.7869064998507,1.,0.168032772805197));
#44636=CARTESIAN_POINT('Ctrl Pts',(-1.77018771684844,-1.,0.1662793551464));
#44637=CARTESIAN_POINT('Ctrl Pts',(-1.77018771684844,1.,0.1662793551464));
#44638=CARTESIAN_POINT('Ctrl Pts',(-1.75666056638427,-1.,0.164834765707158));
#44639=CARTESIAN_POINT('Ctrl Pts',(-1.75666056638427,1.,0.164834765707158));
#44640=CARTESIAN_POINT('Ctrl Pts',(-1.7472034950333,-1.,0.163814161002002));
#44641=CARTESIAN_POINT('Ctrl Pts',(-1.7472034950333,1.,0.163814161002002));
#44642=CARTESIAN_POINT('Ctrl Pts',(-1.74236521665491,-1.,0.163289472382896));
#44643=CARTESIAN_POINT('Ctrl Pts',(-1.74236521665491,1.,0.163289472382896));
#44644=CARTESIAN_POINT('',(-2.19890268624765,1.,0.069476445021958));
#44645=CARTESIAN_POINT('Ctrl Pts',(-2.19890268624765,1.,0.069476445021958));
#44646=CARTESIAN_POINT('Ctrl Pts',(-2.19777582085423,1.,0.0701143536325489));
#44647=CARTESIAN_POINT('Ctrl Pts',(-2.19552129484002,1.,0.0713863779526153));
#44648=CARTESIAN_POINT('Ctrl Pts',(-2.19213712013662,1.,0.0732830357306724));
#44649=CARTESIAN_POINT('Ctrl Pts',(-2.1876201139953,1.,0.0757891465836146));
#44650=CARTESIAN_POINT('Ctrl Pts',(-2.18196589448887,1.,0.0788837727685241));
#44651=CARTESIAN_POINT('Ctrl Pts',(-2.176303712113,1.,0.0819402680872764));
#44652=CARTESIAN_POINT('Ctrl Pts',(-2.17063357870952,1.,0.0849584620835371));
#44653=CARTESIAN_POINT('Ctrl Pts',(-2.16495552645014,1.,0.0879381291386921));
#44654=CARTESIAN_POINT('Ctrl Pts',(-2.15926961544516,1.,0.0908789888107264));
#44655=CARTESIAN_POINT('Ctrl Pts',(-2.1535759397817,1.,0.0937807218867642));
#44656=CARTESIAN_POINT('Ctrl Pts',(-2.14787463531795,1.,0.0966429852305457));
#44657=CARTESIAN_POINT('Ctrl Pts',(-2.14216588396025,1.,0.0994654261990914));
#44658=CARTESIAN_POINT('Ctrl Pts',(-2.13644992667165,1.,0.1022477005561));
#44659=CARTESIAN_POINT('Ctrl Pts',(-2.13072704887293,1.,0.104989479152739));
#44660=CARTESIAN_POINT('Ctrl Pts',(-2.12499752307,1.,0.10769043523109));
#44661=CARTESIAN_POINT('Ctrl Pts',(-2.11926155590865,1.,0.110350236135025));
#44662=CARTESIAN_POINT('Ctrl Pts',(-2.11351924490306,1.,0.112968534419737));
#44663=CARTESIAN_POINT('Ctrl Pts',(-2.10777050261309,1.,0.115544957687926));
#44664=CARTESIAN_POINT('Ctrl Pts',(-2.102015121329,1.,0.118079107988355));
#44665=CARTESIAN_POINT('Ctrl Pts',(-2.0962529286773,1.,0.120570567965122));
#44666=CARTESIAN_POINT('Ctrl Pts',(-2.09048392424825,1.,0.123018905621083));
#44667=CARTESIAN_POINT('Ctrl Pts',(-2.08470840653643,1.,0.125423679412061));
#44668=CARTESIAN_POINT('Ctrl Pts',(-2.07892715110987,1.,0.12778444527612));
#44669=CARTESIAN_POINT('Ctrl Pts',(-2.07314114713063,1.,0.130100748328403));
#44670=CARTESIAN_POINT('Ctrl Pts',(-2.06735123910326,1.,0.13237211154771));
#44671=CARTESIAN_POINT('Ctrl Pts',(-2.06155781517842,1.,0.134598026192106));
#44672=CARTESIAN_POINT('Ctrl Pts',(-2.05576044414264,1.,0.136777941218043));
#44673=CARTESIAN_POINT('Ctrl Pts',(-2.04995762001328,1.,0.138911255368966));
#44674=CARTESIAN_POINT('Ctrl Pts',(-2.04414757947916,1.,0.140997332152546));
#44675=CARTESIAN_POINT('Ctrl Pts',(-2.03832911025912,1.,0.143035515058209));
#44676=CARTESIAN_POINT('Ctrl Pts',(-2.03250223739942,1.,0.145025140186057));
#44677=CARTESIAN_POINT('Ctrl Pts',(-2.02666926182017,1.,0.146965557332583));
#44678=CARTESIAN_POINT('Ctrl Pts',(-2.02083464969894,1.,0.148856124775337));
#44679=CARTESIAN_POINT('Ctrl Pts',(-2.01500291940238,1.,0.150696157673078));
#44680=CARTESIAN_POINT('Ctrl Pts',(-2.00917680318424,1.,0.15248488362145));
#44681=CARTESIAN_POINT('Ctrl Pts',(-2.00335565310543,1.,0.154221403049722));
#44682=CARTESIAN_POINT('Ctrl Pts',(-1.99753284771497,1.,0.155904629548783));
#44683=CARTESIAN_POINT('Ctrl Pts',(-1.99169810931908,1.,0.157533331459227));
#44684=CARTESIAN_POINT('Ctrl Pts',(-1.98584238283292,1.,0.159106226437299));
#44685=CARTESIAN_POINT('Ctrl Pts',(-1.97996195437559,1.,0.160622060784611));
#44686=CARTESIAN_POINT('Ctrl Pts',(-1.97406280235188,1.,0.162079693556288));
#44687=CARTESIAN_POINT('Ctrl Pts',(-1.96816512677967,1.,0.163478185457734));
#44688=CARTESIAN_POINT('Ctrl Pts',(-1.96229379940136,1.,0.164816568920269));
#44689=CARTESIAN_POINT('Ctrl Pts',(-1.9564675971873,1.,0.166093592002812));
#44690=CARTESIAN_POINT('Ctrl Pts',(-1.95069027794294,1.,0.167307501784475));
#44691=CARTESIAN_POINT('Ctrl Pts',(-1.94493757756931,1.,0.168455741607556));
#44692=CARTESIAN_POINT('Ctrl Pts',(-1.93915639211581,1.,0.169534904817491));
#44693=CARTESIAN_POINT('Ctrl Pts',(-1.93329183155539,1.,0.170541253116201));
#44694=CARTESIAN_POINT('Ctrl Pts',(-1.92731093582036,1.,0.171471191532988));
#44695=CARTESIAN_POINT('Ctrl Pts',(-1.9212233439798,1.,0.172321621259514));
#44696=CARTESIAN_POINT('Ctrl Pts',(-1.91511429159527,1.,0.173090695383496));
#44697=CARTESIAN_POINT('Ctrl Pts',(-1.90911693975267,1.,0.173776635257817));
#44698=CARTESIAN_POINT('Ctrl Pts',(-1.90335253862834,1.,0.174375518661085));
#44699=CARTESIAN_POINT('Ctrl Pts',(-1.89788101117132,1.,0.174879405091263));
#44700=CARTESIAN_POINT('Ctrl Pts',(-1.892646301985,1.,0.175274276190844));
#44701=CARTESIAN_POINT('Ctrl Pts',(-1.88742606273259,1.,0.175538155840648));
#44702=CARTESIAN_POINT('Ctrl Pts',(-1.88188663145367,1.,0.175644148889698));
#44703=CARTESIAN_POINT('Ctrl Pts',(-1.87563767773588,1.,0.175563480746485));
#44704=CARTESIAN_POINT('Ctrl Pts',(-1.86828349694799,1.,0.175268337590758));
#44705=CARTESIAN_POINT('Ctrl Pts',(-1.85948367088837,1.,0.17473525927603));
#44706=CARTESIAN_POINT('Ctrl Pts',(-1.8489811319852,1.,0.173946627587731));
#44707=CARTESIAN_POINT('Ctrl Pts',(-1.83658380527692,1.,0.1728894428919));
#44708=CARTESIAN_POINT('Ctrl Pts',(-1.82215766811545,1.,0.171554770204119));
#44709=CARTESIAN_POINT('Ctrl Pts',(-1.80561530629706,1.,0.169936923904608));
#44710=CARTESIAN_POINT('Ctrl Pts',(-1.7869064998507,1.,0.168032772805197));
#44711=CARTESIAN_POINT('Ctrl Pts',(-1.77018771684844,1.,0.1662793551464));
#44712=CARTESIAN_POINT('Ctrl Pts',(-1.75666056638427,1.,0.164834765707158));
#44713=CARTESIAN_POINT('Ctrl Pts',(-1.7472034950333,1.,0.163814161002002));
#44714=CARTESIAN_POINT('Ctrl Pts',(-1.74236521665491,1.,0.163289472382896));
#44715=CARTESIAN_POINT('',(-2.19890268624765,0.,0.069476445021958));
#44716=CARTESIAN_POINT('Origin',(-2.19890268624765,0.,-0.0694764450219585));
#44717=CARTESIAN_POINT('',(-2.19890268624765,1.,-0.0694764450219585));
#44718=CARTESIAN_POINT('',(-2.19890268624765,1.,0.069476445021958));
#44719=CARTESIAN_POINT('',(-2.19890268624765,0.,-0.0694764450219585));
#44720=CARTESIAN_POINT('Ctrl Pts',(-1.74236521665491,-1.,-0.163289472382896));
#44721=CARTESIAN_POINT('Ctrl Pts',(-1.74236521665491,1.,-0.163289472382896));
#44722=CARTESIAN_POINT('Ctrl Pts',(-1.74720349503904,-1.,-0.163814161002474));
#44723=CARTESIAN_POINT('Ctrl Pts',(-1.74720349503904,1.,-0.163814161002474));
#44724=CARTESIAN_POINT('Ctrl Pts',(-1.75666056640041,-1.,-0.164834765708484));
#44725=CARTESIAN_POINT('Ctrl Pts',(-1.75666056640041,1.,-0.164834765708484));
#44726=CARTESIAN_POINT('Ctrl Pts',(-1.77018771687692,-1.,-0.166279355148738));
#44727=CARTESIAN_POINT('Ctrl Pts',(-1.77018771687692,1.,-0.166279355148738));
#44728=CARTESIAN_POINT('Ctrl Pts',(-1.78690649988931,-1.,-0.16803277280837));
#44729=CARTESIAN_POINT('Ctrl Pts',(-1.78690649988931,1.,-0.16803277280837));
#44730=CARTESIAN_POINT('Ctrl Pts',(-1.80561530633924,-1.,-0.169936923908078));
#44731=CARTESIAN_POINT('Ctrl Pts',(-1.80561530633924,1.,-0.169936923908078));
#44732=CARTESIAN_POINT('Ctrl Pts',(-1.82215766815414,-1.,-0.171554770207306));
#44733=CARTESIAN_POINT('Ctrl Pts',(-1.82215766815414,1.,-0.171554770207306));
#44734=CARTESIAN_POINT('Ctrl Pts',(-1.83658380530747,-1.,-0.17288944289442));
#44735=CARTESIAN_POINT('Ctrl Pts',(-1.83658380530747,1.,-0.17288944289442));
#44736=CARTESIAN_POINT('Ctrl Pts',(-1.84898113200543,-1.,-0.173946627589401));
#44737=CARTESIAN_POINT('Ctrl Pts',(-1.84898113200543,1.,-0.173946627589401));
#44738=CARTESIAN_POINT('Ctrl Pts',(-1.85948367089838,-1.,-0.174735259276856));
#44739=CARTESIAN_POINT('Ctrl Pts',(-1.85948367089838,1.,-0.174735259276856));
#44740=CARTESIAN_POINT('Ctrl Pts',(-1.86828349694972,-1.,-0.175268337590901));
#44741=CARTESIAN_POINT('Ctrl Pts',(-1.86828349694972,1.,-0.175268337590901));
#44742=CARTESIAN_POINT('Ctrl Pts',(-1.87563767773249,-1.,-0.175563480746205));
#44743=CARTESIAN_POINT('Ctrl Pts',(-1.87563767773249,1.,-0.175563480746205));
#44744=CARTESIAN_POINT('Ctrl Pts',(-1.88188663144846,-1.,-0.175644148889271));
#44745=CARTESIAN_POINT('Ctrl Pts',(-1.88188663144846,1.,-0.175644148889271));
#44746=CARTESIAN_POINT('Ctrl Pts',(-1.88742606272818,-1.,-0.175538155840286));
#44747=CARTESIAN_POINT('Ctrl Pts',(-1.88742606272818,1.,-0.175538155840286));
#44748=CARTESIAN_POINT('Ctrl Pts',(-1.89264630198279,-1.,-0.175274276190664));
#44749=CARTESIAN_POINT('Ctrl Pts',(-1.89264630198279,1.,-0.175274276190664));
#44750=CARTESIAN_POINT('Ctrl Pts',(-1.89788101117148,-1.,-0.174879405091277));
#44751=CARTESIAN_POINT('Ctrl Pts',(-1.89788101117148,1.,-0.174879405091277));
#44752=CARTESIAN_POINT('Ctrl Pts',(-1.90335253863003,-1.,-0.174375518661222));
#44753=CARTESIAN_POINT('Ctrl Pts',(-1.90335253863003,1.,-0.174375518661222));
#44754=CARTESIAN_POINT('Ctrl Pts',(-1.90911693975475,-1.,-0.173776635257984));
#44755=CARTESIAN_POINT('Ctrl Pts',(-1.90911693975475,1.,-0.173776635257984));
#44756=CARTESIAN_POINT('Ctrl Pts',(-1.91511429159681,-1.,-0.173090695383619));
#44757=CARTESIAN_POINT('Ctrl Pts',(-1.91511429159681,1.,-0.173090695383619));
#44758=CARTESIAN_POINT('Ctrl Pts',(-1.92122334398034,-1.,-0.172321621259557));
#44759=CARTESIAN_POINT('Ctrl Pts',(-1.92122334398034,1.,-0.172321621259557));
#44760=CARTESIAN_POINT('Ctrl Pts',(-1.92731093582,-1.,-0.17147119153296));
#44761=CARTESIAN_POINT('Ctrl Pts',(-1.92731093582,1.,-0.17147119153296));
#44762=CARTESIAN_POINT('Ctrl Pts',(-1.93329183155455,-1.,-0.170541253116136));
#44763=CARTESIAN_POINT('Ctrl Pts',(-1.93329183155455,1.,-0.170541253116136));
#44764=CARTESIAN_POINT('Ctrl Pts',(-1.93915639211497,-1.,-0.169534904817425));
#44765=CARTESIAN_POINT('Ctrl Pts',(-1.93915639211497,1.,-0.169534904817425));
#44766=CARTESIAN_POINT('Ctrl Pts',(-1.94493757756879,-1.,-0.168455741607516));
#44767=CARTESIAN_POINT('Ctrl Pts',(-1.94493757756879,1.,-0.168455741607516));
#44768=CARTESIAN_POINT('Ctrl Pts',(-1.95069027794286,-1.,-0.167307501784469));
#44769=CARTESIAN_POINT('Ctrl Pts',(-1.95069027794286,1.,-0.167307501784469));
#44770=CARTESIAN_POINT('Ctrl Pts',(-1.95646759718755,-1.,-0.166093592002833));
#44771=CARTESIAN_POINT('Ctrl Pts',(-1.95646759718755,1.,-0.166093592002833));
#44772=CARTESIAN_POINT('Ctrl Pts',(-1.96229379940174,-1.,-0.1648165689203));
#44773=CARTESIAN_POINT('Ctrl Pts',(-1.96229379940174,1.,-0.1648165689203));
#44774=CARTESIAN_POINT('Ctrl Pts',(-1.96816512678,-1.,-0.16347818545776));
#44775=CARTESIAN_POINT('Ctrl Pts',(-1.96816512678,1.,-0.16347818545776));
#44776=CARTESIAN_POINT('Ctrl Pts',(-1.97406280235204,-1.,-0.162079693556302));
#44777=CARTESIAN_POINT('Ctrl Pts',(-1.97406280235204,1.,-0.162079693556302));
#44778=CARTESIAN_POINT('Ctrl Pts',(-1.97996195437557,-1.,-0.16062206078461));
#44779=CARTESIAN_POINT('Ctrl Pts',(-1.97996195437557,1.,-0.16062206078461));
#44780=CARTESIAN_POINT('Ctrl Pts',(-1.98584238283279,-1.,-0.159106226437289));
#44781=CARTESIAN_POINT('Ctrl Pts',(-1.98584238283279,1.,-0.159106226437289));
#44782=CARTESIAN_POINT('Ctrl Pts',(-1.99169810931893,-1.,-0.157533331459215));
#44783=CARTESIAN_POINT('Ctrl Pts',(-1.99169810931893,1.,-0.157533331459215));
#44784=CARTESIAN_POINT('Ctrl Pts',(-1.99753284771487,-1.,-0.155904629548775));
#44785=CARTESIAN_POINT('Ctrl Pts',(-1.99753284771487,1.,-0.155904629548775));
#44786=CARTESIAN_POINT('Ctrl Pts',(-2.00335565310539,-1.,-0.154221403049719));
#44787=CARTESIAN_POINT('Ctrl Pts',(-2.00335565310539,1.,-0.154221403049719));
#44788=CARTESIAN_POINT('Ctrl Pts',(-2.00917680318426,-1.,-0.152484883621452));
#44789=CARTESIAN_POINT('Ctrl Pts',(-2.00917680318426,1.,-0.152484883621452));
#44790=CARTESIAN_POINT('Ctrl Pts',(-2.01500291940243,-1.,-0.150696157673084));
#44791=CARTESIAN_POINT('Ctrl Pts',(-2.01500291940243,1.,-0.150696157673084));
#44792=CARTESIAN_POINT('Ctrl Pts',(-2.02083464969897,-1.,-0.148856124775343));
#44793=CARTESIAN_POINT('Ctrl Pts',(-2.02083464969897,1.,-0.148856124775343));
#44794=CARTESIAN_POINT('Ctrl Pts',(-2.02666926182017,-1.,-0.146965557332586));
#44795=CARTESIAN_POINT('Ctrl Pts',(-2.02666926182017,1.,-0.146965557332586));
#44796=CARTESIAN_POINT('Ctrl Pts',(-2.03250223739941,-1.,-0.145025140186058));
#44797=CARTESIAN_POINT('Ctrl Pts',(-2.03250223739941,1.,-0.145025140186058));
#44798=CARTESIAN_POINT('Ctrl Pts',(-2.03832911025913,-1.,-0.143035515058208));
#44799=CARTESIAN_POINT('Ctrl Pts',(-2.03832911025913,1.,-0.143035515058208));
#44800=CARTESIAN_POINT('Ctrl Pts',(-2.04414757947919,-1.,-0.140997332152545));
#44801=CARTESIAN_POINT('Ctrl Pts',(-2.04414757947919,1.,-0.140997332152545));
#44802=CARTESIAN_POINT('Ctrl Pts',(-2.04995762001333,-1.,-0.138911255368966));
#44803=CARTESIAN_POINT('Ctrl Pts',(-2.04995762001333,1.,-0.138911255368966));
#44804=CARTESIAN_POINT('Ctrl Pts',(-2.0557604441427,-1.,-0.136777941218044));
#44805=CARTESIAN_POINT('Ctrl Pts',(-2.0557604441427,1.,-0.136777941218044));
#44806=CARTESIAN_POINT('Ctrl Pts',(-2.06155781517844,-1.,-0.134598026192107));
#44807=CARTESIAN_POINT('Ctrl Pts',(-2.06155781517844,1.,-0.134598026192107));
#44808=CARTESIAN_POINT('Ctrl Pts',(-2.06735123910319,-1.,-0.13237211154771));
#44809=CARTESIAN_POINT('Ctrl Pts',(-2.06735123910319,1.,-0.13237211154771));
#44810=CARTESIAN_POINT('Ctrl Pts',(-2.07314114713047,-1.,-0.130100748328401));
#44811=CARTESIAN_POINT('Ctrl Pts',(-2.07314114713047,1.,-0.130100748328401));
#44812=CARTESIAN_POINT('Ctrl Pts',(-2.07892715110967,-1.,-0.127784445276116));
#44813=CARTESIAN_POINT('Ctrl Pts',(-2.07892715110967,1.,-0.127784445276116));
#44814=CARTESIAN_POINT('Ctrl Pts',(-2.08470840653628,-1.,-0.125423679412058));
#44815=CARTESIAN_POINT('Ctrl Pts',(-2.08470840653628,1.,-0.125423679412058));
#44816=CARTESIAN_POINT('Ctrl Pts',(-2.09048392424826,-1.,-0.123018905621083));
#44817=CARTESIAN_POINT('Ctrl Pts',(-2.09048392424826,1.,-0.123018905621083));
#44818=CARTESIAN_POINT('Ctrl Pts',(-2.09625292867756,-1.,-0.120570567965129));
#44819=CARTESIAN_POINT('Ctrl Pts',(-2.09625292867756,1.,-0.120570567965129));
#44820=CARTESIAN_POINT('Ctrl Pts',(-2.10201512132945,-1.,-0.118079107988368));
#44821=CARTESIAN_POINT('Ctrl Pts',(-2.10201512132945,1.,-0.118079107988368));
#44822=CARTESIAN_POINT('Ctrl Pts',(-2.10777050261359,-1.,-0.11554495768794));
#44823=CARTESIAN_POINT('Ctrl Pts',(-2.10777050261359,1.,-0.11554495768794));
#44824=CARTESIAN_POINT('Ctrl Pts',(-2.11351924490335,-1.,-0.112968534419746));
#44825=CARTESIAN_POINT('Ctrl Pts',(-2.11351924490335,1.,-0.112968534419746));
#44826=CARTESIAN_POINT('Ctrl Pts',(-2.11926155590849,-1.,-0.11035023613502));
#44827=CARTESIAN_POINT('Ctrl Pts',(-2.11926155590849,1.,-0.11035023613502));
#44828=CARTESIAN_POINT('Ctrl Pts',(-2.12499752306927,-1.,-0.107690435231068));
#44829=CARTESIAN_POINT('Ctrl Pts',(-2.12499752306927,1.,-0.107690435231068));
#44830=CARTESIAN_POINT('Ctrl Pts',(-2.1307270488718,-1.,-0.104989479152703));
#44831=CARTESIAN_POINT('Ctrl Pts',(-2.1307270488718,1.,-0.104989479152703));
#44832=CARTESIAN_POINT('Ctrl Pts',(-2.13644992667052,-1.,-0.102247700556064));
#44833=CARTESIAN_POINT('Ctrl Pts',(-2.13644992667052,1.,-0.102247700556064));
#44834=CARTESIAN_POINT('Ctrl Pts',(-2.14216588395974,-1.,-0.0994654261990744));
#44835=CARTESIAN_POINT('Ctrl Pts',(-2.14216588395974,1.,-0.0994654261990744));
#44836=CARTESIAN_POINT('Ctrl Pts',(-2.14787463531864,-1.,-0.096642985230569));
#44837=CARTESIAN_POINT('Ctrl Pts',(-2.14787463531864,1.,-0.096642985230569));
#44838=CARTESIAN_POINT('Ctrl Pts',(-2.15357593978377,-1.,-0.0937807218868346));
#44839=CARTESIAN_POINT('Ctrl Pts',(-2.15357593978377,1.,-0.0937807218868346));
#44840=CARTESIAN_POINT('Ctrl Pts',(-2.15926961544808,-1.,-0.0908789888108267));
#44841=CARTESIAN_POINT('Ctrl Pts',(-2.15926961544808,1.,-0.0908789888108267));
#44842=CARTESIAN_POINT('Ctrl Pts',(-2.16495552645275,-1.,-0.0879381291387824));
#44843=CARTESIAN_POINT('Ctrl Pts',(-2.16495552645275,1.,-0.0879381291387824));
#44844=CARTESIAN_POINT('Ctrl Pts',(-2.17063357871031,-1.,-0.0849584620835644));
#44845=CARTESIAN_POINT('Ctrl Pts',(-2.17063357871031,1.,-0.0849584620835644));
#44846=CARTESIAN_POINT('Ctrl Pts',(-2.1763037121106,-1.,-0.0819402680871941));
#44847=CARTESIAN_POINT('Ctrl Pts',(-2.1763037121106,1.,-0.0819402680871941));
#44848=CARTESIAN_POINT('Ctrl Pts',(-2.18196589448304,-1.,-0.0788837727683229));
#44849=CARTESIAN_POINT('Ctrl Pts',(-2.18196589448304,1.,-0.0788837727683229));
#44850=CARTESIAN_POINT('Ctrl Pts',(-2.1876201139874,-1.,-0.0757891465833413));
#44851=CARTESIAN_POINT('Ctrl Pts',(-2.1876201139874,1.,-0.0757891465833413));
#44852=CARTESIAN_POINT('Ctrl Pts',(-2.19213712012956,-1.,-0.0732830357304277));
#44853=CARTESIAN_POINT('Ctrl Pts',(-2.19213712012956,1.,-0.0732830357304277));
#44854=CARTESIAN_POINT('Ctrl Pts',(-2.19552129483562,-1.,-0.0713863779524629));
#44855=CARTESIAN_POINT('Ctrl Pts',(-2.19552129483562,1.,-0.0713863779524629));
#44856=CARTESIAN_POINT('Ctrl Pts',(-2.19777582085261,-1.,-0.0701143536324927));
#44857=CARTESIAN_POINT('Ctrl Pts',(-2.19777582085261,1.,-0.0701143536324927));
#44858=CARTESIAN_POINT('Ctrl Pts',(-2.19890268624765,-1.,-0.0694764450219585));
#44859=CARTESIAN_POINT('Ctrl Pts',(-2.19890268624765,1.,-0.0694764450219585));
#44860=CARTESIAN_POINT('',(-1.74236521665491,1.,-0.163289472382896));
#44861=CARTESIAN_POINT('Ctrl Pts',(-1.74236521665491,1.,-0.163289472382896));
#44862=CARTESIAN_POINT('Ctrl Pts',(-1.74720349503904,1.,-0.163814161002474));
#44863=CARTESIAN_POINT('Ctrl Pts',(-1.75666056640041,1.,-0.164834765708484));
#44864=CARTESIAN_POINT('Ctrl Pts',(-1.77018771687692,1.,-0.166279355148738));
#44865=CARTESIAN_POINT('Ctrl Pts',(-1.78690649988931,1.,-0.16803277280837));
#44866=CARTESIAN_POINT('Ctrl Pts',(-1.80561530633924,1.,-0.169936923908078));
#44867=CARTESIAN_POINT('Ctrl Pts',(-1.82215766815414,1.,-0.171554770207306));
#44868=CARTESIAN_POINT('Ctrl Pts',(-1.83658380530747,1.,-0.17288944289442));
#44869=CARTESIAN_POINT('Ctrl Pts',(-1.84898113200543,1.,-0.173946627589401));
#44870=CARTESIAN_POINT('Ctrl Pts',(-1.85948367089838,1.,-0.174735259276856));
#44871=CARTESIAN_POINT('Ctrl Pts',(-1.86828349694972,1.,-0.175268337590901));
#44872=CARTESIAN_POINT('Ctrl Pts',(-1.87563767773249,1.,-0.175563480746205));
#44873=CARTESIAN_POINT('Ctrl Pts',(-1.88188663144846,1.,-0.175644148889271));
#44874=CARTESIAN_POINT('Ctrl Pts',(-1.88742606272818,1.,-0.175538155840286));
#44875=CARTESIAN_POINT('Ctrl Pts',(-1.89264630198279,1.,-0.175274276190664));
#44876=CARTESIAN_POINT('Ctrl Pts',(-1.89788101117148,1.,-0.174879405091277));
#44877=CARTESIAN_POINT('Ctrl Pts',(-1.90335253863003,1.,-0.174375518661222));
#44878=CARTESIAN_POINT('Ctrl Pts',(-1.90911693975475,1.,-0.173776635257984));
#44879=CARTESIAN_POINT('Ctrl Pts',(-1.91511429159681,1.,-0.173090695383619));
#44880=CARTESIAN_POINT('Ctrl Pts',(-1.92122334398034,1.,-0.172321621259557));
#44881=CARTESIAN_POINT('Ctrl Pts',(-1.92731093582,1.,-0.17147119153296));
#44882=CARTESIAN_POINT('Ctrl Pts',(-1.93329183155455,1.,-0.170541253116136));
#44883=CARTESIAN_POINT('Ctrl Pts',(-1.93915639211497,1.,-0.169534904817425));
#44884=CARTESIAN_POINT('Ctrl Pts',(-1.94493757756879,1.,-0.168455741607516));
#44885=CARTESIAN_POINT('Ctrl Pts',(-1.95069027794286,1.,-0.167307501784469));
#44886=CARTESIAN_POINT('Ctrl Pts',(-1.95646759718755,1.,-0.166093592002833));
#44887=CARTESIAN_POINT('Ctrl Pts',(-1.96229379940174,1.,-0.1648165689203));
#44888=CARTESIAN_POINT('Ctrl Pts',(-1.96816512678,1.,-0.16347818545776));
#44889=CARTESIAN_POINT('Ctrl Pts',(-1.97406280235204,1.,-0.162079693556302));
#44890=CARTESIAN_POINT('Ctrl Pts',(-1.97996195437557,1.,-0.16062206078461));
#44891=CARTESIAN_POINT('Ctrl Pts',(-1.98584238283279,1.,-0.159106226437289));
#44892=CARTESIAN_POINT('Ctrl Pts',(-1.99169810931893,1.,-0.157533331459215));
#44893=CARTESIAN_POINT('Ctrl Pts',(-1.99753284771487,1.,-0.155904629548775));
#44894=CARTESIAN_POINT('Ctrl Pts',(-2.00335565310539,1.,-0.154221403049719));
#44895=CARTESIAN_POINT('Ctrl Pts',(-2.00917680318426,1.,-0.152484883621452));
#44896=CARTESIAN_POINT('Ctrl Pts',(-2.01500291940243,1.,-0.150696157673084));
#44897=CARTESIAN_POINT('Ctrl Pts',(-2.02083464969897,1.,-0.148856124775343));
#44898=CARTESIAN_POINT('Ctrl Pts',(-2.02666926182017,1.,-0.146965557332586));
#44899=CARTESIAN_POINT('Ctrl Pts',(-2.03250223739941,1.,-0.145025140186058));
#44900=CARTESIAN_POINT('Ctrl Pts',(-2.03832911025913,1.,-0.143035515058208));
#44901=CARTESIAN_POINT('Ctrl Pts',(-2.04414757947919,1.,-0.140997332152545));
#44902=CARTESIAN_POINT('Ctrl Pts',(-2.04995762001333,1.,-0.138911255368966));
#44903=CARTESIAN_POINT('Ctrl Pts',(-2.0557604441427,1.,-0.136777941218044));
#44904=CARTESIAN_POINT('Ctrl Pts',(-2.06155781517844,1.,-0.134598026192107));
#44905=CARTESIAN_POINT('Ctrl Pts',(-2.06735123910319,1.,-0.13237211154771));
#44906=CARTESIAN_POINT('Ctrl Pts',(-2.07314114713047,1.,-0.130100748328401));
#44907=CARTESIAN_POINT('Ctrl Pts',(-2.07892715110967,1.,-0.127784445276116));
#44908=CARTESIAN_POINT('Ctrl Pts',(-2.08470840653628,1.,-0.125423679412058));
#44909=CARTESIAN_POINT('Ctrl Pts',(-2.09048392424826,1.,-0.123018905621083));
#44910=CARTESIAN_POINT('Ctrl Pts',(-2.09625292867756,1.,-0.120570567965129));
#44911=CARTESIAN_POINT('Ctrl Pts',(-2.10201512132945,1.,-0.118079107988368));
#44912=CARTESIAN_POINT('Ctrl Pts',(-2.10777050261359,1.,-0.11554495768794));
#44913=CARTESIAN_POINT('Ctrl Pts',(-2.11351924490335,1.,-0.112968534419746));
#44914=CARTESIAN_POINT('Ctrl Pts',(-2.11926155590849,1.,-0.11035023613502));
#44915=CARTESIAN_POINT('Ctrl Pts',(-2.12499752306927,1.,-0.107690435231068));
#44916=CARTESIAN_POINT('Ctrl Pts',(-2.1307270488718,1.,-0.104989479152703));
#44917=CARTESIAN_POINT('Ctrl Pts',(-2.13644992667052,1.,-0.102247700556064));
#44918=CARTESIAN_POINT('Ctrl Pts',(-2.14216588395974,1.,-0.0994654261990744));
#44919=CARTESIAN_POINT('Ctrl Pts',(-2.14787463531864,1.,-0.096642985230569));
#44920=CARTESIAN_POINT('Ctrl Pts',(-2.15357593978377,1.,-0.0937807218868346));
#44921=CARTESIAN_POINT('Ctrl Pts',(-2.15926961544808,1.,-0.0908789888108267));
#44922=CARTESIAN_POINT('Ctrl Pts',(-2.16495552645275,1.,-0.0879381291387824));
#44923=CARTESIAN_POINT('Ctrl Pts',(-2.17063357871031,1.,-0.0849584620835644));
#44924=CARTESIAN_POINT('Ctrl Pts',(-2.1763037121106,1.,-0.0819402680871941));
#44925=CARTESIAN_POINT('Ctrl Pts',(-2.18196589448304,1.,-0.0788837727683229));
#44926=CARTESIAN_POINT('Ctrl Pts',(-2.1876201139874,1.,-0.0757891465833413));
#44927=CARTESIAN_POINT('Ctrl Pts',(-2.19213712012956,1.,-0.0732830357304277));
#44928=CARTESIAN_POINT('Ctrl Pts',(-2.19552129483562,1.,-0.0713863779524629));
#44929=CARTESIAN_POINT('Ctrl Pts',(-2.19777582085261,1.,-0.0701143536324927));
#44930=CARTESIAN_POINT('Ctrl Pts',(-2.19890268624765,1.,-0.0694764450219585));
#44931=CARTESIAN_POINT('',(-1.74236521665491,0.,-0.163289472382896));
#44932=CARTESIAN_POINT('Origin',(0.,0.,0.));
#44933=CARTESIAN_POINT('',(-1.7075470150345,1.,-0.383122945602004));
#44934=CARTESIAN_POINT('Origin',(0.,1.,0.));
#44935=CARTESIAN_POINT('',(-1.7075470150345,0.,-0.383122945602004));
#44936=CARTESIAN_POINT('Ctrl Pts',(-2.11275013067528,-1.,-0.61342227326009));
#44937=CARTESIAN_POINT('Ctrl Pts',(-2.11275013067528,1.,-0.61342227326009));
#44938=CARTESIAN_POINT('Ctrl Pts',(-2.11187554260142,-1.,-0.61246736556225));
#44939=CARTESIAN_POINT('Ctrl Pts',(-2.11187554260142,1.,-0.61246736556225));
#44940=CARTESIAN_POINT('Ctrl Pts',(-2.11012443807661,-1.,-0.610560911691113));
#44941=CARTESIAN_POINT('Ctrl Pts',(-2.11012443807661,1.,-0.610560911691113));
#44942=CARTESIAN_POINT('Ctrl Pts',(-2.10749199615859,-1.,-0.607711315456826));
#44943=CARTESIAN_POINT('Ctrl Pts',(-2.10749199615859,1.,-0.607711315456826));
#44944=CARTESIAN_POINT('Ctrl Pts',(-2.10397049887709,-1.,-0.603932030738212));
#44945=CARTESIAN_POINT('Ctrl Pts',(-2.10397049887709,1.,-0.603932030738212));
#44946=CARTESIAN_POINT('Ctrl Pts',(-2.09954930865331,-1.,-0.599241616422144));
#44947=CARTESIAN_POINT('Ctrl Pts',(-2.09954930865331,1.,-0.599241616422144));
#44948=CARTESIAN_POINT('Ctrl Pts',(-2.09510876220501,-1.,-0.594585006052823));
#44949=CARTESIAN_POINT('Ctrl Pts',(-2.09510876220501,1.,-0.594585006052823));
#44950=CARTESIAN_POINT('Ctrl Pts',(-2.09064881812053,-1.,-0.589962365403189));
#44951=CARTESIAN_POINT('Ctrl Pts',(-2.09064881812053,1.,-0.589962365403189));
#44952=CARTESIAN_POINT('Ctrl Pts',(-2.086169437277,-1.,-0.585373918990895));
#44953=CARTESIAN_POINT('Ctrl Pts',(-2.086169437277,1.,-0.585373918990895));
#44954=CARTESIAN_POINT('Ctrl Pts',(-2.08167059018138,-1.,-0.580819952107257));
#44955=CARTESIAN_POINT('Ctrl Pts',(-2.08167059018138,1.,-0.580819952107257));
#44956=CARTESIAN_POINT('Ctrl Pts',(-2.07715226767361,-1.,-0.576300797416274));
#44957=CARTESIAN_POINT('Ctrl Pts',(-2.07715226767361,1.,-0.576300797416274));
#44958=CARTESIAN_POINT('Ctrl Pts',(-2.07261449292757,-1.,-0.571816823242411));
#44959=CARTESIAN_POINT('Ctrl Pts',(-2.07261449292757,1.,-0.571816823242411));
#44960=CARTESIAN_POINT('Ctrl Pts',(-2.06805732997383,-1.,-0.567368421181229));
#44961=CARTESIAN_POINT('Ctrl Pts',(-2.06805732997383,1.,-0.567368421181229));
#44962=CARTESIAN_POINT('Ctrl Pts',(-2.06348090160697,-1.,-0.562955993082574));
#44963=CARTESIAN_POINT('Ctrl Pts',(-2.06348090160697,1.,-0.562955993082574));
#44964=CARTESIAN_POINT('Ctrl Pts',(-2.05888537756571,-1.,-0.558579940185467));
#44965=CARTESIAN_POINT('Ctrl Pts',(-2.05888537756571,1.,-0.558579940185467));
#44966=CARTESIAN_POINT('Ctrl Pts',(-2.05427091604482,-1.,-0.554240657464109));
#44967=CARTESIAN_POINT('Ctrl Pts',(-2.05427091604482,1.,-0.554240657464109));
#44968=CARTESIAN_POINT('Ctrl Pts',(-2.04963761077974,-1.,-0.549938525150342));
#44969=CARTESIAN_POINT('Ctrl Pts',(-2.04963761077974,1.,-0.549938525150342));
#44970=CARTESIAN_POINT('Ctrl Pts',(-2.0449854471456,-1.,-0.545673903817348));
#44971=CARTESIAN_POINT('Ctrl Pts',(-2.0449854471456,1.,-0.545673903817348));
#44972=CARTESIAN_POINT('Ctrl Pts',(-2.0403142269048,-1.,-0.54144712061552));
#44973=CARTESIAN_POINT('Ctrl Pts',(-2.0403142269048,1.,-0.54144712061552));
#44974=CARTESIAN_POINT('Ctrl Pts',(-2.03562362953993,-1.,-0.537258489833134));
#44975=CARTESIAN_POINT('Ctrl Pts',(-2.03562362953993,1.,-0.537258489833134));
#44976=CARTESIAN_POINT('Ctrl Pts',(-2.03091336214401,-1.,-0.533108355132905));
#44977=CARTESIAN_POINT('Ctrl Pts',(-2.03091336214401,1.,-0.533108355132905));
#44978=CARTESIAN_POINT('Ctrl Pts',(-2.02618329083289,-1.,-0.52899712724191));
#44979=CARTESIAN_POINT('Ctrl Pts',(-2.02618329083289,1.,-0.52899712724191));
#44980=CARTESIAN_POINT('Ctrl Pts',(-2.02143356304712,-1.,-0.524925318333518));
#44981=CARTESIAN_POINT('Ctrl Pts',(-2.02143356304712,1.,-0.524925318333518));
#44982=CARTESIAN_POINT('Ctrl Pts',(-2.01666477917305,-1.,-0.520893590399428));
#44983=CARTESIAN_POINT('Ctrl Pts',(-2.01666477917305,1.,-0.520893590399428));
#44984=CARTESIAN_POINT('Ctrl Pts',(-2.01187773939257,-1.,-0.516902681728733));
#44985=CARTESIAN_POINT('Ctrl Pts',(-2.01187773939257,1.,-0.516902681728733));
#44986=CARTESIAN_POINT('Ctrl Pts',(-2.00707309946955,-1.,-0.512953306961813));
#44987=CARTESIAN_POINT('Ctrl Pts',(-2.00707309946955,1.,-0.512953306961813));
#44988=CARTESIAN_POINT('Ctrl Pts',(-2.00225107134733,-1.,-0.509046069886152));
#44989=CARTESIAN_POINT('Ctrl Pts',(-2.00225107134733,1.,-0.509046069886152));
#44990=CARTESIAN_POINT('Ctrl Pts',(-1.99741107463567,-1.,-0.505181361323011));
#44991=CARTESIAN_POINT('Ctrl Pts',(-1.99741107463567,1.,-0.505181361323011));
#44992=CARTESIAN_POINT('Ctrl Pts',(-1.9925514912615,-1.,-0.501359287727129));
#44993=CARTESIAN_POINT('Ctrl Pts',(-1.9925514912615,1.,-0.501359287727129));
#44994=CARTESIAN_POINT('Ctrl Pts',(-1.98767044752929,-1.,-0.497579909545564));
#44995=CARTESIAN_POINT('Ctrl Pts',(-1.98767044752929,1.,-0.497579909545564));
#44996=CARTESIAN_POINT('Ctrl Pts',(-1.9827665876182,-1.,-0.493843476541492));
#44997=CARTESIAN_POINT('Ctrl Pts',(-1.9827665876182,1.,-0.493843476541492));
#44998=CARTESIAN_POINT('Ctrl Pts',(-1.97783973019229,-1.,-0.490150627860955));
#44999=CARTESIAN_POINT('Ctrl Pts',(-1.97783973019229,1.,-0.490150627860955));
#45000=CARTESIAN_POINT('Ctrl Pts',(-1.97289186263272,-1.,-0.486502692907661));
#45001=CARTESIAN_POINT('Ctrl Pts',(-1.97289186263272,1.,-0.486502692907661));
#45002=CARTESIAN_POINT('Ctrl Pts',(-1.96792703422358,-1.,-0.482901662120686));
#45003=CARTESIAN_POINT('Ctrl Pts',(-1.96792703422358,1.,-0.482901662120686));
#45004=CARTESIAN_POINT('Ctrl Pts',(-1.96294933055938,-1.,-0.479349583074846));
#45005=CARTESIAN_POINT('Ctrl Pts',(-1.96294933055938,1.,-0.479349583074846));
#45006=CARTESIAN_POINT('Ctrl Pts',(-1.95796111148175,-1.,-0.475848034683171));
#45007=CARTESIAN_POINT('Ctrl Pts',(-1.95796111148175,1.,-0.475848034683171));
#45008=CARTESIAN_POINT('Ctrl Pts',(-1.95296148278136,-1.,-0.472397672264079));
#45009=CARTESIAN_POINT('Ctrl Pts',(-1.95296148278136,1.,-0.472397672264079));
#45010=CARTESIAN_POINT('Ctrl Pts',(-1.94794381136524,-1.,-0.468997482913158));
#45011=CARTESIAN_POINT('Ctrl Pts',(-1.94794381136524,1.,-0.468997482913158));
#45012=CARTESIAN_POINT('Ctrl Pts',(-1.94289794196205,-1.,-0.465645462026064));
#45013=CARTESIAN_POINT('Ctrl Pts',(-1.94289794196205,1.,-0.465645462026064));
#45014=CARTESIAN_POINT('Ctrl Pts',(-1.93781486640834,-1.,-0.462340031009087));
#45015=CARTESIAN_POINT('Ctrl Pts',(-1.93781486640834,1.,-0.462340031009087));
#45016=CARTESIAN_POINT('Ctrl Pts',(-1.93269066517936,-1.,-0.459081234547931));
#45017=CARTESIAN_POINT('Ctrl Pts',(-1.93269066517936,1.,-0.459081234547931));
#45018=CARTESIAN_POINT('Ctrl Pts',(-1.92753067150461,-1.,-0.455872005174335));
#45019=CARTESIAN_POINT('Ctrl Pts',(-1.92753067150461,1.,-0.455872005174335));
#45020=CARTESIAN_POINT('Ctrl Pts',(-1.9223538064847,-1.,-0.452719478359356));
#45021=CARTESIAN_POINT('Ctrl Pts',(-1.9223538064847,1.,-0.452719478359356));
#45022=CARTESIAN_POINT('Ctrl Pts',(-1.91718342555717,-1.,-0.449632260106572));
#45023=CARTESIAN_POINT('Ctrl Pts',(-1.91718342555717,1.,-0.449632260106572));
#45024=CARTESIAN_POINT('Ctrl Pts',(-1.91203699981095,-1.,-0.446617343485651));
#45025=CARTESIAN_POINT('Ctrl Pts',(-1.91203699981095,1.,-0.446617343485651));
#45026=CARTESIAN_POINT('Ctrl Pts',(-1.90691756144906,-1.,-0.44367755684917));
#45027=CARTESIAN_POINT('Ctrl Pts',(-1.90691756144906,1.,-0.44367755684917));
#45028=CARTESIAN_POINT('Ctrl Pts',(-1.90180124389137,-1.,-0.44080783370416));
#45029=CARTESIAN_POINT('Ctrl Pts',(-1.90180124389137,1.,-0.44080783370416));
#45030=CARTESIAN_POINT('Ctrl Pts',(-1.89663648956549,-1.,-0.437995003948443));
#45031=CARTESIAN_POINT('Ctrl Pts',(-1.89663648956549,1.,-0.437995003948443));
#45032=CARTESIAN_POINT('Ctrl Pts',(-1.89136993975585,-1.,-0.43522566096358));
#45033=CARTESIAN_POINT('Ctrl Pts',(-1.89136993975585,1.,-0.43522566096358));
#45034=CARTESIAN_POINT('Ctrl Pts',(-1.88596913666828,-1.,-0.432493038548833));
#45035=CARTESIAN_POINT('Ctrl Pts',(-1.88596913666828,1.,-0.432493038548833));
#45036=CARTESIAN_POINT('Ctrl Pts',(-1.88044229001778,-1.,-0.429803062482217));
#45037=CARTESIAN_POINT('Ctrl Pts',(-1.88044229001778,1.,-0.429803062482217));
#45038=CARTESIAN_POINT('Ctrl Pts',(-1.87486989291333,-1.,-0.427183828518743));
#45039=CARTESIAN_POINT('Ctrl Pts',(-1.87486989291333,1.,-0.427183828518743));
#45040=CARTESIAN_POINT('Ctrl Pts',(-1.8693780394412,-1.,-0.424678177290876));
#45041=CARTESIAN_POINT('Ctrl Pts',(-1.8693780394412,1.,-0.424678177290876));
#45042=CARTESIAN_POINT('Ctrl Pts',(-1.86408083333863,-1.,-0.422327307417884));
#45043=CARTESIAN_POINT('Ctrl Pts',(-1.86408083333863,1.,-0.422327307417884));
#45044=CARTESIAN_POINT('Ctrl Pts',(-1.8590328109667,-1.,-0.420157287975583));
#45045=CARTESIAN_POINT('Ctrl Pts',(-1.8590328109667,1.,-0.420157287975583));
#45046=CARTESIAN_POINT('Ctrl Pts',(-1.8541763285645,-1.,-0.418164129144045));
#45047=CARTESIAN_POINT('Ctrl Pts',(-1.8541763285645,1.,-0.418164129144045));
#45048=CARTESIAN_POINT('Ctrl Pts',(-1.84929312930314,-1.,-0.416300022039885));
#45049=CARTESIAN_POINT('Ctrl Pts',(-1.84929312930314,1.,-0.416300022039885));
#45050=CARTESIAN_POINT('Ctrl Pts',(-1.84405757074218,-1.,-0.414487438255542));
#45051=CARTESIAN_POINT('Ctrl Pts',(-1.84405757074218,1.,-0.414487438255542));
#45052=CARTESIAN_POINT('Ctrl Pts',(-1.8380895347617,-1.,-0.412633125322945));
#45053=CARTESIAN_POINT('Ctrl Pts',(-1.8380895347617,1.,-0.412633125322945));
#45054=CARTESIAN_POINT('Ctrl Pts',(-1.83100408895047,-1.,-0.410641256301276));
#45055=CARTESIAN_POINT('Ctrl Pts',(-1.83100408895047,1.,-0.410641256301276));
#45056=CARTESIAN_POINT('Ctrl Pts',(-1.82247022677562,-1.,-0.408428948106227));
#45057=CARTESIAN_POINT('Ctrl Pts',(-1.82247022677562,1.,-0.408428948106227));
#45058=CARTESIAN_POINT('Ctrl Pts',(-1.81223801812013,-1.,-0.405933518407175));
#45059=CARTESIAN_POINT('Ctrl Pts',(-1.81223801812013,1.,-0.405933518407175));
#45060=CARTESIAN_POINT('Ctrl Pts',(-1.80012077173238,-1.,-0.403107976163396));
#45061=CARTESIAN_POINT('Ctrl Pts',(-1.80012077173238,1.,-0.403107976163396));
#45062=CARTESIAN_POINT('Ctrl Pts',(-1.78598826343754,-1.,-0.399919403774155));
#45063=CARTESIAN_POINT('Ctrl Pts',(-1.78598826343754,1.,-0.399919403774155));
#45064=CARTESIAN_POINT('Ctrl Pts',(-1.76975560043442,-1.,-0.396346196110688));
#45065=CARTESIAN_POINT('Ctrl Pts',(-1.76975560043442,1.,-0.396346196110688));
#45066=CARTESIAN_POINT('Ctrl Pts',(-1.75137405310193,-1.,-0.392375812285395));
#45067=CARTESIAN_POINT('Ctrl Pts',(-1.75137405310193,1.,-0.392375812285395));
#45068=CARTESIAN_POINT('Ctrl Pts',(-1.73493170972829,-1.,-0.388877023502615));
#45069=CARTESIAN_POINT('Ctrl Pts',(-1.73493170972829,1.,-0.388877023502615));
#45070=CARTESIAN_POINT('Ctrl Pts',(-1.72162022244582,-1.,-0.386070790323281));
#45071=CARTESIAN_POINT('Ctrl Pts',(-1.72162022244582,1.,-0.386070790323281));
#45072=CARTESIAN_POINT('Ctrl Pts',(-1.71231062891398,-1.,-0.384119047314215));
#45073=CARTESIAN_POINT('Ctrl Pts',(-1.71231062891398,1.,-0.384119047314215));
#45074=CARTESIAN_POINT('Ctrl Pts',(-1.7075470150345,-1.,-0.383122945602004));
#45075=CARTESIAN_POINT('Ctrl Pts',(-1.7075470150345,1.,-0.383122945602004));
#45076=CARTESIAN_POINT('',(-2.11275013067528,1.,-0.61342227326009));
#45077=CARTESIAN_POINT('Ctrl Pts',(-2.11275013067528,1.,-0.61342227326009));
#45078=CARTESIAN_POINT('Ctrl Pts',(-2.11187554260142,1.,-0.61246736556225));
#45079=CARTESIAN_POINT('Ctrl Pts',(-2.11012443807661,1.,-0.610560911691113));
#45080=CARTESIAN_POINT('Ctrl Pts',(-2.10749199615859,1.,-0.607711315456826));
#45081=CARTESIAN_POINT('Ctrl Pts',(-2.10397049887709,1.,-0.603932030738212));
#45082=CARTESIAN_POINT('Ctrl Pts',(-2.09954930865331,1.,-0.599241616422144));
#45083=CARTESIAN_POINT('Ctrl Pts',(-2.09510876220501,1.,-0.594585006052823));
#45084=CARTESIAN_POINT('Ctrl Pts',(-2.09064881812053,1.,-0.589962365403189));
#45085=CARTESIAN_POINT('Ctrl Pts',(-2.086169437277,1.,-0.585373918990895));
#45086=CARTESIAN_POINT('Ctrl Pts',(-2.08167059018138,1.,-0.580819952107257));
#45087=CARTESIAN_POINT('Ctrl Pts',(-2.07715226767361,1.,-0.576300797416274));
#45088=CARTESIAN_POINT('Ctrl Pts',(-2.07261449292757,1.,-0.571816823242411));
#45089=CARTESIAN_POINT('Ctrl Pts',(-2.06805732997383,1.,-0.567368421181229));
#45090=CARTESIAN_POINT('Ctrl Pts',(-2.06348090160697,1.,-0.562955993082574));
#45091=CARTESIAN_POINT('Ctrl Pts',(-2.05888537756571,1.,-0.558579940185467));
#45092=CARTESIAN_POINT('Ctrl Pts',(-2.05427091604482,1.,-0.554240657464109));
#45093=CARTESIAN_POINT('Ctrl Pts',(-2.04963761077974,1.,-0.549938525150342));
#45094=CARTESIAN_POINT('Ctrl Pts',(-2.0449854471456,1.,-0.545673903817348));
#45095=CARTESIAN_POINT('Ctrl Pts',(-2.0403142269048,1.,-0.54144712061552));
#45096=CARTESIAN_POINT('Ctrl Pts',(-2.03562362953993,1.,-0.537258489833134));
#45097=CARTESIAN_POINT('Ctrl Pts',(-2.03091336214401,1.,-0.533108355132905));
#45098=CARTESIAN_POINT('Ctrl Pts',(-2.02618329083289,1.,-0.52899712724191));
#45099=CARTESIAN_POINT('Ctrl Pts',(-2.02143356304712,1.,-0.524925318333518));
#45100=CARTESIAN_POINT('Ctrl Pts',(-2.01666477917305,1.,-0.520893590399428));
#45101=CARTESIAN_POINT('Ctrl Pts',(-2.01187773939257,1.,-0.516902681728733));
#45102=CARTESIAN_POINT('Ctrl Pts',(-2.00707309946955,1.,-0.512953306961813));
#45103=CARTESIAN_POINT('Ctrl Pts',(-2.00225107134733,1.,-0.509046069886152));
#45104=CARTESIAN_POINT('Ctrl Pts',(-1.99741107463567,1.,-0.505181361323011));
#45105=CARTESIAN_POINT('Ctrl Pts',(-1.9925514912615,1.,-0.501359287727129));
#45106=CARTESIAN_POINT('Ctrl Pts',(-1.98767044752929,1.,-0.497579909545564));
#45107=CARTESIAN_POINT('Ctrl Pts',(-1.9827665876182,1.,-0.493843476541492));
#45108=CARTESIAN_POINT('Ctrl Pts',(-1.97783973019229,1.,-0.490150627860955));
#45109=CARTESIAN_POINT('Ctrl Pts',(-1.97289186263272,1.,-0.486502692907661));
#45110=CARTESIAN_POINT('Ctrl Pts',(-1.96792703422358,1.,-0.482901662120686));
#45111=CARTESIAN_POINT('Ctrl Pts',(-1.96294933055938,1.,-0.479349583074846));
#45112=CARTESIAN_POINT('Ctrl Pts',(-1.95796111148175,1.,-0.475848034683171));
#45113=CARTESIAN_POINT('Ctrl Pts',(-1.95296148278136,1.,-0.472397672264079));
#45114=CARTESIAN_POINT('Ctrl Pts',(-1.94794381136524,1.,-0.468997482913158));
#45115=CARTESIAN_POINT('Ctrl Pts',(-1.94289794196205,1.,-0.465645462026064));
#45116=CARTESIAN_POINT('Ctrl Pts',(-1.93781486640834,1.,-0.462340031009087));
#45117=CARTESIAN_POINT('Ctrl Pts',(-1.93269066517936,1.,-0.459081234547931));
#45118=CARTESIAN_POINT('Ctrl Pts',(-1.92753067150461,1.,-0.455872005174335));
#45119=CARTESIAN_POINT('Ctrl Pts',(-1.9223538064847,1.,-0.452719478359356));
#45120=CARTESIAN_POINT('Ctrl Pts',(-1.91718342555717,1.,-0.449632260106572));
#45121=CARTESIAN_POINT('Ctrl Pts',(-1.91203699981095,1.,-0.446617343485651));
#45122=CARTESIAN_POINT('Ctrl Pts',(-1.90691756144906,1.,-0.44367755684917));
#45123=CARTESIAN_POINT('Ctrl Pts',(-1.90180124389137,1.,-0.44080783370416));
#45124=CARTESIAN_POINT('Ctrl Pts',(-1.89663648956549,1.,-0.437995003948443));
#45125=CARTESIAN_POINT('Ctrl Pts',(-1.89136993975585,1.,-0.43522566096358));
#45126=CARTESIAN_POINT('Ctrl Pts',(-1.88596913666828,1.,-0.432493038548833));
#45127=CARTESIAN_POINT('Ctrl Pts',(-1.88044229001778,1.,-0.429803062482217));
#45128=CARTESIAN_POINT('Ctrl Pts',(-1.87486989291333,1.,-0.427183828518743));
#45129=CARTESIAN_POINT('Ctrl Pts',(-1.8693780394412,1.,-0.424678177290876));
#45130=CARTESIAN_POINT('Ctrl Pts',(-1.86408083333863,1.,-0.422327307417884));
#45131=CARTESIAN_POINT('Ctrl Pts',(-1.8590328109667,1.,-0.420157287975583));
#45132=CARTESIAN_POINT('Ctrl Pts',(-1.8541763285645,1.,-0.418164129144045));
#45133=CARTESIAN_POINT('Ctrl Pts',(-1.84929312930314,1.,-0.416300022039885));
#45134=CARTESIAN_POINT('Ctrl Pts',(-1.84405757074218,1.,-0.414487438255542));
#45135=CARTESIAN_POINT('Ctrl Pts',(-1.8380895347617,1.,-0.412633125322945));
#45136=CARTESIAN_POINT('Ctrl Pts',(-1.83100408895047,1.,-0.410641256301276));
#45137=CARTESIAN_POINT('Ctrl Pts',(-1.82247022677562,1.,-0.408428948106227));
#45138=CARTESIAN_POINT('Ctrl Pts',(-1.81223801812013,1.,-0.405933518407175));
#45139=CARTESIAN_POINT('Ctrl Pts',(-1.80012077173238,1.,-0.403107976163396));
#45140=CARTESIAN_POINT('Ctrl Pts',(-1.78598826343754,1.,-0.399919403774155));
#45141=CARTESIAN_POINT('Ctrl Pts',(-1.76975560043442,1.,-0.396346196110688));
#45142=CARTESIAN_POINT('Ctrl Pts',(-1.75137405310193,1.,-0.392375812285395));
#45143=CARTESIAN_POINT('Ctrl Pts',(-1.73493170972829,1.,-0.388877023502615));
#45144=CARTESIAN_POINT('Ctrl Pts',(-1.72162022244582,1.,-0.386070790323281));
#45145=CARTESIAN_POINT('Ctrl Pts',(-1.71231062891398,1.,-0.384119047314215));
#45146=CARTESIAN_POINT('Ctrl Pts',(-1.7075470150345,1.,-0.383122945602004));
#45147=CARTESIAN_POINT('',(-2.11275013067528,0.,-0.61342227326009));
#45148=CARTESIAN_POINT('Origin',(-2.0698113262342,0.,-0.745574324794401));
#45149=CARTESIAN_POINT('',(-2.0698113262342,1.,-0.745574324794401));
#45150=CARTESIAN_POINT('',(-2.11275013067528,1.,-0.61342227326009));
#45151=CARTESIAN_POINT('',(-2.0698113262342,0.,-0.745574324794401));
#45152=CARTESIAN_POINT('Ctrl Pts',(-1.60662857109684,-1.,-0.693717979106306));
#45153=CARTESIAN_POINT('Ctrl Pts',(-1.60662857109684,1.,-0.693717979106306));
#45154=CARTESIAN_POINT('Ctrl Pts',(-1.61106790958151,-1.,-0.695712097881194));
#45155=CARTESIAN_POINT('Ctrl Pts',(-1.61106790958151,1.,-0.695712097881194));
#45156=CARTESIAN_POINT('Ctrl Pts',(-1.61974673472612,-1.,-0.699605146405088));
#45157=CARTESIAN_POINT('Ctrl Pts',(-1.61974673472612,1.,-0.699605146405088));
#45158=CARTESIAN_POINT('Ctrl Pts',(-1.63216541664676,-1.,-0.705159151988319));
#45159=CARTESIAN_POINT('Ctrl Pts',(-1.63216541664676,1.,-0.705159151988319));
#45160=CARTESIAN_POINT('Ctrl Pts',(-1.64752408832016,-1.,-0.711993139355394));
#45161=CARTESIAN_POINT('Ctrl Pts',(-1.64752408832016,1.,-0.711993139355394));
#45162=CARTESIAN_POINT('Ctrl Pts',(-1.6647288055568,-1.,-0.719585433804282));
#45163=CARTESIAN_POINT('Ctrl Pts',(-1.6647288055568,1.,-0.719585433804282));
#45164=CARTESIAN_POINT('Ctrl Pts',(-1.67996158455503,-1.,-0.726235967997433));
#45165=CARTESIAN_POINT('Ctrl Pts',(-1.67996158455503,1.,-0.726235967997433));
#45166=CARTESIAN_POINT('Ctrl Pts',(-1.69326921975743,-1.,-0.731963238697195));
#45167=CARTESIAN_POINT('Ctrl Pts',(-1.69326921975743,1.,-0.731963238697195));
#45168=CARTESIAN_POINT('Ctrl Pts',(-1.70473309006121,-1.,-0.736799665724771));
#45169=CARTESIAN_POINT('Ctrl Pts',(-1.70473309006121,1.,-0.736799665724771));
#45170=CARTESIAN_POINT('Ctrl Pts',(-1.71447789751927,-1.,-0.740795162032087));
#45171=CARTESIAN_POINT('Ctrl Pts',(-1.71447789751927,1.,-0.740795162032087));
#45172=CARTESIAN_POINT('Ctrl Pts',(-1.7226822991693,-1.,-0.744021445433764));
#45173=CARTESIAN_POINT('Ctrl Pts',(-1.7226822991693,1.,-0.744021445433764));
#45174=CARTESIAN_POINT('Ctrl Pts',(-1.72958533647399,-1.,-0.746574710096436));
#45175=CARTESIAN_POINT('Ctrl Pts',(-1.72958533647399,1.,-0.746574710096436));
#45176=CARTESIAN_POINT('Ctrl Pts',(-1.73550351679848,-1.,-0.748582462954854));
#45177=CARTESIAN_POINT('Ctrl Pts',(-1.73550351679848,1.,-0.748582462954854));
#45178=CARTESIAN_POINT('Ctrl Pts',(-1.74080458266705,-1.,-0.75019343597954));
#45179=CARTESIAN_POINT('Ctrl Pts',(-1.74080458266705,1.,-0.75019343597954));
#45180=CARTESIAN_POINT('Ctrl Pts',(-1.74585086852298,-1.,-0.751555614163629));
#45181=CARTESIAN_POINT('Ctrl Pts',(-1.74585086852298,1.,-0.751555614163629));
#45182=CARTESIAN_POINT('Ctrl Pts',(-1.75095139468809,-1.,-0.752797683531377));
#45183=CARTESIAN_POINT('Ctrl Pts',(-1.75095139468809,1.,-0.752797683531377));
#45184=CARTESIAN_POINT('Ctrl Pts',(-1.75631083600175,-1.,-0.75400925402848));
#45185=CARTESIAN_POINT('Ctrl Pts',(-1.75631083600175,1.,-0.75400925402848));
#45186=CARTESIAN_POINT('Ctrl Pts',(-1.7619781724032,-1.,-0.755220979975262));
#45187=CARTESIAN_POINT('Ctrl Pts',(-1.7619781724032,1.,-0.755220979975262));
#45188=CARTESIAN_POINT('Ctrl Pts',(-1.76789396003141,-1.,-0.756421896028403));
#45189=CARTESIAN_POINT('Ctrl Pts',(-1.76789396003141,1.,-0.756421896028403));
#45190=CARTESIAN_POINT('Ctrl Pts',(-1.77394167108342,-1.,-0.757578264077238));
#45191=CARTESIAN_POINT('Ctrl Pts',(-1.77394167108342,1.,-0.757578264077238));
#45192=CARTESIAN_POINT('Ctrl Pts',(-1.77999411220912,-1.,-0.75865062667738));
#45193=CARTESIAN_POINT('Ctrl Pts',(-1.77999411220912,1.,-0.75865062667738));
#45194=CARTESIAN_POINT('Ctrl Pts',(-1.78596964884526,-1.,-0.759614401109868));
#45195=CARTESIAN_POINT('Ctrl Pts',(-1.78596964884526,1.,-0.759614401109868));
#45196=CARTESIAN_POINT('Ctrl Pts',(-1.79185815610802,-1.,-0.760469555880425));
#45197=CARTESIAN_POINT('Ctrl Pts',(-1.79185815610802,1.,-0.760469555880425));
#45198=CARTESIAN_POINT('Ctrl Pts',(-1.79768986997735,-1.,-0.761229695230359));
#45199=CARTESIAN_POINT('Ctrl Pts',(-1.79768986997735,1.,-0.761229695230359));
#45200=CARTESIAN_POINT('Ctrl Pts',(-1.80351583877334,-1.,-0.761915336443515));
#45201=CARTESIAN_POINT('Ctrl Pts',(-1.80351583877334,1.,-0.761915336443515));
#45202=CARTESIAN_POINT('Ctrl Pts',(-1.80938551463989,-1.,-0.762546129464036));
#45203=CARTESIAN_POINT('Ctrl Pts',(-1.80938551463989,1.,-0.762546129464036));
#45204=CARTESIAN_POINT('Ctrl Pts',(-1.81532118405566,-1.,-0.763132003836783));
#45205=CARTESIAN_POINT('Ctrl Pts',(-1.81532118405566,1.,-0.763132003836783));
#45206=CARTESIAN_POINT('Ctrl Pts',(-1.82131873145297,-1.,-0.763673465462854));
#45207=CARTESIAN_POINT('Ctrl Pts',(-1.82131873145297,1.,-0.763673465462854));
#45208=CARTESIAN_POINT('Ctrl Pts',(-1.8273599120008,-1.,-0.764165902606055));
#45209=CARTESIAN_POINT('Ctrl Pts',(-1.8273599120008,1.,-0.764165902606055));
#45210=CARTESIAN_POINT('Ctrl Pts',(-1.8334207722714,-1.,-0.764602549687845));
#45211=CARTESIAN_POINT('Ctrl Pts',(-1.8334207722714,1.,-0.764602549687845));
#45212=CARTESIAN_POINT('Ctrl Pts',(-1.83948181064823,-1.,-0.764978057881687));
#45213=CARTESIAN_POINT('Ctrl Pts',(-1.83948181064823,1.,-0.764978057881687));
#45214=CARTESIAN_POINT('Ctrl Pts',(-1.8455369887591,-1.,-0.765291664861971));
#45215=CARTESIAN_POINT('Ctrl Pts',(-1.8455369887591,1.,-0.765291664861971));
#45216=CARTESIAN_POINT('Ctrl Pts',(-1.85158945130054,-1.,-0.765545710619023));
#45217=CARTESIAN_POINT('Ctrl Pts',(-1.85158945130054,1.,-0.765545710619023));
#45218=CARTESIAN_POINT('Ctrl Pts',(-1.85764741390391,-1.,-0.765744212909305));
#45219=CARTESIAN_POINT('Ctrl Pts',(-1.85764741390391,1.,-0.765744212909305));
#45220=CARTESIAN_POINT('Ctrl Pts',(-1.86372027063314,-1.,-0.765891519092557));
#45221=CARTESIAN_POINT('Ctrl Pts',(-1.86372027063314,1.,-0.765891519092557));
#45222=CARTESIAN_POINT('Ctrl Pts',(-1.86981398314345,-1.,-0.765990708546111));
#45223=CARTESIAN_POINT('Ctrl Pts',(-1.86981398314345,1.,-0.765990708546111));
#45224=CARTESIAN_POINT('Ctrl Pts',(-1.87592888967886,-1.,-0.766042837036759));
#45225=CARTESIAN_POINT('Ctrl Pts',(-1.87592888967886,1.,-0.766042837036759));
#45226=CARTESIAN_POINT('Ctrl Pts',(-1.88206215302561,-1.,-0.766047794851868));
#45227=CARTESIAN_POINT('Ctrl Pts',(-1.88206215302561,1.,-0.766047794851868));
#45228=CARTESIAN_POINT('Ctrl Pts',(-1.88820926433409,-1.,-0.76600483706209));
#45229=CARTESIAN_POINT('Ctrl Pts',(-1.88820926433409,1.,-0.76600483706209));
#45230=CARTESIAN_POINT('Ctrl Pts',(-1.89436577771389,-1.,-0.765913193856979));
#45231=CARTESIAN_POINT('Ctrl Pts',(-1.89436577771389,1.,-0.765913193856979));
#45232=CARTESIAN_POINT('Ctrl Pts',(-1.90052930393599,-1.,-0.765772772593395));
#45233=CARTESIAN_POINT('Ctrl Pts',(-1.90052930393599,1.,-0.765772772593395));
#45234=CARTESIAN_POINT('Ctrl Pts',(-1.90669961402362,-1.,-0.765584196937936));
#45235=CARTESIAN_POINT('Ctrl Pts',(-1.90669961402362,1.,-0.765584196937936));
#45236=CARTESIAN_POINT('Ctrl Pts',(-1.91287765805174,-1.,-0.765348465884739));
#45237=CARTESIAN_POINT('Ctrl Pts',(-1.91287765805174,1.,-0.765348465884739));
#45238=CARTESIAN_POINT('Ctrl Pts',(-1.91906491634197,-1.,-0.765066729667095));
#45239=CARTESIAN_POINT('Ctrl Pts',(-1.91906491634197,1.,-0.765066729667095));
#45240=CARTESIAN_POINT('Ctrl Pts',(-1.92526263537041,-1.,-0.764740025488189));
#45241=CARTESIAN_POINT('Ctrl Pts',(-1.92526263537041,1.,-0.764740025488189));
#45242=CARTESIAN_POINT('Ctrl Pts',(-1.93147105496367,-1.,-0.764369010673889));
#45243=CARTESIAN_POINT('Ctrl Pts',(-1.93147105496367,1.,-0.764369010673889));
#45244=CARTESIAN_POINT('Ctrl Pts',(-1.93768964875867,-1.,-0.763954049121393));
#45245=CARTESIAN_POINT('Ctrl Pts',(-1.93768964875867,1.,-0.763954049121393));
#45246=CARTESIAN_POINT('Ctrl Pts',(-1.94391746617626,-1.,-0.76349533353858));
#45247=CARTESIAN_POINT('Ctrl Pts',(-1.94391746617626,1.,-0.76349533353858));
#45248=CARTESIAN_POINT('Ctrl Pts',(-1.95015342590025,-1.,-0.762992990878774));
#45249=CARTESIAN_POINT('Ctrl Pts',(-1.95015342590025,1.,-0.762992990878774));
#45250=CARTESIAN_POINT('Ctrl Pts',(-1.95639665309893,-1.,-0.762447203806263));
#45251=CARTESIAN_POINT('Ctrl Pts',(-1.95639665309893,1.,-0.762447203806263));
#45252=CARTESIAN_POINT('Ctrl Pts',(-1.96264672744229,-1.,-0.761858300014575));
#45253=CARTESIAN_POINT('Ctrl Pts',(-1.96264672744229,1.,-0.761858300014575));
#45254=CARTESIAN_POINT('Ctrl Pts',(-1.96890351582545,-1.,-0.761226690483986));
#45255=CARTESIAN_POINT('Ctrl Pts',(-1.96890351582545,1.,-0.761226690483986));
#45256=CARTESIAN_POINT('Ctrl Pts',(-1.97516705321521,-1.,-0.760552825409855));
#45257=CARTESIAN_POINT('Ctrl Pts',(-1.97516705321521,1.,-0.760552825409855));
#45258=CARTESIAN_POINT('Ctrl Pts',(-1.98143741418156,-1.,-0.759837147452135));
#45259=CARTESIAN_POINT('Ctrl Pts',(-1.98143741418156,1.,-0.759837147452135));
#45260=CARTESIAN_POINT('Ctrl Pts',(-1.98771456680806,-1.,-0.759080037802242));
#45261=CARTESIAN_POINT('Ctrl Pts',(-1.98771456680806,1.,-0.759080037802242));
#45262=CARTESIAN_POINT('Ctrl Pts',(-1.9939983109871,-1.,-0.758281796766377));
#45263=CARTESIAN_POINT('Ctrl Pts',(-1.9939983109871,1.,-0.758281796766377));
#45264=CARTESIAN_POINT('Ctrl Pts',(-2.00028834739072,-1.,-0.757442676862341));
#45265=CARTESIAN_POINT('Ctrl Pts',(-2.00028834739072,1.,-0.757442676862341));
#45266=CARTESIAN_POINT('Ctrl Pts',(-2.00658431587682,-1.,-0.756562904646496));
#45267=CARTESIAN_POINT('Ctrl Pts',(-2.00658431587682,1.,-0.756562904646496));
#45268=CARTESIAN_POINT('Ctrl Pts',(-2.01288584328149,-1.,-0.7556427049581));
#45269=CARTESIAN_POINT('Ctrl Pts',(-2.01288584328149,1.,-0.7556427049581));
#45270=CARTESIAN_POINT('Ctrl Pts',(-2.01919259406003,-1.,-0.75468233072352));
#45271=CARTESIAN_POINT('Ctrl Pts',(-2.01919259406003,1.,-0.75468233072352));
#45272=CARTESIAN_POINT('Ctrl Pts',(-2.02550428623587,-1.,-0.753682061113765));
#45273=CARTESIAN_POINT('Ctrl Pts',(-2.02550428623587,1.,-0.753682061113765));
#45274=CARTESIAN_POINT('Ctrl Pts',(-2.03182068456467,-1.,-0.752642180488104));
#45275=CARTESIAN_POINT('Ctrl Pts',(-2.03182068456467,1.,-0.752642180488104));
#45276=CARTESIAN_POINT('Ctrl Pts',(-2.03814160092173,-1.,-0.751562963361383));
#45277=CARTESIAN_POINT('Ctrl Pts',(-2.03814160092173,1.,-0.751562963361383));
#45278=CARTESIAN_POINT('Ctrl Pts',(-2.04446689147754,-1.,-0.750444657874758));
#45279=CARTESIAN_POINT('Ctrl Pts',(-2.04446689147754,1.,-0.750444657874758));
#45280=CARTESIAN_POINT('Ctrl Pts',(-2.05079645591606,-1.,-0.749287468663053));
#45281=CARTESIAN_POINT('Ctrl Pts',(-2.05079645591606,1.,-0.749287468663053));
#45282=CARTESIAN_POINT('Ctrl Pts',(-2.05713023030263,-1.,-0.748091554181101));
#45283=CARTESIAN_POINT('Ctrl Pts',(-2.05713023030263,1.,-0.748091554181101));
#45284=CARTESIAN_POINT('Ctrl Pts',(-2.06220058927162,-1.,-0.747103932785504));
#45285=CARTESIAN_POINT('Ctrl Pts',(-2.06220058927162,1.,-0.747103932785504));
#45286=CARTESIAN_POINT('Ctrl Pts',(-2.06600523016401,-1.,-0.746345871542695));
#45287=CARTESIAN_POINT('Ctrl Pts',(-2.06600523016401,1.,-0.746345871542695));
#45288=CARTESIAN_POINT('Ctrl Pts',(-2.06854248895575,-1.,-0.74583279137781));
#45289=CARTESIAN_POINT('Ctrl Pts',(-2.06854248895575,1.,-0.74583279137781));
#45290=CARTESIAN_POINT('Ctrl Pts',(-2.0698113262342,-1.,-0.745574324794401));
#45291=CARTESIAN_POINT('Ctrl Pts',(-2.0698113262342,1.,-0.745574324794401));
#45292=CARTESIAN_POINT('',(-1.60662857109684,1.,-0.693717979106306));
#45293=CARTESIAN_POINT('Ctrl Pts',(-1.60662857109684,1.,-0.693717979106306));
#45294=CARTESIAN_POINT('Ctrl Pts',(-1.61106790958151,1.,-0.695712097881194));
#45295=CARTESIAN_POINT('Ctrl Pts',(-1.61974673472612,1.,-0.699605146405088));
#45296=CARTESIAN_POINT('Ctrl Pts',(-1.63216541664676,1.,-0.705159151988319));
#45297=CARTESIAN_POINT('Ctrl Pts',(-1.64752408832016,1.,-0.711993139355394));
#45298=CARTESIAN_POINT('Ctrl Pts',(-1.6647288055568,1.,-0.719585433804282));
#45299=CARTESIAN_POINT('Ctrl Pts',(-1.67996158455503,1.,-0.726235967997433));
#45300=CARTESIAN_POINT('Ctrl Pts',(-1.69326921975743,1.,-0.731963238697195));
#45301=CARTESIAN_POINT('Ctrl Pts',(-1.70473309006121,1.,-0.736799665724771));
#45302=CARTESIAN_POINT('Ctrl Pts',(-1.71447789751927,1.,-0.740795162032087));
#45303=CARTESIAN_POINT('Ctrl Pts',(-1.7226822991693,1.,-0.744021445433764));
#45304=CARTESIAN_POINT('Ctrl Pts',(-1.72958533647399,1.,-0.746574710096436));
#45305=CARTESIAN_POINT('Ctrl Pts',(-1.73550351679848,1.,-0.748582462954854));
#45306=CARTESIAN_POINT('Ctrl Pts',(-1.74080458266705,1.,-0.75019343597954));
#45307=CARTESIAN_POINT('Ctrl Pts',(-1.74585086852298,1.,-0.751555614163629));
#45308=CARTESIAN_POINT('Ctrl Pts',(-1.75095139468809,1.,-0.752797683531377));
#45309=CARTESIAN_POINT('Ctrl Pts',(-1.75631083600175,1.,-0.75400925402848));
#45310=CARTESIAN_POINT('Ctrl Pts',(-1.7619781724032,1.,-0.755220979975262));
#45311=CARTESIAN_POINT('Ctrl Pts',(-1.76789396003141,1.,-0.756421896028403));
#45312=CARTESIAN_POINT('Ctrl Pts',(-1.77394167108342,1.,-0.757578264077238));
#45313=CARTESIAN_POINT('Ctrl Pts',(-1.77999411220912,1.,-0.75865062667738));
#45314=CARTESIAN_POINT('Ctrl Pts',(-1.78596964884526,1.,-0.759614401109868));
#45315=CARTESIAN_POINT('Ctrl Pts',(-1.79185815610802,1.,-0.760469555880425));
#45316=CARTESIAN_POINT('Ctrl Pts',(-1.79768986997735,1.,-0.761229695230359));
#45317=CARTESIAN_POINT('Ctrl Pts',(-1.80351583877334,1.,-0.761915336443515));
#45318=CARTESIAN_POINT('Ctrl Pts',(-1.80938551463989,1.,-0.762546129464036));
#45319=CARTESIAN_POINT('Ctrl Pts',(-1.81532118405566,1.,-0.763132003836783));
#45320=CARTESIAN_POINT('Ctrl Pts',(-1.82131873145297,1.,-0.763673465462854));
#45321=CARTESIAN_POINT('Ctrl Pts',(-1.8273599120008,1.,-0.764165902606055));
#45322=CARTESIAN_POINT('Ctrl Pts',(-1.8334207722714,1.,-0.764602549687845));
#45323=CARTESIAN_POINT('Ctrl Pts',(-1.83948181064823,1.,-0.764978057881687));
#45324=CARTESIAN_POINT('Ctrl Pts',(-1.8455369887591,1.,-0.765291664861971));
#45325=CARTESIAN_POINT('Ctrl Pts',(-1.85158945130054,1.,-0.765545710619023));
#45326=CARTESIAN_POINT('Ctrl Pts',(-1.85764741390391,1.,-0.765744212909305));
#45327=CARTESIAN_POINT('Ctrl Pts',(-1.86372027063314,1.,-0.765891519092557));
#45328=CARTESIAN_POINT('Ctrl Pts',(-1.86981398314345,1.,-0.765990708546111));
#45329=CARTESIAN_POINT('Ctrl Pts',(-1.87592888967886,1.,-0.766042837036759));
#45330=CARTESIAN_POINT('Ctrl Pts',(-1.88206215302561,1.,-0.766047794851868));
#45331=CARTESIAN_POINT('Ctrl Pts',(-1.88820926433409,1.,-0.76600483706209));
#45332=CARTESIAN_POINT('Ctrl Pts',(-1.89436577771389,1.,-0.765913193856979));
#45333=CARTESIAN_POINT('Ctrl Pts',(-1.90052930393599,1.,-0.765772772593395));
#45334=CARTESIAN_POINT('Ctrl Pts',(-1.90669961402362,1.,-0.765584196937936));
#45335=CARTESIAN_POINT('Ctrl Pts',(-1.91287765805174,1.,-0.765348465884739));
#45336=CARTESIAN_POINT('Ctrl Pts',(-1.91906491634197,1.,-0.765066729667095));
#45337=CARTESIAN_POINT('Ctrl Pts',(-1.92526263537041,1.,-0.764740025488189));
#45338=CARTESIAN_POINT('Ctrl Pts',(-1.93147105496367,1.,-0.764369010673889));
#45339=CARTESIAN_POINT('Ctrl Pts',(-1.93768964875867,1.,-0.763954049121393));
#45340=CARTESIAN_POINT('Ctrl Pts',(-1.94391746617626,1.,-0.76349533353858));
#45341=CARTESIAN_POINT('Ctrl Pts',(-1.95015342590025,1.,-0.762992990878774));
#45342=CARTESIAN_POINT('Ctrl Pts',(-1.95639665309893,1.,-0.762447203806263));
#45343=CARTESIAN_POINT('Ctrl Pts',(-1.96264672744229,1.,-0.761858300014575));
#45344=CARTESIAN_POINT('Ctrl Pts',(-1.96890351582545,1.,-0.761226690483986));
#45345=CARTESIAN_POINT('Ctrl Pts',(-1.97516705321521,1.,-0.760552825409855));
#45346=CARTESIAN_POINT('Ctrl Pts',(-1.98143741418156,1.,-0.759837147452135));
#45347=CARTESIAN_POINT('Ctrl Pts',(-1.98771456680806,1.,-0.759080037802242));
#45348=CARTESIAN_POINT('Ctrl Pts',(-1.9939983109871,1.,-0.758281796766377));
#45349=CARTESIAN_POINT('Ctrl Pts',(-2.00028834739072,1.,-0.757442676862341));
#45350=CARTESIAN_POINT('Ctrl Pts',(-2.00658431587682,1.,-0.756562904646496));
#45351=CARTESIAN_POINT('Ctrl Pts',(-2.01288584328149,1.,-0.7556427049581));
#45352=CARTESIAN_POINT('Ctrl Pts',(-2.01919259406003,1.,-0.75468233072352));
#45353=CARTESIAN_POINT('Ctrl Pts',(-2.02550428623587,1.,-0.753682061113765));
#45354=CARTESIAN_POINT('Ctrl Pts',(-2.03182068456467,1.,-0.752642180488104));
#45355=CARTESIAN_POINT('Ctrl Pts',(-2.03814160092173,1.,-0.751562963361383));
#45356=CARTESIAN_POINT('Ctrl Pts',(-2.04446689147754,1.,-0.750444657874758));
#45357=CARTESIAN_POINT('Ctrl Pts',(-2.05079645591606,1.,-0.749287468663053));
#45358=CARTESIAN_POINT('Ctrl Pts',(-2.05713023030263,1.,-0.748091554181101));
#45359=CARTESIAN_POINT('Ctrl Pts',(-2.06220058927162,1.,-0.747103932785504));
#45360=CARTESIAN_POINT('Ctrl Pts',(-2.06600523016401,1.,-0.746345871542695));
#45361=CARTESIAN_POINT('Ctrl Pts',(-2.06854248895575,1.,-0.74583279137781));
#45362=CARTESIAN_POINT('Ctrl Pts',(-2.0698113262342,1.,-0.745574324794401));
#45363=CARTESIAN_POINT('',(-1.60662857109684,0.,-0.693717979106306));
#45364=CARTESIAN_POINT('Origin',(0.,0.,0.));
#45365=CARTESIAN_POINT('',(-1.5055822144029,1.,-0.892032620296855));
#45366=CARTESIAN_POINT('Origin',(0.,1.,0.));
#45367=CARTESIAN_POINT('',(-1.5055822144029,0.,-0.892032620296855));
#45368=CARTESIAN_POINT('Ctrl Pts',(-1.81978687191668,-1.,-1.23627494547115));
#45369=CARTESIAN_POINT('Ctrl Pts',(-1.81978687191668,1.,-1.23627494547115));
#45370=CARTESIAN_POINT('Ctrl Pts',(-1.81925017193666,-1.,-1.23509651170476));
#45371=CARTESIAN_POINT('Ctrl Pts',(-1.81925017193666,1.,-1.23509651170476));
#45372=CARTESIAN_POINT('Ctrl Pts',(-1.81817389921279,-1.,-1.2327422452705));
#45373=CARTESIAN_POINT('Ctrl Pts',(-1.81817389921279,1.,-1.2327422452705));
#45374=CARTESIAN_POINT('Ctrl Pts',(-1.8165508718364,-1.,-1.2292186489137));
#45375=CARTESIAN_POINT('Ctrl Pts',(-1.8165508718364,1.,-1.2292186489137));
#45376=CARTESIAN_POINT('Ctrl Pts',(-1.81436959210434,-1.,-1.2245361330495));
#45377=CARTESIAN_POINT('Ctrl Pts',(-1.81436959210434,1.,-1.2245361330495));
#45378=CARTESIAN_POINT('Ctrl Pts',(-1.81161420806656,-1.,-1.21870906103557));
#45379=CARTESIAN_POINT('Ctrl Pts',(-1.81161420806656,1.,-1.21870906103557));
#45380=CARTESIAN_POINT('Ctrl Pts',(-1.80882996917129,-1.,-1.21290815708314));
#45381=CARTESIAN_POINT('Ctrl Pts',(-1.80882996917129,1.,-1.21290815708314));
#45382=CARTESIAN_POINT('Ctrl Pts',(-1.80601678480707,-1.,-1.20713356605475));
#45383=CARTESIAN_POINT('Ctrl Pts',(-1.80601678480707,1.,-1.20713356605475));
#45384=CARTESIAN_POINT('Ctrl Pts',(-1.80317454838603,-1.,-1.20138548938974));
#45385=CARTESIAN_POINT('Ctrl Pts',(-1.80317454838603,1.,-1.20138548938974));
#45386=CARTESIAN_POINT('Ctrl Pts',(-1.80030314369879,-1.,-1.19566418930242));
#45387=CARTESIAN_POINT('Ctrl Pts',(-1.80030314369879,1.,-1.19566418930242));
#45388=CARTESIAN_POINT('Ctrl Pts',(-1.79740245923478,-1.,-1.18996997934445));
#45389=CARTESIAN_POINT('Ctrl Pts',(-1.79740245923478,1.,-1.18996997934445));
#45390=CARTESIAN_POINT('Ctrl Pts',(-1.79447240321515,-1.,-1.18430321697432));
#45391=CARTESIAN_POINT('Ctrl Pts',(-1.79447240321515,1.,-1.18430321697432));
#45392=CARTESIAN_POINT('Ctrl Pts',(-1.79151291552689,-1.,-1.17866429440809));
#45393=CARTESIAN_POINT('Ctrl Pts',(-1.79151291552689,1.,-1.17866429440809));
#45394=CARTESIAN_POINT('Ctrl Pts',(-1.78852398877616,-1.,-1.17305363177328));
#45395=CARTESIAN_POINT('Ctrl Pts',(-1.78852398877616,1.,-1.17305363177328));
#45396=CARTESIAN_POINT('Ctrl Pts',(-1.78550566040443,-1.,-1.16747166312303));
#45397=CARTESIAN_POINT('Ctrl Pts',(-1.78550566040443,1.,-1.16747166312303));
#45398=CARTESIAN_POINT('Ctrl Pts',(-1.78245795881009,-1.,-1.16191881298499));
#45399=CARTESIAN_POINT('Ctrl Pts',(-1.78245795881009,1.,-1.16191881298499));
#45400=CARTESIAN_POINT('Ctrl Pts',(-1.77938085564275,-1.,-1.15639547194698));
#45401=CARTESIAN_POINT('Ctrl Pts',(-1.77938085564275,1.,-1.15639547194698));
#45402=CARTESIAN_POINT('Ctrl Pts',(-1.7762742255701,-1.,-1.15090197841515));
#45403=CARTESIAN_POINT('Ctrl Pts',(-1.7762742255701,1.,-1.15090197841515));
#45404=CARTESIAN_POINT('Ctrl Pts',(-1.77313777896194,-1.,-1.1454385822692));
#45405=CARTESIAN_POINT('Ctrl Pts',(-1.77313777896194,1.,-1.1454385822692));
#45406=CARTESIAN_POINT('Ctrl Pts',(-1.76997111386769,-1.,-1.14000548336975));
#45407=CARTESIAN_POINT('Ctrl Pts',(-1.76997111386769,1.,-1.14000548336975));
#45408=CARTESIAN_POINT('Ctrl Pts',(-1.76677384551862,-1.,-1.1346029180462));
#45409=CARTESIAN_POINT('Ctrl Pts',(-1.76677384551862,1.,-1.1346029180462));
#45410=CARTESIAN_POINT('Ctrl Pts',(-1.7635457196617,-1.,-1.12923123555075));
#45411=CARTESIAN_POINT('Ctrl Pts',(-1.7635457196617,1.,-1.12923123555075));
#45412=CARTESIAN_POINT('Ctrl Pts',(-1.76028671825096,-1.,-1.12389096855086));
#45413=CARTESIAN_POINT('Ctrl Pts',(-1.76028671825096,1.,-1.12389096855086));
#45414=CARTESIAN_POINT('Ctrl Pts',(-1.75699720772105,-1.,-1.11858293216763));
#45415=CARTESIAN_POINT('Ctrl Pts',(-1.75699720772105,1.,-1.11858293216763));
#45416=CARTESIAN_POINT('Ctrl Pts',(-1.7536777209463,-1.,-1.11330807582551));
#45417=CARTESIAN_POINT('Ctrl Pts',(-1.7536777209463,1.,-1.11330807582551));
#45418=CARTESIAN_POINT('Ctrl Pts',(-1.7503286607592,-1.,-1.10806728183007));
#45419=CARTESIAN_POINT('Ctrl Pts',(-1.7503286607592,1.,-1.10806728183007));
#45420=CARTESIAN_POINT('Ctrl Pts',(-1.74695004214923,-1.,-1.10286118991143));
#45421=CARTESIAN_POINT('Ctrl Pts',(-1.74695004214923,1.,-1.10286118991143));
#45422=CARTESIAN_POINT('Ctrl Pts',(-1.74354119236208,-1.,-1.09768999241225));
#45423=CARTESIAN_POINT('Ctrl Pts',(-1.74354119236208,1.,-1.09768999241225));
#45424=CARTESIAN_POINT('Ctrl Pts',(-1.74010053962247,-1.,-1.09255329056493));
#45425=CARTESIAN_POINT('Ctrl Pts',(-1.74010053962247,1.,-1.09255329056493));
#45426=CARTESIAN_POINT('Ctrl Pts',(-1.73662628326091,-1.,-1.08745056285427));
#45427=CARTESIAN_POINT('Ctrl Pts',(-1.73662628326091,1.,-1.08745056285427));
#45428=CARTESIAN_POINT('Ctrl Pts',(-1.73311705663407,-1.,-1.08238162784749));
#45429=CARTESIAN_POINT('Ctrl Pts',(-1.73311705663407,1.,-1.08238162784749));
#45430=CARTESIAN_POINT('Ctrl Pts',(-1.72957248977424,-1.,-1.0773470373727));
#45431=CARTESIAN_POINT('Ctrl Pts',(-1.72957248977424,1.,-1.0773470373727));
#45432=CARTESIAN_POINT('Ctrl Pts',(-1.72599406198488,-1.,-1.07234866990252));
#45433=CARTESIAN_POINT('Ctrl Pts',(-1.72599406198488,1.,-1.07234866990252));
#45434=CARTESIAN_POINT('Ctrl Pts',(-1.72238500928453,-1.,-1.06738966975462));
#45435=CARTESIAN_POINT('Ctrl Pts',(-1.72238500928453,1.,-1.06738966975462));
#45436=CARTESIAN_POINT('Ctrl Pts',(-1.71874858456904,-1.,-1.06247324680647));
#45437=CARTESIAN_POINT('Ctrl Pts',(-1.71874858456904,1.,-1.06247324680647));
#45438=CARTESIAN_POINT('Ctrl Pts',(-1.7150865442702,-1.,-1.05760163192479));
#45439=CARTESIAN_POINT('Ctrl Pts',(-1.7150865442702,1.,-1.05760163192479));
#45440=CARTESIAN_POINT('Ctrl Pts',(-1.71139783543989,-1.,-1.05277517202855));
#45441=CARTESIAN_POINT('Ctrl Pts',(-1.71139783543989,1.,-1.05277517202855));
#45442=CARTESIAN_POINT('Ctrl Pts',(-1.70767646263649,-1.,-1.04799085404995));
#45443=CARTESIAN_POINT('Ctrl Pts',(-1.70767646263649,1.,-1.04799085404995));
#45444=CARTESIAN_POINT('Ctrl Pts',(-1.70391338707982,-1.,-1.04324363334554));
#45445=CARTESIAN_POINT('Ctrl Pts',(-1.70391338707982,1.,-1.04324363334554));
#45446=CARTESIAN_POINT('Ctrl Pts',(-1.70010052930962,-1.,-1.03852922490789));
#45447=CARTESIAN_POINT('Ctrl Pts',(-1.70010052930962,1.,-1.03852922490789));
#45448=CARTESIAN_POINT('Ctrl Pts',(-1.69623414782771,-1.,-1.03384646003588));
#45449=CARTESIAN_POINT('Ctrl Pts',(-1.69623414782771,1.,-1.03384646003588));
#45450=CARTESIAN_POINT('Ctrl Pts',(-1.69231840863458,-1.,-1.02919977579147));
#45451=CARTESIAN_POINT('Ctrl Pts',(-1.69231840863458,1.,-1.02919977579147));
#45452=CARTESIAN_POINT('Ctrl Pts',(-1.68836910178447,-1.,-1.02460180535255));
#45453=CARTESIAN_POINT('Ctrl Pts',(-1.68836910178447,1.,-1.02460180535255));
#45454=CARTESIAN_POINT('Ctrl Pts',(-1.68440578021706,-1.,-1.02006795074201));
#45455=CARTESIAN_POINT('Ctrl Pts',(-1.68440578021706,1.,-1.02006795074201));
#45456=CARTESIAN_POINT('Ctrl Pts',(-1.68044289894798,-1.,-1.01561026162773));
#45457=CARTESIAN_POINT('Ctrl Pts',(-1.68044289894798,1.,-1.01561026162773));
#45458=CARTESIAN_POINT('Ctrl Pts',(-1.67648246776464,-1.,-1.01123236493511));
#45459=CARTESIAN_POINT('Ctrl Pts',(-1.67648246776464,1.,-1.01123236493511));
#45460=CARTESIAN_POINT('Ctrl Pts',(-1.67250335383293,-1.,-1.00692206696414));
#45461=CARTESIAN_POINT('Ctrl Pts',(-1.67250335383293,1.,-1.00692206696414));
#45462=CARTESIAN_POINT('Ctrl Pts',(-1.66846059277303,-1.,-1.00265091003727));
#45463=CARTESIAN_POINT('Ctrl Pts',(-1.66846059277303,1.,-1.00265091003727));
#45464=CARTESIAN_POINT('Ctrl Pts',(-1.66430758030376,-1.,-0.998389654952758));
#45465=CARTESIAN_POINT('Ctrl Pts',(-1.66430758030376,1.,-0.998389654952758));
#45466=CARTESIAN_POINT('Ctrl Pts',(-1.66001553809947,-1.,-0.994121836661306));
#45467=CARTESIAN_POINT('Ctrl Pts',(-1.66001553809947,1.,-0.994121836661306));
#45468=CARTESIAN_POINT('Ctrl Pts',(-1.65559044289699,-1.,-0.989855627854165));
#45469=CARTESIAN_POINT('Ctrl Pts',(-1.65559044289699,1.,-0.989855627854165));
#45470=CARTESIAN_POINT('Ctrl Pts',(-1.65110016612638,-1.,-0.985642622920821));
#45471=CARTESIAN_POINT('Ctrl Pts',(-1.65110016612638,1.,-0.985642622920821));
#45472=CARTESIAN_POINT('Ctrl Pts',(-1.64665139190656,-1.,-0.981562530939489));
#45473=CARTESIAN_POINT('Ctrl Pts',(-1.64665139190656,1.,-0.981562530939489));
#45474=CARTESIAN_POINT('Ctrl Pts',(-1.64233990826687,-1.,-0.977689794119416));
#45475=CARTESIAN_POINT('Ctrl Pts',(-1.64233990826687,1.,-0.977689794119416));
#45476=CARTESIAN_POINT('Ctrl Pts',(-1.63820952658144,-1.,-0.974066058287418));
#45477=CARTESIAN_POINT('Ctrl Pts',(-1.63820952658144,1.,-0.974066058287418));
#45478=CARTESIAN_POINT('Ctrl Pts',(-1.63420665729798,-1.,-0.970669715997509));
#45479=CARTESIAN_POINT('Ctrl Pts',(-1.63420665729798,1.,-0.970669715997509));
#45480=CARTESIAN_POINT('Ctrl Pts',(-1.63013849959461,-1.,-0.967387853230345));
#45481=CARTESIAN_POINT('Ctrl Pts',(-1.63013849959461,1.,-0.967387853230345));
#45482=CARTESIAN_POINT('Ctrl Pts',(-1.62571930670187,-1.,-0.964046107040536));
#45483=CARTESIAN_POINT('Ctrl Pts',(-1.62571930670187,1.,-0.964046107040536));
#45484=CARTESIAN_POINT('Ctrl Pts',(-1.62061638140221,-1.,-0.960438326101729));
#45485=CARTESIAN_POINT('Ctrl Pts',(-1.62061638140221,1.,-0.960438326101729));
#45486=CARTESIAN_POINT('Ctrl Pts',(-1.61449324337085,-1.,-0.956354422920671));
#45487=CARTESIAN_POINT('Ctrl Pts',(-1.61449324337085,1.,-0.956354422920671));
#45488=CARTESIAN_POINT('Ctrl Pts',(-1.60706069896936,-1.,-0.951613284356035));
#45489=CARTESIAN_POINT('Ctrl Pts',(-1.60706069896936,1.,-0.951613284356035));
#45490=CARTESIAN_POINT('Ctrl Pts',(-1.59810042043673,-1.,-0.946078063315257));
#45491=CARTESIAN_POINT('Ctrl Pts',(-1.59810042043673,1.,-0.946078063315257));
#45492=CARTESIAN_POINT('Ctrl Pts',(-1.58744937487176,-1.,-0.939646377893399));
#45493=CARTESIAN_POINT('Ctrl Pts',(-1.58744937487176,1.,-0.939646377893399));
#45494=CARTESIAN_POINT('Ctrl Pts',(-1.57499388382243,-1.,-0.932246680108685));
#45495=CARTESIAN_POINT('Ctrl Pts',(-1.57499388382243,1.,-0.932246680108685));
#45496=CARTESIAN_POINT('Ctrl Pts',(-1.56065988578893,-1.,-0.923832188944341));
#45497=CARTESIAN_POINT('Ctrl Pts',(-1.56065988578893,1.,-0.923832188944341));
#45498=CARTESIAN_POINT('Ctrl Pts',(-1.54440491149498,-1.,-0.914375919026456));
#45499=CARTESIAN_POINT('Ctrl Pts',(-1.54440491149498,1.,-0.914375919026456));
#45500=CARTESIAN_POINT('Ctrl Pts',(-1.52984849887993,-1.,-0.905967409625651));
#45501=CARTESIAN_POINT('Ctrl Pts',(-1.52984849887993,1.,-0.905967409625651));
#45502=CARTESIAN_POINT('Ctrl Pts',(-1.51805569590094,-1.,-0.899185047483511));
#45503=CARTESIAN_POINT('Ctrl Pts',(-1.51805569590094,1.,-0.899185047483511));
#45504=CARTESIAN_POINT('Ctrl Pts',(-1.50980486806688,-1.,-0.894452006964543));
#45505=CARTESIAN_POINT('Ctrl Pts',(-1.50980486806688,1.,-0.894452006964543));
#45506=CARTESIAN_POINT('Ctrl Pts',(-1.5055822144029,-1.,-0.892032620296855));
#45507=CARTESIAN_POINT('Ctrl Pts',(-1.5055822144029,1.,-0.892032620296855));
#45508=CARTESIAN_POINT('',(-1.81978687191668,1.,-1.23627494547115));
#45509=CARTESIAN_POINT('Ctrl Pts',(-1.81978687191668,1.,-1.23627494547115));
#45510=CARTESIAN_POINT('Ctrl Pts',(-1.81925017193666,1.,-1.23509651170476));
#45511=CARTESIAN_POINT('Ctrl Pts',(-1.81817389921279,1.,-1.2327422452705));
#45512=CARTESIAN_POINT('Ctrl Pts',(-1.8165508718364,1.,-1.2292186489137));
#45513=CARTESIAN_POINT('Ctrl Pts',(-1.81436959210434,1.,-1.2245361330495));
#45514=CARTESIAN_POINT('Ctrl Pts',(-1.81161420806656,1.,-1.21870906103557));
#45515=CARTESIAN_POINT('Ctrl Pts',(-1.80882996917129,1.,-1.21290815708314));
#45516=CARTESIAN_POINT('Ctrl Pts',(-1.80601678480707,1.,-1.20713356605475));
#45517=CARTESIAN_POINT('Ctrl Pts',(-1.80317454838603,1.,-1.20138548938974));
#45518=CARTESIAN_POINT('Ctrl Pts',(-1.80030314369879,1.,-1.19566418930242));
#45519=CARTESIAN_POINT('Ctrl Pts',(-1.79740245923478,1.,-1.18996997934445));
#45520=CARTESIAN_POINT('Ctrl Pts',(-1.79447240321515,1.,-1.18430321697432));
#45521=CARTESIAN_POINT('Ctrl Pts',(-1.79151291552689,1.,-1.17866429440809));
#45522=CARTESIAN_POINT('Ctrl Pts',(-1.78852398877616,1.,-1.17305363177328));
#45523=CARTESIAN_POINT('Ctrl Pts',(-1.78550566040443,1.,-1.16747166312303));
#45524=CARTESIAN_POINT('Ctrl Pts',(-1.78245795881009,1.,-1.16191881298499));
#45525=CARTESIAN_POINT('Ctrl Pts',(-1.77938085564275,1.,-1.15639547194698));
#45526=CARTESIAN_POINT('Ctrl Pts',(-1.7762742255701,1.,-1.15090197841515));
#45527=CARTESIAN_POINT('Ctrl Pts',(-1.77313777896194,1.,-1.1454385822692));
#45528=CARTESIAN_POINT('Ctrl Pts',(-1.76997111386769,1.,-1.14000548336975));
#45529=CARTESIAN_POINT('Ctrl Pts',(-1.76677384551862,1.,-1.1346029180462));
#45530=CARTESIAN_POINT('Ctrl Pts',(-1.7635457196617,1.,-1.12923123555075));
#45531=CARTESIAN_POINT('Ctrl Pts',(-1.76028671825096,1.,-1.12389096855086));
#45532=CARTESIAN_POINT('Ctrl Pts',(-1.75699720772105,1.,-1.11858293216763));
#45533=CARTESIAN_POINT('Ctrl Pts',(-1.7536777209463,1.,-1.11330807582551));
#45534=CARTESIAN_POINT('Ctrl Pts',(-1.7503286607592,1.,-1.10806728183007));
#45535=CARTESIAN_POINT('Ctrl Pts',(-1.74695004214923,1.,-1.10286118991143));
#45536=CARTESIAN_POINT('Ctrl Pts',(-1.74354119236208,1.,-1.09768999241225));
#45537=CARTESIAN_POINT('Ctrl Pts',(-1.74010053962247,1.,-1.09255329056493));
#45538=CARTESIAN_POINT('Ctrl Pts',(-1.73662628326091,1.,-1.08745056285427));
#45539=CARTESIAN_POINT('Ctrl Pts',(-1.73311705663407,1.,-1.08238162784749));
#45540=CARTESIAN_POINT('Ctrl Pts',(-1.72957248977424,1.,-1.0773470373727));
#45541=CARTESIAN_POINT('Ctrl Pts',(-1.72599406198488,1.,-1.07234866990252));
#45542=CARTESIAN_POINT('Ctrl Pts',(-1.72238500928453,1.,-1.06738966975462));
#45543=CARTESIAN_POINT('Ctrl Pts',(-1.71874858456904,1.,-1.06247324680647));
#45544=CARTESIAN_POINT('Ctrl Pts',(-1.7150865442702,1.,-1.05760163192479));
#45545=CARTESIAN_POINT('Ctrl Pts',(-1.71139783543989,1.,-1.05277517202855));
#45546=CARTESIAN_POINT('Ctrl Pts',(-1.70767646263649,1.,-1.04799085404995));
#45547=CARTESIAN_POINT('Ctrl Pts',(-1.70391338707982,1.,-1.04324363334554));
#45548=CARTESIAN_POINT('Ctrl Pts',(-1.70010052930962,1.,-1.03852922490789));
#45549=CARTESIAN_POINT('Ctrl Pts',(-1.69623414782771,1.,-1.03384646003588));
#45550=CARTESIAN_POINT('Ctrl Pts',(-1.69231840863458,1.,-1.02919977579147));
#45551=CARTESIAN_POINT('Ctrl Pts',(-1.68836910178447,1.,-1.02460180535255));
#45552=CARTESIAN_POINT('Ctrl Pts',(-1.68440578021706,1.,-1.02006795074201));
#45553=CARTESIAN_POINT('Ctrl Pts',(-1.68044289894798,1.,-1.01561026162773));
#45554=CARTESIAN_POINT('Ctrl Pts',(-1.67648246776464,1.,-1.01123236493511));
#45555=CARTESIAN_POINT('Ctrl Pts',(-1.67250335383293,1.,-1.00692206696414));
#45556=CARTESIAN_POINT('Ctrl Pts',(-1.66846059277303,1.,-1.00265091003727));
#45557=CARTESIAN_POINT('Ctrl Pts',(-1.66430758030376,1.,-0.998389654952758));
#45558=CARTESIAN_POINT('Ctrl Pts',(-1.66001553809947,1.,-0.994121836661306));
#45559=CARTESIAN_POINT('Ctrl Pts',(-1.65559044289699,1.,-0.989855627854165));
#45560=CARTESIAN_POINT('Ctrl Pts',(-1.65110016612638,1.,-0.985642622920821));
#45561=CARTESIAN_POINT('Ctrl Pts',(-1.64665139190656,1.,-0.981562530939489));
#45562=CARTESIAN_POINT('Ctrl Pts',(-1.64233990826687,1.,-0.977689794119416));
#45563=CARTESIAN_POINT('Ctrl Pts',(-1.63820952658144,1.,-0.974066058287418));
#45564=CARTESIAN_POINT('Ctrl Pts',(-1.63420665729798,1.,-0.970669715997509));
#45565=CARTESIAN_POINT('Ctrl Pts',(-1.63013849959461,1.,-0.967387853230345));
#45566=CARTESIAN_POINT('Ctrl Pts',(-1.62571930670187,1.,-0.964046107040536));
#45567=CARTESIAN_POINT('Ctrl Pts',(-1.62061638140221,1.,-0.960438326101729));
#45568=CARTESIAN_POINT('Ctrl Pts',(-1.61449324337085,1.,-0.956354422920671));
#45569=CARTESIAN_POINT('Ctrl Pts',(-1.60706069896936,1.,-0.951613284356035));
#45570=CARTESIAN_POINT('Ctrl Pts',(-1.59810042043673,1.,-0.946078063315257));
#45571=CARTESIAN_POINT('Ctrl Pts',(-1.58744937487176,1.,-0.939646377893399));
#45572=CARTESIAN_POINT('Ctrl Pts',(-1.57499388382243,1.,-0.932246680108685));
#45573=CARTESIAN_POINT('Ctrl Pts',(-1.56065988578893,1.,-0.923832188944341));
#45574=CARTESIAN_POINT('Ctrl Pts',(-1.54440491149498,1.,-0.914375919026456));
#45575=CARTESIAN_POINT('Ctrl Pts',(-1.52984849887993,1.,-0.905967409625651));
#45576=CARTESIAN_POINT('Ctrl Pts',(-1.51805569590094,1.,-0.899185047483511));
#45577=CARTESIAN_POINT('Ctrl Pts',(-1.50980486806688,1.,-0.894452006964543));
#45578=CARTESIAN_POINT('Ctrl Pts',(-1.5055822144029,1.,-0.892032620296855));
#45579=CARTESIAN_POINT('',(-1.81978687191668,0.,-1.23627494547115));
#45580=CARTESIAN_POINT('Origin',(-1.73811241238545,0.,-1.34869019493419));
#45581=CARTESIAN_POINT('',(-1.73811241238545,1.,-1.34869019493419));
#45582=CARTESIAN_POINT('',(-1.81978687191668,1.,-1.23627494547115));
#45583=CARTESIAN_POINT('',(-1.73811241238545,0.,-1.34869019493419));
#45584=CARTESIAN_POINT('Ctrl Pts',(-1.31362392696032,-1.,-1.15624053661742));
#45585=CARTESIAN_POINT('Ctrl Pts',(-1.31362392696032,1.,-1.15624053661742));
#45586=CARTESIAN_POINT('Ctrl Pts',(-1.31722977216397,-1.,-1.15950888730809));
#45587=CARTESIAN_POINT('Ctrl Pts',(-1.31722977216397,1.,-1.15950888730809));
#45588=CARTESIAN_POINT('Ctrl Pts',(-1.32428080721772,-1.,-1.16589330093588));
#45589=CARTESIAN_POINT('Ctrl Pts',(-1.32428080721772,1.,-1.16589330093588));
#45590=CARTESIAN_POINT('Ctrl Pts',(-1.33437539347008,-1.,-1.17501305789857));
#45591=CARTESIAN_POINT('Ctrl Pts',(-1.33437539347008,1.,-1.17501305789857));
#45592=CARTESIAN_POINT('Ctrl Pts',(-1.34687054001093,-1.,-1.18625865667441));
#45593=CARTESIAN_POINT('Ctrl Pts',(-1.34687054001093,1.,-1.18625865667441));
#45594=CARTESIAN_POINT('Ctrl Pts',(-1.36088705043885,-1.,-1.1987959077932));
#45595=CARTESIAN_POINT('Ctrl Pts',(-1.36088705043885,1.,-1.1987959077932));
#45596=CARTESIAN_POINT('Ctrl Pts',(-1.37331915607905,-1.,-1.20982812925645));
#45597=CARTESIAN_POINT('Ctrl Pts',(-1.37331915607905,1.,-1.20982812925645));
#45598=CARTESIAN_POINT('Ctrl Pts',(-1.38420564527715,-1.,-1.21938737280852));
#45599=CARTESIAN_POINT('Ctrl Pts',(-1.38420564527715,1.,-1.21938737280852));
#45600=CARTESIAN_POINT('Ctrl Pts',(-1.39361389568796,-1.,-1.22752961899387));
#45601=CARTESIAN_POINT('Ctrl Pts',(-1.39361389568796,1.,-1.22752961899387));
#45602=CARTESIAN_POINT('Ctrl Pts',(-1.40164708206106,-1.,-1.23434087290423));
#45603=CARTESIAN_POINT('Ctrl Pts',(-1.40164708206106,1.,-1.23434087290423));
#45604=CARTESIAN_POINT('Ctrl Pts',(-1.40845295531283,-1.,-1.23994455029534));
#45605=CARTESIAN_POINT('Ctrl Pts',(-1.40845295531283,1.,-1.23994455029534));
#45606=CARTESIAN_POINT('Ctrl Pts',(-1.41422913175179,-1.,-1.24450600513056));
#45607=CARTESIAN_POINT('Ctrl Pts',(-1.41422913175179,1.,-1.24450600513056));
#45608=CARTESIAN_POINT('Ctrl Pts',(-1.41923722596025,-1.,-1.24824430986571));
#45609=CARTESIAN_POINT('Ctrl Pts',(-1.41923722596025,1.,-1.24824430986571));
#45610=CARTESIAN_POINT('Ctrl Pts',(-1.42378102115575,-1.,-1.2514145557001));
#45611=CARTESIAN_POINT('Ctrl Pts',(-1.42378102115575,1.,-1.2514145557001));
#45612=CARTESIAN_POINT('Ctrl Pts',(-1.42815938799387,-1.,-1.25426945222639));
#45613=CARTESIAN_POINT('Ctrl Pts',(-1.42815938799387,1.,-1.25426945222639));
#45614=CARTESIAN_POINT('Ctrl Pts',(-1.43262645609691,-1.,-1.25702687965755));
#45615=CARTESIAN_POINT('Ctrl Pts',(-1.43262645609691,1.,-1.25702687965755));
#45616=CARTESIAN_POINT('Ctrl Pts',(-1.43734919180848,-1.,-1.25983531012005));
#45617=CARTESIAN_POINT('Ctrl Pts',(-1.43734919180848,1.,-1.25983531012005));
#45618=CARTESIAN_POINT('Ctrl Pts',(-1.44236470511303,-1.,-1.26273903323859));
#45619=CARTESIAN_POINT('Ctrl Pts',(-1.44236470511303,1.,-1.26273903323859));
#45620=CARTESIAN_POINT('Ctrl Pts',(-1.44761985001662,-1.,-1.26570925118868));
#45621=CARTESIAN_POINT('Ctrl Pts',(-1.44761985001662,1.,-1.26570925118868));
#45622=CARTESIAN_POINT('Ctrl Pts',(-1.45301422764247,-1.,-1.2686778680489));
#45623=CARTESIAN_POINT('Ctrl Pts',(-1.45301422764247,1.,-1.2686778680489));
#45624=CARTESIAN_POINT('Ctrl Pts',(-1.45843906294697,-1.,-1.27156805265289));
#45625=CARTESIAN_POINT('Ctrl Pts',(-1.45843906294697,1.,-1.27156805265289));
#45626=CARTESIAN_POINT('Ctrl Pts',(-1.46382431332476,-1.,-1.27433119897822));
#45627=CARTESIAN_POINT('Ctrl Pts',(-1.46382431332476,1.,-1.27433119897822));
#45628=CARTESIAN_POINT('Ctrl Pts',(-1.46916035917133,-1.,-1.27696414831089));
#45629=CARTESIAN_POINT('Ctrl Pts',(-1.46916035917133,1.,-1.27696414831089));
#45630=CARTESIAN_POINT('Ctrl Pts',(-1.4744717526707,-1.,-1.2794891824849));
#45631=CARTESIAN_POINT('Ctrl Pts',(-1.4744717526707,1.,-1.2794891824849));
#45632=CARTESIAN_POINT('Ctrl Pts',(-1.47980070347095,-1.,-1.28194158939517));
#45633=CARTESIAN_POINT('Ctrl Pts',(-1.47980070347095,1.,-1.28194158939517));
#45634=CARTESIAN_POINT('Ctrl Pts',(-1.4851881711891,-1.,-1.28435533880201));
#45635=CARTESIAN_POINT('Ctrl Pts',(-1.4851881711891,1.,-1.28435533880201));
#45636=CARTESIAN_POINT('Ctrl Pts',(-1.4906522831278,-1.,-1.2867467611644));
#45637=CARTESIAN_POINT('Ctrl Pts',(-1.4906522831278,1.,-1.2867467611644));
#45638=CARTESIAN_POINT('Ctrl Pts',(-1.49618896881754,-1.,-1.28911506584254));
#45639=CARTESIAN_POINT('Ctrl Pts',(-1.49618896881754,1.,-1.28911506584254));
#45640=CARTESIAN_POINT('Ctrl Pts',(-1.50178230149776,-1.,-1.29145022885181));
#45641=CARTESIAN_POINT('Ctrl Pts',(-1.50178230149776,1.,-1.29145022885181));
#45642=CARTESIAN_POINT('Ctrl Pts',(-1.50741159078365,-1.,-1.29373841372842));
#45643=CARTESIAN_POINT('Ctrl Pts',(-1.50741159078365,1.,-1.29373841372842));
#45644=CARTESIAN_POINT('Ctrl Pts',(-1.51305994241402,-1.,-1.29596850710509));
#45645=CARTESIAN_POINT('Ctrl Pts',(-1.51305994241402,1.,-1.29596850710509));
#45646=CARTESIAN_POINT('Ctrl Pts',(-1.51872184912724,-1.,-1.29813791800747));
#45647=CARTESIAN_POINT('Ctrl Pts',(-1.51872184912724,1.,-1.29813791800747));
#45648=CARTESIAN_POINT('Ctrl Pts',(-1.52439957861062,-1.,-1.30024984366328));
#45649=CARTESIAN_POINT('Ctrl Pts',(-1.52439957861062,1.,-1.30024984366328));
#45650=CARTESIAN_POINT('Ctrl Pts',(-1.53009970283891,-1.,-1.30231064395568));
#45651=CARTESIAN_POINT('Ctrl Pts',(-1.53009970283891,1.,-1.30231064395568));
#45652=CARTESIAN_POINT('Ctrl Pts',(-1.53582981268977,-1.,-1.30432735639489));
#45653=CARTESIAN_POINT('Ctrl Pts',(-1.53582981268977,1.,-1.30432735639489));
#45654=CARTESIAN_POINT('Ctrl Pts',(-1.54159462645432,-1.,-1.30630475189556));
#45655=CARTESIAN_POINT('Ctrl Pts',(-1.54159462645432,1.,-1.30630475189556));
#45656=CARTESIAN_POINT('Ctrl Pts',(-1.54739413957185,-1.,-1.30824393907473));
#45657=CARTESIAN_POINT('Ctrl Pts',(-1.54739413957185,1.,-1.30824393907473));
#45658=CARTESIAN_POINT('Ctrl Pts',(-1.55322568759481,-1.,-1.31014393684222));
#45659=CARTESIAN_POINT('Ctrl Pts',(-1.55322568759481,1.,-1.31014393684222));
#45660=CARTESIAN_POINT('Ctrl Pts',(-1.55908521254821,-1.,-1.31200264341696));
#45661=CARTESIAN_POINT('Ctrl Pts',(-1.55908521254821,1.,-1.31200264341696));
#45662=CARTESIAN_POINT('Ctrl Pts',(-1.56496872402353,-1.,-1.31381795281002));
#45663=CARTESIAN_POINT('Ctrl Pts',(-1.56496872402353,1.,-1.31381795281002));
#45664=CARTESIAN_POINT('Ctrl Pts',(-1.57087397835723,-1.,-1.31558903860016));
#45665=CARTESIAN_POINT('Ctrl Pts',(-1.57087397835723,1.,-1.31558903860016));
#45666=CARTESIAN_POINT('Ctrl Pts',(-1.5768005650559,-1.,-1.31731642317187));
#45667=CARTESIAN_POINT('Ctrl Pts',(-1.5768005650559,1.,-1.31731642317187));
#45668=CARTESIAN_POINT('Ctrl Pts',(-1.58274907898834,-1.,-1.31900135021432));
#45669=CARTESIAN_POINT('Ctrl Pts',(-1.58274907898834,1.,-1.31900135021432));
#45670=CARTESIAN_POINT('Ctrl Pts',(-1.58872057258245,-1.,-1.32064537110892));
#45671=CARTESIAN_POINT('Ctrl Pts',(-1.58872057258245,1.,-1.32064537110892));
#45672=CARTESIAN_POINT('Ctrl Pts',(-1.59471591079403,-1.,-1.32224985747682));
#45673=CARTESIAN_POINT('Ctrl Pts',(-1.59471591079403,1.,-1.32224985747682));
#45674=CARTESIAN_POINT('Ctrl Pts',(-1.60073511858687,-1.,-1.32381550858256));
#45675=CARTESIAN_POINT('Ctrl Pts',(-1.60073511858687,1.,-1.32381550858256));
#45676=CARTESIAN_POINT('Ctrl Pts',(-1.60677758290954,-1.,-1.32534250785782));
#45677=CARTESIAN_POINT('Ctrl Pts',(-1.60677758290954,1.,-1.32534250785782));
#45678=CARTESIAN_POINT('Ctrl Pts',(-1.6128423401575,-1.,-1.32683074483356));
#45679=CARTESIAN_POINT('Ctrl Pts',(-1.6128423401575,1.,-1.32683074483356));
#45680=CARTESIAN_POINT('Ctrl Pts',(-1.61892832270724,-1.,-1.32828000610449));
#45681=CARTESIAN_POINT('Ctrl Pts',(-1.61892832270724,1.,-1.32828000610449));
#45682=CARTESIAN_POINT('Ctrl Pts',(-1.62503464209797,-1.,-1.3296901950568));
#45683=CARTESIAN_POINT('Ctrl Pts',(-1.62503464209797,1.,-1.3296901950568));
#45684=CARTESIAN_POINT('Ctrl Pts',(-1.63116079730923,-1.,-1.33106149345645));
#45685=CARTESIAN_POINT('Ctrl Pts',(-1.63116079730923,1.,-1.33106149345645));
#45686=CARTESIAN_POINT('Ctrl Pts',(-1.63730653475089,-1.,-1.33239425103724));
#45687=CARTESIAN_POINT('Ctrl Pts',(-1.63730653475089,1.,-1.33239425103724));
#45688=CARTESIAN_POINT('Ctrl Pts',(-1.6434717485603,-1.,-1.33368890676572));
#45689=CARTESIAN_POINT('Ctrl Pts',(-1.6434717485603,1.,-1.33368890676572));
#45690=CARTESIAN_POINT('Ctrl Pts',(-1.6496563728683,-1.,-1.33494590467993));
#45691=CARTESIAN_POINT('Ctrl Pts',(-1.6496563728683,1.,-1.33494590467993));
#45692=CARTESIAN_POINT('Ctrl Pts',(-1.65586025952593,-1.,-1.33616559745172));
#45693=CARTESIAN_POINT('Ctrl Pts',(-1.65586025952593,1.,-1.33616559745172));
#45694=CARTESIAN_POINT('Ctrl Pts',(-1.66208312541983,-1.,-1.33734820885262));
#45695=CARTESIAN_POINT('Ctrl Pts',(-1.66208312541983,1.,-1.33734820885262));
#45696=CARTESIAN_POINT('Ctrl Pts',(-1.66832460783989,-1.,-1.33849388654388));
#45697=CARTESIAN_POINT('Ctrl Pts',(-1.66832460783989,1.,-1.33849388654388));
#45698=CARTESIAN_POINT('Ctrl Pts',(-1.67458429426086,-1.,-1.3396027347034));
#45699=CARTESIAN_POINT('Ctrl Pts',(-1.67458429426086,1.,-1.3396027347034));
#45700=CARTESIAN_POINT('Ctrl Pts',(-1.68086176030362,-1.,-1.34067485185203));
#45701=CARTESIAN_POINT('Ctrl Pts',(-1.68086176030362,1.,-1.34067485185203));
#45702=CARTESIAN_POINT('Ctrl Pts',(-1.68715660868764,-1.,-1.341710374848));
#45703=CARTESIAN_POINT('Ctrl Pts',(-1.68715660868764,1.,-1.341710374848));
#45704=CARTESIAN_POINT('Ctrl Pts',(-1.6934684849687,-1.,-1.34270948206319));
#45705=CARTESIAN_POINT('Ctrl Pts',(-1.6934684849687,1.,-1.34270948206319));
#45706=CARTESIAN_POINT('Ctrl Pts',(-1.69979707754427,-1.,-1.34367237124483));
#45707=CARTESIAN_POINT('Ctrl Pts',(-1.69979707754427,1.,-1.34367237124483));
#45708=CARTESIAN_POINT('Ctrl Pts',(-1.70614212266738,-1.,-1.34459924533831));
#45709=CARTESIAN_POINT('Ctrl Pts',(-1.70614212266738,1.,-1.34459924533831));
#45710=CARTESIAN_POINT('Ctrl Pts',(-1.71250340686822,-1.,-1.34549029589416));
#45711=CARTESIAN_POINT('Ctrl Pts',(-1.71250340686822,1.,-1.34549029589416));
#45712=CARTESIAN_POINT('Ctrl Pts',(-1.7188807715049,-1.,-1.34634568653227));
#45713=CARTESIAN_POINT('Ctrl Pts',(-1.7188807715049,1.,-1.34634568653227));
#45714=CARTESIAN_POINT('Ctrl Pts',(-1.72527410680674,-1.,-1.34716554819527));
#45715=CARTESIAN_POINT('Ctrl Pts',(-1.72527410680674,1.,-1.34716554819527));
#45716=CARTESIAN_POINT('Ctrl Pts',(-1.7304014965394,-1.,-1.34779309152035));
#45717=CARTESIAN_POINT('Ctrl Pts',(-1.7304014965394,1.,-1.34779309152035));
#45718=CARTESIAN_POINT('Ctrl Pts',(-1.73425417885907,-1.,-1.34824783112887));
#45719=CARTESIAN_POINT('Ctrl Pts',(-1.73425417885907,1.,-1.34824783112887));
#45720=CARTESIAN_POINT('Ctrl Pts',(-1.73682580585691,-1.,-1.34854391898045));
#45721=CARTESIAN_POINT('Ctrl Pts',(-1.73682580585691,1.,-1.34854391898045));
#45722=CARTESIAN_POINT('Ctrl Pts',(-1.73811241238545,-1.,-1.34869019493419));
#45723=CARTESIAN_POINT('Ctrl Pts',(-1.73811241238545,1.,-1.34869019493419));
#45724=CARTESIAN_POINT('',(-1.31362392696032,1.,-1.15624053661742));
#45725=CARTESIAN_POINT('Ctrl Pts',(-1.31362392696032,1.,-1.15624053661742));
#45726=CARTESIAN_POINT('Ctrl Pts',(-1.31722977216397,1.,-1.15950888730809));
#45727=CARTESIAN_POINT('Ctrl Pts',(-1.32428080721772,1.,-1.16589330093588));
#45728=CARTESIAN_POINT('Ctrl Pts',(-1.33437539347008,1.,-1.17501305789857));
#45729=CARTESIAN_POINT('Ctrl Pts',(-1.34687054001093,1.,-1.18625865667441));
#45730=CARTESIAN_POINT('Ctrl Pts',(-1.36088705043885,1.,-1.1987959077932));
#45731=CARTESIAN_POINT('Ctrl Pts',(-1.37331915607905,1.,-1.20982812925645));
#45732=CARTESIAN_POINT('Ctrl Pts',(-1.38420564527715,1.,-1.21938737280852));
#45733=CARTESIAN_POINT('Ctrl Pts',(-1.39361389568796,1.,-1.22752961899387));
#45734=CARTESIAN_POINT('Ctrl Pts',(-1.40164708206106,1.,-1.23434087290423));
#45735=CARTESIAN_POINT('Ctrl Pts',(-1.40845295531283,1.,-1.23994455029534));
#45736=CARTESIAN_POINT('Ctrl Pts',(-1.41422913175179,1.,-1.24450600513056));
#45737=CARTESIAN_POINT('Ctrl Pts',(-1.41923722596025,1.,-1.24824430986571));
#45738=CARTESIAN_POINT('Ctrl Pts',(-1.42378102115575,1.,-1.2514145557001));
#45739=CARTESIAN_POINT('Ctrl Pts',(-1.42815938799387,1.,-1.25426945222639));
#45740=CARTESIAN_POINT('Ctrl Pts',(-1.43262645609691,1.,-1.25702687965755));
#45741=CARTESIAN_POINT('Ctrl Pts',(-1.43734919180848,1.,-1.25983531012005));
#45742=CARTESIAN_POINT('Ctrl Pts',(-1.44236470511303,1.,-1.26273903323859));
#45743=CARTESIAN_POINT('Ctrl Pts',(-1.44761985001662,1.,-1.26570925118868));
#45744=CARTESIAN_POINT('Ctrl Pts',(-1.45301422764247,1.,-1.2686778680489));
#45745=CARTESIAN_POINT('Ctrl Pts',(-1.45843906294697,1.,-1.27156805265289));
#45746=CARTESIAN_POINT('Ctrl Pts',(-1.46382431332476,1.,-1.27433119897822));
#45747=CARTESIAN_POINT('Ctrl Pts',(-1.46916035917133,1.,-1.27696414831089));
#45748=CARTESIAN_POINT('Ctrl Pts',(-1.4744717526707,1.,-1.2794891824849));
#45749=CARTESIAN_POINT('Ctrl Pts',(-1.47980070347095,1.,-1.28194158939517));
#45750=CARTESIAN_POINT('Ctrl Pts',(-1.4851881711891,1.,-1.28435533880201));
#45751=CARTESIAN_POINT('Ctrl Pts',(-1.4906522831278,1.,-1.2867467611644));
#45752=CARTESIAN_POINT('Ctrl Pts',(-1.49618896881754,1.,-1.28911506584254));
#45753=CARTESIAN_POINT('Ctrl Pts',(-1.50178230149776,1.,-1.29145022885181));
#45754=CARTESIAN_POINT('Ctrl Pts',(-1.50741159078365,1.,-1.29373841372842));
#45755=CARTESIAN_POINT('Ctrl Pts',(-1.51305994241402,1.,-1.29596850710509));
#45756=CARTESIAN_POINT('Ctrl Pts',(-1.51872184912724,1.,-1.29813791800747));
#45757=CARTESIAN_POINT('Ctrl Pts',(-1.52439957861062,1.,-1.30024984366328));
#45758=CARTESIAN_POINT('Ctrl Pts',(-1.53009970283891,1.,-1.30231064395568));
#45759=CARTESIAN_POINT('Ctrl Pts',(-1.53582981268977,1.,-1.30432735639489));
#45760=CARTESIAN_POINT('Ctrl Pts',(-1.54159462645432,1.,-1.30630475189556));
#45761=CARTESIAN_POINT('Ctrl Pts',(-1.54739413957185,1.,-1.30824393907473));
#45762=CARTESIAN_POINT('Ctrl Pts',(-1.55322568759481,1.,-1.31014393684222));
#45763=CARTESIAN_POINT('Ctrl Pts',(-1.55908521254821,1.,-1.31200264341696));
#45764=CARTESIAN_POINT('Ctrl Pts',(-1.56496872402353,1.,-1.31381795281002));
#45765=CARTESIAN_POINT('Ctrl Pts',(-1.57087397835723,1.,-1.31558903860016));
#45766=CARTESIAN_POINT('Ctrl Pts',(-1.5768005650559,1.,-1.31731642317187));
#45767=CARTESIAN_POINT('Ctrl Pts',(-1.58274907898834,1.,-1.31900135021432));
#45768=CARTESIAN_POINT('Ctrl Pts',(-1.58872057258245,1.,-1.32064537110892));
#45769=CARTESIAN_POINT('Ctrl Pts',(-1.59471591079403,1.,-1.32224985747682));
#45770=CARTESIAN_POINT('Ctrl Pts',(-1.60073511858687,1.,-1.32381550858256));
#45771=CARTESIAN_POINT('Ctrl Pts',(-1.60677758290954,1.,-1.32534250785782));
#45772=CARTESIAN_POINT('Ctrl Pts',(-1.6128423401575,1.,-1.32683074483356));
#45773=CARTESIAN_POINT('Ctrl Pts',(-1.61892832270724,1.,-1.32828000610449));
#45774=CARTESIAN_POINT('Ctrl Pts',(-1.62503464209797,1.,-1.3296901950568));
#45775=CARTESIAN_POINT('Ctrl Pts',(-1.63116079730923,1.,-1.33106149345645));
#45776=CARTESIAN_POINT('Ctrl Pts',(-1.63730653475089,1.,-1.33239425103724));
#45777=CARTESIAN_POINT('Ctrl Pts',(-1.6434717485603,1.,-1.33368890676572));
#45778=CARTESIAN_POINT('Ctrl Pts',(-1.6496563728683,1.,-1.33494590467993));
#45779=CARTESIAN_POINT('Ctrl Pts',(-1.65586025952593,1.,-1.33616559745172));
#45780=CARTESIAN_POINT('Ctrl Pts',(-1.66208312541983,1.,-1.33734820885262));
#45781=CARTESIAN_POINT('Ctrl Pts',(-1.66832460783989,1.,-1.33849388654388));
#45782=CARTESIAN_POINT('Ctrl Pts',(-1.67458429426086,1.,-1.3396027347034));
#45783=CARTESIAN_POINT('Ctrl Pts',(-1.68086176030362,1.,-1.34067485185203));
#45784=CARTESIAN_POINT('Ctrl Pts',(-1.68715660868764,1.,-1.341710374848));
#45785=CARTESIAN_POINT('Ctrl Pts',(-1.6934684849687,1.,-1.34270948206319));
#45786=CARTESIAN_POINT('Ctrl Pts',(-1.69979707754427,1.,-1.34367237124483));
#45787=CARTESIAN_POINT('Ctrl Pts',(-1.70614212266738,1.,-1.34459924533831));
#45788=CARTESIAN_POINT('Ctrl Pts',(-1.71250340686822,1.,-1.34549029589416));
#45789=CARTESIAN_POINT('Ctrl Pts',(-1.7188807715049,1.,-1.34634568653227));
#45790=CARTESIAN_POINT('Ctrl Pts',(-1.72527410680674,1.,-1.34716554819527));
#45791=CARTESIAN_POINT('Ctrl Pts',(-1.7304014965394,1.,-1.34779309152035));
#45792=CARTESIAN_POINT('Ctrl Pts',(-1.73425417885907,1.,-1.34824783112887));
#45793=CARTESIAN_POINT('Ctrl Pts',(-1.73682580585691,1.,-1.34854391898045));
#45794=CARTESIAN_POINT('Ctrl Pts',(-1.73811241238545,1.,-1.34869019493419));
#45795=CARTESIAN_POINT('',(-1.31362392696032,0.,-1.15624053661742));
#45796=CARTESIAN_POINT('Origin',(0.,0.,0.));
#45797=CARTESIAN_POINT('',(-1.15624053661742,1.,-1.31362392696033));
#45798=CARTESIAN_POINT('Origin',(0.,1.,0.));
#45799=CARTESIAN_POINT('',(-1.15624053661742,0.,-1.31362392696033));
#45800=CARTESIAN_POINT('Ctrl Pts',(-1.34869019493419,-1.,-1.73811241238545));
#45801=CARTESIAN_POINT('Ctrl Pts',(-1.34869019493419,1.,-1.73811241238545));
#45802=CARTESIAN_POINT('Ctrl Pts',(-1.34854391898145,-1.,-1.73682580585819));
#45803=CARTESIAN_POINT('Ctrl Pts',(-1.34854391898145,1.,-1.73682580585819));
#45804=CARTESIAN_POINT('Ctrl Pts',(-1.34824783113158,-1.,-1.73425417886255));
#45805=CARTESIAN_POINT('Ctrl Pts',(-1.34824783113158,1.,-1.73425417886255));
#45806=CARTESIAN_POINT('Ctrl Pts',(-1.3477930915247,-1.,-1.73040149654497));
#45807=CARTESIAN_POINT('Ctrl Pts',(-1.3477930915247,1.,-1.73040149654497));
#45808=CARTESIAN_POINT('Ctrl Pts',(-1.34716554820013,-1.,-1.72527410681298));
#45809=CARTESIAN_POINT('Ctrl Pts',(-1.34716554820013,1.,-1.72527410681298));
#45810=CARTESIAN_POINT('Ctrl Pts',(-1.34634568653586,-1.,-1.7188807715095));
#45811=CARTESIAN_POINT('Ctrl Pts',(-1.34634568653586,1.,-1.7188807715095));
#45812=CARTESIAN_POINT('Ctrl Pts',(-1.34549029589563,-1.,-1.71250340687011));
#45813=CARTESIAN_POINT('Ctrl Pts',(-1.34549029589563,1.,-1.71250340687011));
#45814=CARTESIAN_POINT('Ctrl Pts',(-1.34459924533783,-1.,-1.70614212266676));
#45815=CARTESIAN_POINT('Ctrl Pts',(-1.34459924533783,1.,-1.70614212266676));
#45816=CARTESIAN_POINT('Ctrl Pts',(-1.34367237124322,-1.,-1.69979707754221));
#45817=CARTESIAN_POINT('Ctrl Pts',(-1.34367237124322,1.,-1.69979707754221));
#45818=CARTESIAN_POINT('Ctrl Pts',(-1.34270948206139,-1.,-1.6934684849664));
#45819=CARTESIAN_POINT('Ctrl Pts',(-1.34270948206139,1.,-1.6934684849664));
#45820=CARTESIAN_POINT('Ctrl Pts',(-1.34171037484673,-1.,-1.68715660868602));
#45821=CARTESIAN_POINT('Ctrl Pts',(-1.34171037484673,1.,-1.68715660868602));
#45822=CARTESIAN_POINT('Ctrl Pts',(-1.3406748518516,-1.,-1.68086176030308));
#45823=CARTESIAN_POINT('Ctrl Pts',(-1.3406748518516,1.,-1.68086176030308));
#45824=CARTESIAN_POINT('Ctrl Pts',(-1.33960273470372,-1.,-1.67458429426126));
#45825=CARTESIAN_POINT('Ctrl Pts',(-1.33960273470372,1.,-1.67458429426126));
#45826=CARTESIAN_POINT('Ctrl Pts',(-1.33849388654458,-1.,-1.66832460784078));
#45827=CARTESIAN_POINT('Ctrl Pts',(-1.33849388654458,1.,-1.66832460784078));
#45828=CARTESIAN_POINT('Ctrl Pts',(-1.33734820885331,-1.,-1.66208312542073));
#45829=CARTESIAN_POINT('Ctrl Pts',(-1.33734820885331,1.,-1.66208312542073));
#45830=CARTESIAN_POINT('Ctrl Pts',(-1.33616559745217,-1.,-1.65586025952651));
#45831=CARTESIAN_POINT('Ctrl Pts',(-1.33616559745217,1.,-1.65586025952651));
#45832=CARTESIAN_POINT('Ctrl Pts',(-1.33494590468003,-1.,-1.64965637286843));
#45833=CARTESIAN_POINT('Ctrl Pts',(-1.33494590468003,1.,-1.64965637286843));
#45834=CARTESIAN_POINT('Ctrl Pts',(-1.33368890676554,-1.,-1.64347174856007));
#45835=CARTESIAN_POINT('Ctrl Pts',(-1.33368890676554,1.,-1.64347174856007));
#45836=CARTESIAN_POINT('Ctrl Pts',(-1.33239425103694,-1.,-1.6373065347505));
#45837=CARTESIAN_POINT('Ctrl Pts',(-1.33239425103694,1.,-1.6373065347505));
#45838=CARTESIAN_POINT('Ctrl Pts',(-1.33106149345618,-1.,-1.63116079730887));
#45839=CARTESIAN_POINT('Ctrl Pts',(-1.33106149345618,1.,-1.63116079730887));
#45840=CARTESIAN_POINT('Ctrl Pts',(-1.32969019505665,-1.,-1.62503464209777));
#45841=CARTESIAN_POINT('Ctrl Pts',(-1.32969019505665,1.,-1.62503464209777));
#45842=CARTESIAN_POINT('Ctrl Pts',(-1.32828000610448,-1.,-1.61892832270723));
#45843=CARTESIAN_POINT('Ctrl Pts',(-1.32828000610448,1.,-1.61892832270723));
#45844=CARTESIAN_POINT('Ctrl Pts',(-1.32683074483365,-1.,-1.61284234015762));
#45845=CARTESIAN_POINT('Ctrl Pts',(-1.32683074483365,1.,-1.61284234015762));
#45846=CARTESIAN_POINT('Ctrl Pts',(-1.32534250785794,-1.,-1.6067775829097));
#45847=CARTESIAN_POINT('Ctrl Pts',(-1.32534250785794,1.,-1.6067775829097));
#45848=CARTESIAN_POINT('Ctrl Pts',(-1.32381550858266,-1.,-1.600735118587));
#45849=CARTESIAN_POINT('Ctrl Pts',(-1.32381550858266,1.,-1.600735118587));
#45850=CARTESIAN_POINT('Ctrl Pts',(-1.32224985747686,-1.,-1.59471591079408));
#45851=CARTESIAN_POINT('Ctrl Pts',(-1.32224985747686,1.,-1.59471591079408));
#45852=CARTESIAN_POINT('Ctrl Pts',(-1.32064537110891,-1.,-1.58872057258244));
#45853=CARTESIAN_POINT('Ctrl Pts',(-1.32064537110891,1.,-1.58872057258244));
#45854=CARTESIAN_POINT('Ctrl Pts',(-1.31900135021428,-1.,-1.58274907898829));
#45855=CARTESIAN_POINT('Ctrl Pts',(-1.31900135021428,1.,-1.58274907898829));
#45856=CARTESIAN_POINT('Ctrl Pts',(-1.31731642317183,-1.,-1.57680056505585));
#45857=CARTESIAN_POINT('Ctrl Pts',(-1.31731642317183,1.,-1.57680056505585));
#45858=CARTESIAN_POINT('Ctrl Pts',(-1.31558903860015,-1.,-1.57087397835721));
#45859=CARTESIAN_POINT('Ctrl Pts',(-1.31558903860015,1.,-1.57087397835721));
#45860=CARTESIAN_POINT('Ctrl Pts',(-1.31381795281002,-1.,-1.56496872402352));
#45861=CARTESIAN_POINT('Ctrl Pts',(-1.31381795281002,1.,-1.56496872402352));
#45862=CARTESIAN_POINT('Ctrl Pts',(-1.31200264341696,-1.,-1.55908521254822));
#45863=CARTESIAN_POINT('Ctrl Pts',(-1.31200264341696,1.,-1.55908521254822));
#45864=CARTESIAN_POINT('Ctrl Pts',(-1.31014393684221,-1.,-1.55322568759481));
#45865=CARTESIAN_POINT('Ctrl Pts',(-1.31014393684221,1.,-1.55322568759481));
#45866=CARTESIAN_POINT('Ctrl Pts',(-1.30824393907471,-1.,-1.54739413957183));
#45867=CARTESIAN_POINT('Ctrl Pts',(-1.30824393907471,1.,-1.54739413957183));
#45868=CARTESIAN_POINT('Ctrl Pts',(-1.30630475189553,-1.,-1.54159462645428));
#45869=CARTESIAN_POINT('Ctrl Pts',(-1.30630475189553,1.,-1.54159462645428));
#45870=CARTESIAN_POINT('Ctrl Pts',(-1.30432735639487,-1.,-1.53582981268976));
#45871=CARTESIAN_POINT('Ctrl Pts',(-1.30432735639487,1.,-1.53582981268976));
#45872=CARTESIAN_POINT('Ctrl Pts',(-1.3023106439557,-1.,-1.53009970283893));
#45873=CARTESIAN_POINT('Ctrl Pts',(-1.3023106439557,1.,-1.53009970283893));
#45874=CARTESIAN_POINT('Ctrl Pts',(-1.30024984366334,-1.,-1.5243995786107));
#45875=CARTESIAN_POINT('Ctrl Pts',(-1.30024984366334,1.,-1.5243995786107));
#45876=CARTESIAN_POINT('Ctrl Pts',(-1.29813791800757,-1.,-1.51872184912735));
#45877=CARTESIAN_POINT('Ctrl Pts',(-1.29813791800757,1.,-1.51872184912735));
#45878=CARTESIAN_POINT('Ctrl Pts',(-1.29596850710518,-1.,-1.51305994241412));
#45879=CARTESIAN_POINT('Ctrl Pts',(-1.29596850710518,1.,-1.51305994241412));
#45880=CARTESIAN_POINT('Ctrl Pts',(-1.29373841372843,-1.,-1.50741159078367));
#45881=CARTESIAN_POINT('Ctrl Pts',(-1.29373841372843,1.,-1.50741159078367));
#45882=CARTESIAN_POINT('Ctrl Pts',(-1.29145022885171,-1.,-1.50178230149764));
#45883=CARTESIAN_POINT('Ctrl Pts',(-1.29145022885171,1.,-1.50178230149764));
#45884=CARTESIAN_POINT('Ctrl Pts',(-1.28911506584232,-1.,-1.49618896881729));
#45885=CARTESIAN_POINT('Ctrl Pts',(-1.28911506584232,1.,-1.49618896881729));
#45886=CARTESIAN_POINT('Ctrl Pts',(-1.28674676116415,-1.,-1.4906522831275));
#45887=CARTESIAN_POINT('Ctrl Pts',(-1.28674676116415,1.,-1.4906522831275));
#45888=CARTESIAN_POINT('Ctrl Pts',(-1.28435533880184,-1.,-1.48518817118891));
#45889=CARTESIAN_POINT('Ctrl Pts',(-1.28435533880184,1.,-1.48518817118891));
#45890=CARTESIAN_POINT('Ctrl Pts',(-1.28194158939522,-1.,-1.47980070347102));
#45891=CARTESIAN_POINT('Ctrl Pts',(-1.28194158939522,1.,-1.47980070347102));
#45892=CARTESIAN_POINT('Ctrl Pts',(-1.27948918248524,-1.,-1.4744717526711));
#45893=CARTESIAN_POINT('Ctrl Pts',(-1.27948918248524,1.,-1.4744717526711));
#45894=CARTESIAN_POINT('Ctrl Pts',(-1.27696414831144,-1.,-1.46916035917197));
#45895=CARTESIAN_POINT('Ctrl Pts',(-1.27696414831144,1.,-1.46916035917197));
#45896=CARTESIAN_POINT('Ctrl Pts',(-1.27433119897877,-1.,-1.4638243133254));
#45897=CARTESIAN_POINT('Ctrl Pts',(-1.27433119897877,1.,-1.4638243133254));
#45898=CARTESIAN_POINT('Ctrl Pts',(-1.27156805265312,-1.,-1.45843906294725));
#45899=CARTESIAN_POINT('Ctrl Pts',(-1.27156805265312,1.,-1.45843906294725));
#45900=CARTESIAN_POINT('Ctrl Pts',(-1.26867786804854,-1.,-1.45301422764205));
#45901=CARTESIAN_POINT('Ctrl Pts',(-1.26867786804854,1.,-1.45301422764205));
#45902=CARTESIAN_POINT('Ctrl Pts',(-1.26570925118767,-1.,-1.44761985001544));
#45903=CARTESIAN_POINT('Ctrl Pts',(-1.26570925118767,1.,-1.44761985001544));
#45904=CARTESIAN_POINT('Ctrl Pts',(-1.26273903323723,-1.,-1.44236470511145));
#45905=CARTESIAN_POINT('Ctrl Pts',(-1.26273903323723,1.,-1.44236470511145));
#45906=CARTESIAN_POINT('Ctrl Pts',(-1.25983531011894,-1.,-1.43734919180719));
#45907=CARTESIAN_POINT('Ctrl Pts',(-1.25983531011894,1.,-1.43734919180719));
#45908=CARTESIAN_POINT('Ctrl Pts',(-1.25702687965744,-1.,-1.43262645609679));
#45909=CARTESIAN_POINT('Ctrl Pts',(-1.25702687965744,1.,-1.43262645609679));
#45910=CARTESIAN_POINT('Ctrl Pts',(-1.25426945222783,-1.,-1.42815938799555));
#45911=CARTESIAN_POINT('Ctrl Pts',(-1.25426945222783,1.,-1.42815938799555));
#45912=CARTESIAN_POINT('Ctrl Pts',(-1.25141455570299,-1.,-1.42378102115911));
#45913=CARTESIAN_POINT('Ctrl Pts',(-1.25141455570299,1.,-1.42378102115911));
#45914=CARTESIAN_POINT('Ctrl Pts',(-1.24824430986911,-1.,-1.41923722596421));
#45915=CARTESIAN_POINT('Ctrl Pts',(-1.24824430986911,1.,-1.41923722596421));
#45916=CARTESIAN_POINT('Ctrl Pts',(-1.24450600513278,-1.,-1.41422913175437));
#45917=CARTESIAN_POINT('Ctrl Pts',(-1.24450600513278,1.,-1.41422913175437));
#45918=CARTESIAN_POINT('Ctrl Pts',(-1.23994455029421,-1.,-1.40845295531151));
#45919=CARTESIAN_POINT('Ctrl Pts',(-1.23994455029421,1.,-1.40845295531151));
#45920=CARTESIAN_POINT('Ctrl Pts',(-1.23434087289768,-1.,-1.40164708205345));
#45921=CARTESIAN_POINT('Ctrl Pts',(-1.23434087289768,1.,-1.40164708205345));
#45922=CARTESIAN_POINT('Ctrl Pts',(-1.22752961898063,-1.,-1.39361389567257));
#45923=CARTESIAN_POINT('Ctrl Pts',(-1.22752961898063,1.,-1.39361389567257));
#45924=CARTESIAN_POINT('Ctrl Pts',(-1.21938737278853,-1.,-1.38420564525391));
#45925=CARTESIAN_POINT('Ctrl Pts',(-1.21938737278853,1.,-1.38420564525391));
#45926=CARTESIAN_POINT('Ctrl Pts',(-1.20982812923113,-1.,-1.37331915604962));
#45927=CARTESIAN_POINT('Ctrl Pts',(-1.20982812923113,1.,-1.37331915604962));
#45928=CARTESIAN_POINT('Ctrl Pts',(-1.1987959077656,-1.,-1.36088705040677));
#45929=CARTESIAN_POINT('Ctrl Pts',(-1.1987959077656,1.,-1.36088705040677));
#45930=CARTESIAN_POINT('Ctrl Pts',(-1.18625865664915,-1.,-1.34687053998157));
#45931=CARTESIAN_POINT('Ctrl Pts',(-1.18625865664915,1.,-1.34687053998157));
#45932=CARTESIAN_POINT('Ctrl Pts',(-1.17501305787994,-1.,-1.33437539344842));
#45933=CARTESIAN_POINT('Ctrl Pts',(-1.17501305787994,1.,-1.33437539344842));
#45934=CARTESIAN_POINT('Ctrl Pts',(-1.16589330092532,-1.,-1.32428080720544));
#45935=CARTESIAN_POINT('Ctrl Pts',(-1.16589330092532,1.,-1.32428080720544));
#45936=CARTESIAN_POINT('Ctrl Pts',(-1.15950888730433,-1.,-1.3172297721596));
#45937=CARTESIAN_POINT('Ctrl Pts',(-1.15950888730433,1.,-1.3172297721596));
#45938=CARTESIAN_POINT('Ctrl Pts',(-1.15624053661742,-1.,-1.31362392696033));
#45939=CARTESIAN_POINT('Ctrl Pts',(-1.15624053661742,1.,-1.31362392696033));
#45940=CARTESIAN_POINT('',(-1.34869019493419,1.,-1.73811241238545));
#45941=CARTESIAN_POINT('Ctrl Pts',(-1.34869019493419,1.,-1.73811241238545));
#45942=CARTESIAN_POINT('Ctrl Pts',(-1.34854391898145,1.,-1.73682580585819));
#45943=CARTESIAN_POINT('Ctrl Pts',(-1.34824783113158,1.,-1.73425417886255));
#45944=CARTESIAN_POINT('Ctrl Pts',(-1.3477930915247,1.,-1.73040149654497));
#45945=CARTESIAN_POINT('Ctrl Pts',(-1.34716554820013,1.,-1.72527410681298));
#45946=CARTESIAN_POINT('Ctrl Pts',(-1.34634568653586,1.,-1.7188807715095));
#45947=CARTESIAN_POINT('Ctrl Pts',(-1.34549029589563,1.,-1.71250340687011));
#45948=CARTESIAN_POINT('Ctrl Pts',(-1.34459924533783,1.,-1.70614212266676));
#45949=CARTESIAN_POINT('Ctrl Pts',(-1.34367237124322,1.,-1.69979707754221));
#45950=CARTESIAN_POINT('Ctrl Pts',(-1.34270948206139,1.,-1.6934684849664));
#45951=CARTESIAN_POINT('Ctrl Pts',(-1.34171037484673,1.,-1.68715660868602));
#45952=CARTESIAN_POINT('Ctrl Pts',(-1.3406748518516,1.,-1.68086176030308));
#45953=CARTESIAN_POINT('Ctrl Pts',(-1.33960273470372,1.,-1.67458429426126));
#45954=CARTESIAN_POINT('Ctrl Pts',(-1.33849388654458,1.,-1.66832460784078));
#45955=CARTESIAN_POINT('Ctrl Pts',(-1.33734820885331,1.,-1.66208312542073));
#45956=CARTESIAN_POINT('Ctrl Pts',(-1.33616559745217,1.,-1.65586025952651));
#45957=CARTESIAN_POINT('Ctrl Pts',(-1.33494590468003,1.,-1.64965637286843));
#45958=CARTESIAN_POINT('Ctrl Pts',(-1.33368890676554,1.,-1.64347174856007));
#45959=CARTESIAN_POINT('Ctrl Pts',(-1.33239425103694,1.,-1.6373065347505));
#45960=CARTESIAN_POINT('Ctrl Pts',(-1.33106149345618,1.,-1.63116079730887));
#45961=CARTESIAN_POINT('Ctrl Pts',(-1.32969019505665,1.,-1.62503464209777));
#45962=CARTESIAN_POINT('Ctrl Pts',(-1.32828000610448,1.,-1.61892832270723));
#45963=CARTESIAN_POINT('Ctrl Pts',(-1.32683074483365,1.,-1.61284234015762));
#45964=CARTESIAN_POINT('Ctrl Pts',(-1.32534250785794,1.,-1.6067775829097));
#45965=CARTESIAN_POINT('Ctrl Pts',(-1.32381550858266,1.,-1.600735118587));
#45966=CARTESIAN_POINT('Ctrl Pts',(-1.32224985747686,1.,-1.59471591079408));
#45967=CARTESIAN_POINT('Ctrl Pts',(-1.32064537110891,1.,-1.58872057258244));
#45968=CARTESIAN_POINT('Ctrl Pts',(-1.31900135021428,1.,-1.58274907898829));
#45969=CARTESIAN_POINT('Ctrl Pts',(-1.31731642317183,1.,-1.57680056505585));
#45970=CARTESIAN_POINT('Ctrl Pts',(-1.31558903860015,1.,-1.57087397835721));
#45971=CARTESIAN_POINT('Ctrl Pts',(-1.31381795281002,1.,-1.56496872402352));
#45972=CARTESIAN_POINT('Ctrl Pts',(-1.31200264341696,1.,-1.55908521254822));
#45973=CARTESIAN_POINT('Ctrl Pts',(-1.31014393684221,1.,-1.55322568759481));
#45974=CARTESIAN_POINT('Ctrl Pts',(-1.30824393907471,1.,-1.54739413957183));
#45975=CARTESIAN_POINT('Ctrl Pts',(-1.30630475189553,1.,-1.54159462645428));
#45976=CARTESIAN_POINT('Ctrl Pts',(-1.30432735639487,1.,-1.53582981268976));
#45977=CARTESIAN_POINT('Ctrl Pts',(-1.3023106439557,1.,-1.53009970283893));
#45978=CARTESIAN_POINT('Ctrl Pts',(-1.30024984366334,1.,-1.5243995786107));
#45979=CARTESIAN_POINT('Ctrl Pts',(-1.29813791800757,1.,-1.51872184912735));
#45980=CARTESIAN_POINT('Ctrl Pts',(-1.29596850710518,1.,-1.51305994241412));
#45981=CARTESIAN_POINT('Ctrl Pts',(-1.29373841372843,1.,-1.50741159078367));
#45982=CARTESIAN_POINT('Ctrl Pts',(-1.29145022885171,1.,-1.50178230149764));
#45983=CARTESIAN_POINT('Ctrl Pts',(-1.28911506584232,1.,-1.49618896881729));
#45984=CARTESIAN_POINT('Ctrl Pts',(-1.28674676116415,1.,-1.4906522831275));
#45985=CARTESIAN_POINT('Ctrl Pts',(-1.28435533880184,1.,-1.48518817118891));
#45986=CARTESIAN_POINT('Ctrl Pts',(-1.28194158939522,1.,-1.47980070347102));
#45987=CARTESIAN_POINT('Ctrl Pts',(-1.27948918248524,1.,-1.4744717526711));
#45988=CARTESIAN_POINT('Ctrl Pts',(-1.27696414831144,1.,-1.46916035917197));
#45989=CARTESIAN_POINT('Ctrl Pts',(-1.27433119897877,1.,-1.4638243133254));
#45990=CARTESIAN_POINT('Ctrl Pts',(-1.27156805265312,1.,-1.45843906294725));
#45991=CARTESIAN_POINT('Ctrl Pts',(-1.26867786804854,1.,-1.45301422764205));
#45992=CARTESIAN_POINT('Ctrl Pts',(-1.26570925118767,1.,-1.44761985001544));
#45993=CARTESIAN_POINT('Ctrl Pts',(-1.26273903323723,1.,-1.44236470511145));
#45994=CARTESIAN_POINT('Ctrl Pts',(-1.25983531011894,1.,-1.43734919180719));
#45995=CARTESIAN_POINT('Ctrl Pts',(-1.25702687965744,1.,-1.43262645609679));
#45996=CARTESIAN_POINT('Ctrl Pts',(-1.25426945222783,1.,-1.42815938799555));
#45997=CARTESIAN_POINT('Ctrl Pts',(-1.25141455570299,1.,-1.42378102115911));
#45998=CARTESIAN_POINT('Ctrl Pts',(-1.24824430986911,1.,-1.41923722596421));
#45999=CARTESIAN_POINT('Ctrl Pts',(-1.24450600513278,1.,-1.41422913175437));
#46000=CARTESIAN_POINT('Ctrl Pts',(-1.23994455029421,1.,-1.40845295531151));
#46001=CARTESIAN_POINT('Ctrl Pts',(-1.23434087289768,1.,-1.40164708205345));
#46002=CARTESIAN_POINT('Ctrl Pts',(-1.22752961898063,1.,-1.39361389567257));
#46003=CARTESIAN_POINT('Ctrl Pts',(-1.21938737278853,1.,-1.38420564525391));
#46004=CARTESIAN_POINT('Ctrl Pts',(-1.20982812923113,1.,-1.37331915604962));
#46005=CARTESIAN_POINT('Ctrl Pts',(-1.1987959077656,1.,-1.36088705040677));
#46006=CARTESIAN_POINT('Ctrl Pts',(-1.18625865664915,1.,-1.34687053998157));
#46007=CARTESIAN_POINT('Ctrl Pts',(-1.17501305787994,1.,-1.33437539344842));
#46008=CARTESIAN_POINT('Ctrl Pts',(-1.16589330092532,1.,-1.32428080720544));
#46009=CARTESIAN_POINT('Ctrl Pts',(-1.15950888730433,1.,-1.3172297721596));
#46010=CARTESIAN_POINT('Ctrl Pts',(-1.15624053661742,1.,-1.31362392696033));
#46011=CARTESIAN_POINT('',(-1.34869019493419,0.,-1.73811241238545));
#46012=CARTESIAN_POINT('Origin',(-1.23627494547115,0.,-1.81978687191668));
#46013=CARTESIAN_POINT('',(-1.23627494547115,1.,-1.81978687191668));
#46014=CARTESIAN_POINT('',(-1.34869019493419,1.,-1.73811241238545));
#46015=CARTESIAN_POINT('',(-1.23627494547115,0.,-1.81978687191668));
#46016=CARTESIAN_POINT('Ctrl Pts',(-0.892032620296855,-1.,-1.5055822144029));
#46017=CARTESIAN_POINT('Ctrl Pts',(-0.892032620296855,1.,-1.5055822144029));
#46018=CARTESIAN_POINT('Ctrl Pts',(-0.894452006967538,-1.,-1.50980486807181));
#46019=CARTESIAN_POINT('Ctrl Pts',(-0.894452006967538,1.,-1.50980486807181));
#46020=CARTESIAN_POINT('Ctrl Pts',(-0.89918504749193,-1.,-1.51805569591479));
#46021=CARTESIAN_POINT('Ctrl Pts',(-0.89918504749193,1.,-1.51805569591479));
#46022=CARTESIAN_POINT('Ctrl Pts',(-0.905967409640499,-1.,-1.52984849890434));
#46023=CARTESIAN_POINT('Ctrl Pts',(-0.905967409640499,1.,-1.52984849890434));
#46024=CARTESIAN_POINT('Ctrl Pts',(-0.91437591904658,-1.,-1.54440491152808));
#46025=CARTESIAN_POINT('Ctrl Pts',(-0.91437591904658,1.,-1.54440491152808));
#46026=CARTESIAN_POINT('Ctrl Pts',(-0.923832188966322,-1.,-1.56065988582509));
#46027=CARTESIAN_POINT('Ctrl Pts',(-0.923832188966322,1.,-1.56065988582509));
#46028=CARTESIAN_POINT('Ctrl Pts',(-0.932246680128849,-1.,-1.57499388385561));
#46029=CARTESIAN_POINT('Ctrl Pts',(-0.932246680128849,1.,-1.57499388385561));
#46030=CARTESIAN_POINT('Ctrl Pts',(-0.939646377909319,-1.,-1.58744937489796));
#46031=CARTESIAN_POINT('Ctrl Pts',(-0.939646377909319,1.,-1.58744937489796));
#46032=CARTESIAN_POINT('Ctrl Pts',(-0.946078063325796,-1.,-1.59810042045408));
#46033=CARTESIAN_POINT('Ctrl Pts',(-0.946078063325796,1.,-1.59810042045408));
#46034=CARTESIAN_POINT('Ctrl Pts',(-0.951613284361248,-1.,-1.60706069897794));
#46035=CARTESIAN_POINT('Ctrl Pts',(-0.951613284361248,1.,-1.60706069897794));
#46036=CARTESIAN_POINT('Ctrl Pts',(-0.956354422921573,-1.,-1.61449324337233));
#46037=CARTESIAN_POINT('Ctrl Pts',(-0.956354422921573,1.,-1.61449324337233));
#46038=CARTESIAN_POINT('Ctrl Pts',(-0.960438326099958,-1.,-1.62061638139929));
#46039=CARTESIAN_POINT('Ctrl Pts',(-0.960438326099958,1.,-1.62061638139929));
#46040=CARTESIAN_POINT('Ctrl Pts',(-0.964046107037821,-1.,-1.6257193066974));
#46041=CARTESIAN_POINT('Ctrl Pts',(-0.964046107037821,1.,-1.6257193066974));
#46042=CARTESIAN_POINT('Ctrl Pts',(-0.967387853228041,-1.,-1.63013849959083));
#46043=CARTESIAN_POINT('Ctrl Pts',(-0.967387853228041,1.,-1.63013849959083));
#46044=CARTESIAN_POINT('Ctrl Pts',(-0.970669715996356,-1.,-1.63420665729609));
#46045=CARTESIAN_POINT('Ctrl Pts',(-0.970669715996356,1.,-1.63420665729609));
#46046=CARTESIAN_POINT('Ctrl Pts',(-0.974066058287501,-1.,-1.63820952658157));
#46047=CARTESIAN_POINT('Ctrl Pts',(-0.974066058287501,1.,-1.63820952658157));
#46048=CARTESIAN_POINT('Ctrl Pts',(-0.977689794120297,-1.,-1.64233990826831));
#46049=CARTESIAN_POINT('Ctrl Pts',(-0.977689794120297,1.,-1.64233990826831));
#46050=CARTESIAN_POINT('Ctrl Pts',(-0.981562530940574,-1.,-1.64665139190834));
#46051=CARTESIAN_POINT('Ctrl Pts',(-0.981562530940574,1.,-1.64665139190834));
#46052=CARTESIAN_POINT('Ctrl Pts',(-0.985642622921626,-1.,-1.6511001661277));
#46053=CARTESIAN_POINT('Ctrl Pts',(-0.985642622921626,1.,-1.6511001661277));
#46054=CARTESIAN_POINT('Ctrl Pts',(-0.98985562785445,-1.,-1.65559044289746));
#46055=CARTESIAN_POINT('Ctrl Pts',(-0.98985562785445,1.,-1.65559044289746));
#46056=CARTESIAN_POINT('Ctrl Pts',(-0.994121836661116,-1.,-1.66001553809916));
#46057=CARTESIAN_POINT('Ctrl Pts',(-0.994121836661116,1.,-1.66001553809916));
#46058=CARTESIAN_POINT('Ctrl Pts',(-0.998389654952317,-1.,-1.66430758030304));
#46059=CARTESIAN_POINT('Ctrl Pts',(-0.998389654952317,1.,-1.66430758030304));
#46060=CARTESIAN_POINT('Ctrl Pts',(-1.00265091003682,-1.,-1.66846059277231));
#46061=CARTESIAN_POINT('Ctrl Pts',(-1.00265091003682,1.,-1.66846059277231));
#46062=CARTESIAN_POINT('Ctrl Pts',(-1.00692206696387,-1.,-1.67250335383248));
#46063=CARTESIAN_POINT('Ctrl Pts',(-1.00692206696387,1.,-1.67250335383248));
#46064=CARTESIAN_POINT('Ctrl Pts',(-1.01123236493507,-1.,-1.67648246776457));
#46065=CARTESIAN_POINT('Ctrl Pts',(-1.01123236493507,1.,-1.67648246776457));
#46066=CARTESIAN_POINT('Ctrl Pts',(-1.01561026162787,-1.,-1.6804428989482));
#46067=CARTESIAN_POINT('Ctrl Pts',(-1.01561026162787,1.,-1.6804428989482));
#46068=CARTESIAN_POINT('Ctrl Pts',(-1.02006795074222,-1.,-1.68440578021739));
#46069=CARTESIAN_POINT('Ctrl Pts',(-1.02006795074222,1.,-1.68440578021739));
#46070=CARTESIAN_POINT('Ctrl Pts',(-1.02460180535272,-1.,-1.68836910178475));
#46071=CARTESIAN_POINT('Ctrl Pts',(-1.02460180535272,1.,-1.68836910178475));
#46072=CARTESIAN_POINT('Ctrl Pts',(-1.02919977579155,-1.,-1.69231840863471));
#46073=CARTESIAN_POINT('Ctrl Pts',(-1.02919977579155,1.,-1.69231840863471));
#46074=CARTESIAN_POINT('Ctrl Pts',(-1.03384646003587,-1.,-1.69623414782769));
#46075=CARTESIAN_POINT('Ctrl Pts',(-1.03384646003587,1.,-1.69623414782769));
#46076=CARTESIAN_POINT('Ctrl Pts',(-1.03852922490782,-1.,-1.70010052930951));
#46077=CARTESIAN_POINT('Ctrl Pts',(-1.03852922490782,1.,-1.70010052930951));
#46078=CARTESIAN_POINT('Ctrl Pts',(-1.04324363334546,-1.,-1.70391338707969));
#46079=CARTESIAN_POINT('Ctrl Pts',(-1.04324363334546,1.,-1.70391338707969));
#46080=CARTESIAN_POINT('Ctrl Pts',(-1.0479908540499,-1.,-1.70767646263641));
#46081=CARTESIAN_POINT('Ctrl Pts',(-1.0479908540499,1.,-1.70767646263641));
#46082=CARTESIAN_POINT('Ctrl Pts',(-1.05277517202854,-1.,-1.71139783543986));
#46083=CARTESIAN_POINT('Ctrl Pts',(-1.05277517202854,1.,-1.71139783543986));
#46084=CARTESIAN_POINT('Ctrl Pts',(-1.05760163192481,-1.,-1.71508654427022));
#46085=CARTESIAN_POINT('Ctrl Pts',(-1.05760163192481,1.,-1.71508654427022));
#46086=CARTESIAN_POINT('Ctrl Pts',(-1.0624732468065,-1.,-1.71874858456908));
#46087=CARTESIAN_POINT('Ctrl Pts',(-1.0624732468065,1.,-1.71874858456908));
#46088=CARTESIAN_POINT('Ctrl Pts',(-1.06738966975463,-1.,-1.72238500928456));
#46089=CARTESIAN_POINT('Ctrl Pts',(-1.06738966975463,1.,-1.72238500928456));
#46090=CARTESIAN_POINT('Ctrl Pts',(-1.07234866990252,-1.,-1.72599406198489));
#46091=CARTESIAN_POINT('Ctrl Pts',(-1.07234866990252,1.,-1.72599406198489));
#46092=CARTESIAN_POINT('Ctrl Pts',(-1.0773470373727,-1.,-1.72957248977424));
#46093=CARTESIAN_POINT('Ctrl Pts',(-1.0773470373727,1.,-1.72957248977424));
#46094=CARTESIAN_POINT('Ctrl Pts',(-1.08238162784749,-1.,-1.73311705663407));
#46095=CARTESIAN_POINT('Ctrl Pts',(-1.08238162784749,1.,-1.73311705663407));
#46096=CARTESIAN_POINT('Ctrl Pts',(-1.08745056285429,-1.,-1.73662628326093));
#46097=CARTESIAN_POINT('Ctrl Pts',(-1.08745056285429,1.,-1.73662628326093));
#46098=CARTESIAN_POINT('Ctrl Pts',(-1.09255329056496,-1.,-1.74010053962252));
#46099=CARTESIAN_POINT('Ctrl Pts',(-1.09255329056496,1.,-1.74010053962252));
#46100=CARTESIAN_POINT('Ctrl Pts',(-1.09768999241229,-1.,-1.74354119236212));
#46101=CARTESIAN_POINT('Ctrl Pts',(-1.09768999241229,1.,-1.74354119236212));
#46102=CARTESIAN_POINT('Ctrl Pts',(-1.10286118991144,-1.,-1.74695004214924));
#46103=CARTESIAN_POINT('Ctrl Pts',(-1.10286118991144,1.,-1.74695004214924));
#46104=CARTESIAN_POINT('Ctrl Pts',(-1.10806728183003,-1.,-1.75032866075914));
#46105=CARTESIAN_POINT('Ctrl Pts',(-1.10806728183003,1.,-1.75032866075914));
#46106=CARTESIAN_POINT('Ctrl Pts',(-1.11330807582542,-1.,-1.75367772094617));
#46107=CARTESIAN_POINT('Ctrl Pts',(-1.11330807582542,1.,-1.75367772094617));
#46108=CARTESIAN_POINT('Ctrl Pts',(-1.11858293216752,-1.,-1.75699720772089));
#46109=CARTESIAN_POINT('Ctrl Pts',(-1.11858293216752,1.,-1.75699720772089));
#46110=CARTESIAN_POINT('Ctrl Pts',(-1.12389096855078,-1.,-1.76028671825084));
#46111=CARTESIAN_POINT('Ctrl Pts',(-1.12389096855078,1.,-1.76028671825084));
#46112=CARTESIAN_POINT('Ctrl Pts',(-1.12923123555076,-1.,-1.76354571966171));
#46113=CARTESIAN_POINT('Ctrl Pts',(-1.12923123555076,1.,-1.76354571966171));
#46114=CARTESIAN_POINT('Ctrl Pts',(-1.13460291804635,-1.,-1.76677384551883));
#46115=CARTESIAN_POINT('Ctrl Pts',(-1.13460291804635,1.,-1.76677384551883));
#46116=CARTESIAN_POINT('Ctrl Pts',(-1.14000548337,-1.,-1.76997111386806));
#46117=CARTESIAN_POINT('Ctrl Pts',(-1.14000548337,1.,-1.76997111386806));
#46118=CARTESIAN_POINT('Ctrl Pts',(-1.14543858226948,-1.,-1.77313777896234));
#46119=CARTESIAN_POINT('Ctrl Pts',(-1.14543858226948,1.,-1.77313777896234));
#46120=CARTESIAN_POINT('Ctrl Pts',(-1.15090197841531,-1.,-1.77627422557034));
#46121=CARTESIAN_POINT('Ctrl Pts',(-1.15090197841531,1.,-1.77627422557034));
#46122=CARTESIAN_POINT('Ctrl Pts',(-1.15639547194689,-1.,-1.77938085564261));
#46123=CARTESIAN_POINT('Ctrl Pts',(-1.15639547194689,1.,-1.77938085564261));
#46124=CARTESIAN_POINT('Ctrl Pts',(-1.16191881298458,-1.,-1.78245795880949));
#46125=CARTESIAN_POINT('Ctrl Pts',(-1.16191881298458,1.,-1.78245795880949));
#46126=CARTESIAN_POINT('Ctrl Pts',(-1.16747166312239,-1.,-1.78550566040349));
#46127=CARTESIAN_POINT('Ctrl Pts',(-1.16747166312239,1.,-1.78550566040349));
#46128=CARTESIAN_POINT('Ctrl Pts',(-1.17305363177265,-1.,-1.78852398877523));
#46129=CARTESIAN_POINT('Ctrl Pts',(-1.17305363177265,1.,-1.78852398877523));
#46130=CARTESIAN_POINT('Ctrl Pts',(-1.17866429440781,-1.,-1.79151291552646));
#46131=CARTESIAN_POINT('Ctrl Pts',(-1.17866429440781,1.,-1.79151291552646));
#46132=CARTESIAN_POINT('Ctrl Pts',(-1.18430321697471,-1.,-1.79447240321572));
#46133=CARTESIAN_POINT('Ctrl Pts',(-1.18430321697471,1.,-1.79447240321572));
#46134=CARTESIAN_POINT('Ctrl Pts',(-1.1899699793456,-1.,-1.79740245923649));
#46135=CARTESIAN_POINT('Ctrl Pts',(-1.1899699793456,1.,-1.79740245923649));
#46136=CARTESIAN_POINT('Ctrl Pts',(-1.19566418930405,-1.,-1.80030314370121));
#46137=CARTESIAN_POINT('Ctrl Pts',(-1.19566418930405,1.,-1.80030314370121));
#46138=CARTESIAN_POINT('Ctrl Pts',(-1.2013854893912,-1.,-1.8031745483882));
#46139=CARTESIAN_POINT('Ctrl Pts',(-1.2013854893912,1.,-1.8031745483882));
#46140=CARTESIAN_POINT('Ctrl Pts',(-1.20713356605519,-1.,-1.80601678480772));
#46141=CARTESIAN_POINT('Ctrl Pts',(-1.20713356605519,1.,-1.80601678480772));
#46142=CARTESIAN_POINT('Ctrl Pts',(-1.2129081570818,-1.,-1.80882996916931));
#46143=CARTESIAN_POINT('Ctrl Pts',(-1.2129081570818,1.,-1.80882996916931));
#46144=CARTESIAN_POINT('Ctrl Pts',(-1.2187090610323,-1.,-1.81161420806172));
#46145=CARTESIAN_POINT('Ctrl Pts',(-1.2187090610323,1.,-1.81161420806172));
#46146=CARTESIAN_POINT('Ctrl Pts',(-1.22453613304507,-1.,-1.81436959209778));
#46147=CARTESIAN_POINT('Ctrl Pts',(-1.22453613304507,1.,-1.81436959209778));
#46148=CARTESIAN_POINT('Ctrl Pts',(-1.22921864890975,-1.,-1.81655087183054));
#46149=CARTESIAN_POINT('Ctrl Pts',(-1.22921864890975,1.,-1.81655087183054));
#46150=CARTESIAN_POINT('Ctrl Pts',(-1.23274224526804,-1.,-1.81817389920914));
#46151=CARTESIAN_POINT('Ctrl Pts',(-1.23274224526804,1.,-1.81817389920914));
#46152=CARTESIAN_POINT('Ctrl Pts',(-1.23509651170384,-1.,-1.81925017193531));
#46153=CARTESIAN_POINT('Ctrl Pts',(-1.23509651170384,1.,-1.81925017193531));
#46154=CARTESIAN_POINT('Ctrl Pts',(-1.23627494547115,-1.,-1.81978687191668));
#46155=CARTESIAN_POINT('Ctrl Pts',(-1.23627494547115,1.,-1.81978687191668));
#46156=CARTESIAN_POINT('',(-0.892032620296855,1.,-1.5055822144029));
#46157=CARTESIAN_POINT('Ctrl Pts',(-0.892032620296855,1.,-1.5055822144029));
#46158=CARTESIAN_POINT('Ctrl Pts',(-0.894452006967538,1.,-1.50980486807181));
#46159=CARTESIAN_POINT('Ctrl Pts',(-0.89918504749193,1.,-1.51805569591479));
#46160=CARTESIAN_POINT('Ctrl Pts',(-0.905967409640499,1.,-1.52984849890434));
#46161=CARTESIAN_POINT('Ctrl Pts',(-0.91437591904658,1.,-1.54440491152808));
#46162=CARTESIAN_POINT('Ctrl Pts',(-0.923832188966322,1.,-1.56065988582509));
#46163=CARTESIAN_POINT('Ctrl Pts',(-0.932246680128849,1.,-1.57499388385561));
#46164=CARTESIAN_POINT('Ctrl Pts',(-0.939646377909319,1.,-1.58744937489796));
#46165=CARTESIAN_POINT('Ctrl Pts',(-0.946078063325796,1.,-1.59810042045408));
#46166=CARTESIAN_POINT('Ctrl Pts',(-0.951613284361248,1.,-1.60706069897794));
#46167=CARTESIAN_POINT('Ctrl Pts',(-0.956354422921573,1.,-1.61449324337233));
#46168=CARTESIAN_POINT('Ctrl Pts',(-0.960438326099958,1.,-1.62061638139929));
#46169=CARTESIAN_POINT('Ctrl Pts',(-0.964046107037821,1.,-1.6257193066974));
#46170=CARTESIAN_POINT('Ctrl Pts',(-0.967387853228041,1.,-1.63013849959083));
#46171=CARTESIAN_POINT('Ctrl Pts',(-0.970669715996356,1.,-1.63420665729609));
#46172=CARTESIAN_POINT('Ctrl Pts',(-0.974066058287501,1.,-1.63820952658157));
#46173=CARTESIAN_POINT('Ctrl Pts',(-0.977689794120297,1.,-1.64233990826831));
#46174=CARTESIAN_POINT('Ctrl Pts',(-0.981562530940574,1.,-1.64665139190834));
#46175=CARTESIAN_POINT('Ctrl Pts',(-0.985642622921626,1.,-1.6511001661277));
#46176=CARTESIAN_POINT('Ctrl Pts',(-0.98985562785445,1.,-1.65559044289746));
#46177=CARTESIAN_POINT('Ctrl Pts',(-0.994121836661116,1.,-1.66001553809916));
#46178=CARTESIAN_POINT('Ctrl Pts',(-0.998389654952317,1.,-1.66430758030304));
#46179=CARTESIAN_POINT('Ctrl Pts',(-1.00265091003682,1.,-1.66846059277231));
#46180=CARTESIAN_POINT('Ctrl Pts',(-1.00692206696387,1.,-1.67250335383248));
#46181=CARTESIAN_POINT('Ctrl Pts',(-1.01123236493507,1.,-1.67648246776457));
#46182=CARTESIAN_POINT('Ctrl Pts',(-1.01561026162787,1.,-1.6804428989482));
#46183=CARTESIAN_POINT('Ctrl Pts',(-1.02006795074222,1.,-1.68440578021739));
#46184=CARTESIAN_POINT('Ctrl Pts',(-1.02460180535272,1.,-1.68836910178475));
#46185=CARTESIAN_POINT('Ctrl Pts',(-1.02919977579155,1.,-1.69231840863471));
#46186=CARTESIAN_POINT('Ctrl Pts',(-1.03384646003587,1.,-1.69623414782769));
#46187=CARTESIAN_POINT('Ctrl Pts',(-1.03852922490782,1.,-1.70010052930951));
#46188=CARTESIAN_POINT('Ctrl Pts',(-1.04324363334546,1.,-1.70391338707969));
#46189=CARTESIAN_POINT('Ctrl Pts',(-1.0479908540499,1.,-1.70767646263641));
#46190=CARTESIAN_POINT('Ctrl Pts',(-1.05277517202854,1.,-1.71139783543986));
#46191=CARTESIAN_POINT('Ctrl Pts',(-1.05760163192481,1.,-1.71508654427022));
#46192=CARTESIAN_POINT('Ctrl Pts',(-1.0624732468065,1.,-1.71874858456908));
#46193=CARTESIAN_POINT('Ctrl Pts',(-1.06738966975463,1.,-1.72238500928456));
#46194=CARTESIAN_POINT('Ctrl Pts',(-1.07234866990252,1.,-1.72599406198489));
#46195=CARTESIAN_POINT('Ctrl Pts',(-1.0773470373727,1.,-1.72957248977424));
#46196=CARTESIAN_POINT('Ctrl Pts',(-1.08238162784749,1.,-1.73311705663407));
#46197=CARTESIAN_POINT('Ctrl Pts',(-1.08745056285429,1.,-1.73662628326093));
#46198=CARTESIAN_POINT('Ctrl Pts',(-1.09255329056496,1.,-1.74010053962252));
#46199=CARTESIAN_POINT('Ctrl Pts',(-1.09768999241229,1.,-1.74354119236212));
#46200=CARTESIAN_POINT('Ctrl Pts',(-1.10286118991144,1.,-1.74695004214924));
#46201=CARTESIAN_POINT('Ctrl Pts',(-1.10806728183003,1.,-1.75032866075914));
#46202=CARTESIAN_POINT('Ctrl Pts',(-1.11330807582542,1.,-1.75367772094617));
#46203=CARTESIAN_POINT('Ctrl Pts',(-1.11858293216752,1.,-1.75699720772089));
#46204=CARTESIAN_POINT('Ctrl Pts',(-1.12389096855078,1.,-1.76028671825084));
#46205=CARTESIAN_POINT('Ctrl Pts',(-1.12923123555076,1.,-1.76354571966171));
#46206=CARTESIAN_POINT('Ctrl Pts',(-1.13460291804635,1.,-1.76677384551883));
#46207=CARTESIAN_POINT('Ctrl Pts',(-1.14000548337,1.,-1.76997111386806));
#46208=CARTESIAN_POINT('Ctrl Pts',(-1.14543858226948,1.,-1.77313777896234));
#46209=CARTESIAN_POINT('Ctrl Pts',(-1.15090197841531,1.,-1.77627422557034));
#46210=CARTESIAN_POINT('Ctrl Pts',(-1.15639547194689,1.,-1.77938085564261));
#46211=CARTESIAN_POINT('Ctrl Pts',(-1.16191881298458,1.,-1.78245795880949));
#46212=CARTESIAN_POINT('Ctrl Pts',(-1.16747166312239,1.,-1.78550566040349));
#46213=CARTESIAN_POINT('Ctrl Pts',(-1.17305363177265,1.,-1.78852398877523));
#46214=CARTESIAN_POINT('Ctrl Pts',(-1.17866429440781,1.,-1.79151291552646));
#46215=CARTESIAN_POINT('Ctrl Pts',(-1.18430321697471,1.,-1.79447240321572));
#46216=CARTESIAN_POINT('Ctrl Pts',(-1.1899699793456,1.,-1.79740245923649));
#46217=CARTESIAN_POINT('Ctrl Pts',(-1.19566418930405,1.,-1.80030314370121));
#46218=CARTESIAN_POINT('Ctrl Pts',(-1.2013854893912,1.,-1.8031745483882));
#46219=CARTESIAN_POINT('Ctrl Pts',(-1.20713356605519,1.,-1.80601678480772));
#46220=CARTESIAN_POINT('Ctrl Pts',(-1.2129081570818,1.,-1.80882996916931));
#46221=CARTESIAN_POINT('Ctrl Pts',(-1.2187090610323,1.,-1.81161420806172));
#46222=CARTESIAN_POINT('Ctrl Pts',(-1.22453613304507,1.,-1.81436959209778));
#46223=CARTESIAN_POINT('Ctrl Pts',(-1.22921864890975,1.,-1.81655087183054));
#46224=CARTESIAN_POINT('Ctrl Pts',(-1.23274224526804,1.,-1.81817389920914));
#46225=CARTESIAN_POINT('Ctrl Pts',(-1.23509651170384,1.,-1.81925017193531));
#46226=CARTESIAN_POINT('Ctrl Pts',(-1.23627494547115,1.,-1.81978687191668));
#46227=CARTESIAN_POINT('',(-0.892032620296856,0.,-1.5055822144029));
#46228=CARTESIAN_POINT('Origin',(0.,0.,0.));
#46229=CARTESIAN_POINT('',(-0.693717979106305,1.,-1.60662857109684));
#46230=CARTESIAN_POINT('Origin',(0.,1.,0.));
#46231=CARTESIAN_POINT('',(-0.693717979106306,0.,-1.60662857109684));
#46232=CARTESIAN_POINT('Ctrl Pts',(-0.745574324794401,-1.,-2.0698113262342));
#46233=CARTESIAN_POINT('Ctrl Pts',(-0.745574324794401,1.,-2.0698113262342));
#46234=CARTESIAN_POINT('Ctrl Pts',(-0.745832791378367,-1.,-2.06854248895728));
#46235=CARTESIAN_POINT('Ctrl Pts',(-0.745832791378367,1.,-2.06854248895728));
#46236=CARTESIAN_POINT('Ctrl Pts',(-0.7463458715442,-1.,-2.06600523016815));
#46237=CARTESIAN_POINT('Ctrl Pts',(-0.7463458715442,1.,-2.06600523016815));
#46238=CARTESIAN_POINT('Ctrl Pts',(-0.747103932787919,-1.,-2.06220058927826));
#46239=CARTESIAN_POINT('Ctrl Pts',(-0.747103932787919,1.,-2.06220058927826));
#46240=CARTESIAN_POINT('Ctrl Pts',(-0.748091554183802,-1.,-2.05713023031006));
#46241=CARTESIAN_POINT('Ctrl Pts',(-0.748091554183802,1.,-2.05713023031006));
#46242=CARTESIAN_POINT('Ctrl Pts',(-0.749287468665046,-1.,-2.05079645592154));
#46243=CARTESIAN_POINT('Ctrl Pts',(-0.749287468665046,1.,-2.05079645592154));
#46244=CARTESIAN_POINT('Ctrl Pts',(-0.750444657875576,-1.,-2.04446689147979));
#46245=CARTESIAN_POINT('Ctrl Pts',(-0.750444657875576,1.,-2.04446689147979));
#46246=CARTESIAN_POINT('Ctrl Pts',(-0.751562963361115,-1.,-2.03814160092099));
#46247=CARTESIAN_POINT('Ctrl Pts',(-0.751562963361115,1.,-2.03814160092099));
#46248=CARTESIAN_POINT('Ctrl Pts',(-0.752642180487211,-1.,-2.03182068456221));
#46249=CARTESIAN_POINT('Ctrl Pts',(-0.752642180487211,1.,-2.03182068456221));
#46250=CARTESIAN_POINT('Ctrl Pts',(-0.753682061112768,-1.,-2.02550428623313));
#46251=CARTESIAN_POINT('Ctrl Pts',(-0.753682061112768,1.,-2.02550428623313));
#46252=CARTESIAN_POINT('Ctrl Pts',(-0.754682330722816,-1.,-2.01919259405809));
#46253=CARTESIAN_POINT('Ctrl Pts',(-0.754682330722816,1.,-2.01919259405809));
#46254=CARTESIAN_POINT('Ctrl Pts',(-0.755642704957865,-1.,-2.01288584328084));
#46255=CARTESIAN_POINT('Ctrl Pts',(-0.755642704957865,1.,-2.01288584328084));
#46256=CARTESIAN_POINT('Ctrl Pts',(-0.75656290464667,-1.,-2.0065843158773));
#46257=CARTESIAN_POINT('Ctrl Pts',(-0.75656290464667,1.,-2.0065843158773));
#46258=CARTESIAN_POINT('Ctrl Pts',(-0.757442676862724,-1.,-2.00028834739178));
#46259=CARTESIAN_POINT('Ctrl Pts',(-0.757442676862724,1.,-2.00028834739178));
#46260=CARTESIAN_POINT('Ctrl Pts',(-0.758281796766761,-1.,-1.99399831098817));
#46261=CARTESIAN_POINT('Ctrl Pts',(-0.758281796766761,1.,-1.99399831098817));
#46262=CARTESIAN_POINT('Ctrl Pts',(-0.759080037802488,-1.,-1.98771456680874));
#46263=CARTESIAN_POINT('Ctrl Pts',(-0.759080037802488,1.,-1.98771456680874));
#46264=CARTESIAN_POINT('Ctrl Pts',(-0.75983714745219,-1.,-1.98143741418172));
#46265=CARTESIAN_POINT('Ctrl Pts',(-0.75983714745219,1.,-1.98143741418172));
#46266=CARTESIAN_POINT('Ctrl Pts',(-0.760552825409757,-1.,-1.97516705321494));
#46267=CARTESIAN_POINT('Ctrl Pts',(-0.760552825409757,1.,-1.97516705321494));
#46268=CARTESIAN_POINT('Ctrl Pts',(-0.76122669048382,-1.,-1.96890351582499));
#46269=CARTESIAN_POINT('Ctrl Pts',(-0.76122669048382,1.,-1.96890351582499));
#46270=CARTESIAN_POINT('Ctrl Pts',(-0.761858300014423,-1.,-1.96264672744186));
#46271=CARTESIAN_POINT('Ctrl Pts',(-0.761858300014423,1.,-1.96264672744186));
#46272=CARTESIAN_POINT('Ctrl Pts',(-0.762447203806179,-1.,-1.95639665309869));
#46273=CARTESIAN_POINT('Ctrl Pts',(-0.762447203806179,1.,-1.95639665309869));
#46274=CARTESIAN_POINT('Ctrl Pts',(-0.762992990878769,-1.,-1.95015342590024));
#46275=CARTESIAN_POINT('Ctrl Pts',(-0.762992990878769,1.,-1.95015342590024));
#46276=CARTESIAN_POINT('Ctrl Pts',(-0.763495333538629,-1.,-1.9439174661764));
#46277=CARTESIAN_POINT('Ctrl Pts',(-0.763495333538629,1.,-1.9439174661764));
#46278=CARTESIAN_POINT('Ctrl Pts',(-0.763954049121458,-1.,-1.93768964875886));
#46279=CARTESIAN_POINT('Ctrl Pts',(-0.763954049121458,1.,-1.93768964875886));
#46280=CARTESIAN_POINT('Ctrl Pts',(-0.764369010673941,-1.,-1.93147105496382));
#46281=CARTESIAN_POINT('Ctrl Pts',(-0.764369010673941,1.,-1.93147105496382));
#46282=CARTESIAN_POINT('Ctrl Pts',(-0.764740025488211,-1.,-1.92526263537048));
#46283=CARTESIAN_POINT('Ctrl Pts',(-0.764740025488211,1.,-1.92526263537048));
#46284=CARTESIAN_POINT('Ctrl Pts',(-0.765066729667088,-1.,-1.91906491634196));
#46285=CARTESIAN_POINT('Ctrl Pts',(-0.765066729667088,1.,-1.91906491634196));
#46286=CARTESIAN_POINT('Ctrl Pts',(-0.765348465884722,-1.,-1.91287765805169));
#46287=CARTESIAN_POINT('Ctrl Pts',(-0.765348465884722,1.,-1.91287765805169));
#46288=CARTESIAN_POINT('Ctrl Pts',(-0.765584196937919,-1.,-1.90669961402356));
#46289=CARTESIAN_POINT('Ctrl Pts',(-0.765584196937919,1.,-1.90669961402356));
#46290=CARTESIAN_POINT('Ctrl Pts',(-0.765772772593386,-1.,-1.90052930393596));
#46291=CARTESIAN_POINT('Ctrl Pts',(-0.765772772593386,1.,-1.90052930393596));
#46292=CARTESIAN_POINT('Ctrl Pts',(-0.765913193856978,-1.,-1.89436577771388));
#46293=CARTESIAN_POINT('Ctrl Pts',(-0.765913193856978,1.,-1.89436577771388));
#46294=CARTESIAN_POINT('Ctrl Pts',(-0.766004837062091,-1.,-1.88820926433409));
#46295=CARTESIAN_POINT('Ctrl Pts',(-0.766004837062091,1.,-1.88820926433409));
#46296=CARTESIAN_POINT('Ctrl Pts',(-0.766047794851865,-1.,-1.88206215302561));
#46297=CARTESIAN_POINT('Ctrl Pts',(-0.766047794851865,1.,-1.88206215302561));
#46298=CARTESIAN_POINT('Ctrl Pts',(-0.766042837036744,-1.,-1.87592888967883));
#46299=CARTESIAN_POINT('Ctrl Pts',(-0.766042837036744,1.,-1.87592888967883));
#46300=CARTESIAN_POINT('Ctrl Pts',(-0.765990708546091,-1.,-1.86981398314341));
#46301=CARTESIAN_POINT('Ctrl Pts',(-0.765990708546091,1.,-1.86981398314341));
#46302=CARTESIAN_POINT('Ctrl Pts',(-0.765891519092547,-1.,-1.86372027063312));
#46303=CARTESIAN_POINT('Ctrl Pts',(-0.765891519092547,1.,-1.86372027063312));
#46304=CARTESIAN_POINT('Ctrl Pts',(-0.765744212909318,-1.,-1.85764741390394));
#46305=CARTESIAN_POINT('Ctrl Pts',(-0.765744212909318,1.,-1.85764741390394));
#46306=CARTESIAN_POINT('Ctrl Pts',(-0.765545710619062,-1.,-1.85158945130063));
#46307=CARTESIAN_POINT('Ctrl Pts',(-0.765545710619062,1.,-1.85158945130063));
#46308=CARTESIAN_POINT('Ctrl Pts',(-0.765291664862029,-1.,-1.84553698875924));
#46309=CARTESIAN_POINT('Ctrl Pts',(-0.765291664862029,1.,-1.84553698875924));
#46310=CARTESIAN_POINT('Ctrl Pts',(-0.764978057881737,-1.,-1.83948181064835));
#46311=CARTESIAN_POINT('Ctrl Pts',(-0.764978057881737,1.,-1.83948181064835));
#46312=CARTESIAN_POINT('Ctrl Pts',(-0.764602549687853,-1.,-1.83342077227142));
#46313=CARTESIAN_POINT('Ctrl Pts',(-0.764602549687853,1.,-1.83342077227142));
#46314=CARTESIAN_POINT('Ctrl Pts',(-0.764165902605995,-1.,-1.82735991200065));
#46315=CARTESIAN_POINT('Ctrl Pts',(-0.764165902605995,1.,-1.82735991200065));
#46316=CARTESIAN_POINT('Ctrl Pts',(-0.763673465462726,-1.,-1.82131873145266));
#46317=CARTESIAN_POINT('Ctrl Pts',(-0.763673465462726,1.,-1.82131873145266));
#46318=CARTESIAN_POINT('Ctrl Pts',(-0.763132003836634,-1.,-1.8153211840553));
#46319=CARTESIAN_POINT('Ctrl Pts',(-0.763132003836634,1.,-1.8153211840553));
#46320=CARTESIAN_POINT('Ctrl Pts',(-0.762546129463938,-1.,-1.80938551463965));
#46321=CARTESIAN_POINT('Ctrl Pts',(-0.762546129463938,1.,-1.80938551463965));
#46322=CARTESIAN_POINT('Ctrl Pts',(-0.761915336443547,-1.,-1.80351583877342));
#46323=CARTESIAN_POINT('Ctrl Pts',(-0.761915336443547,1.,-1.80351583877342));
#46324=CARTESIAN_POINT('Ctrl Pts',(-0.761229695230558,-1.,-1.79768986997783));
#46325=CARTESIAN_POINT('Ctrl Pts',(-0.761229695230558,1.,-1.79768986997783));
#46326=CARTESIAN_POINT('Ctrl Pts',(-0.760469555880749,-1.,-1.7918581561088));
#46327=CARTESIAN_POINT('Ctrl Pts',(-0.760469555880749,1.,-1.7918581561088));
#46328=CARTESIAN_POINT('Ctrl Pts',(-0.759614401110189,-1.,-1.78596964884604));
#46329=CARTESIAN_POINT('Ctrl Pts',(-0.759614401110189,1.,-1.78596964884604));
#46330=CARTESIAN_POINT('Ctrl Pts',(-0.758650626677518,-1.,-1.77999411220945));
#46331=CARTESIAN_POINT('Ctrl Pts',(-0.758650626677518,1.,-1.77999411220945));
#46332=CARTESIAN_POINT('Ctrl Pts',(-0.757578264077029,-1.,-1.77394167108292));
#46333=CARTESIAN_POINT('Ctrl Pts',(-0.757578264077029,1.,-1.77394167108292));
#46334=CARTESIAN_POINT('Ctrl Pts',(-0.75642189602781,-1.,-1.76789396002998));
#46335=CARTESIAN_POINT('Ctrl Pts',(-0.75642189602781,1.,-1.76789396002998));
#46336=CARTESIAN_POINT('Ctrl Pts',(-0.755220979974461,-1.,-1.76197817240128));
#46337=CARTESIAN_POINT('Ctrl Pts',(-0.755220979974461,1.,-1.76197817240128));
#46338=CARTESIAN_POINT('Ctrl Pts',(-0.754009254027829,-1.,-1.75631083600019));
#46339=CARTESIAN_POINT('Ctrl Pts',(-0.754009254027829,1.,-1.75631083600019));
#46340=CARTESIAN_POINT('Ctrl Pts',(-0.752797683531314,-1.,-1.75095139468794));
#46341=CARTESIAN_POINT('Ctrl Pts',(-0.752797683531314,1.,-1.75095139468794));
#46342=CARTESIAN_POINT('Ctrl Pts',(-0.751555614164482,-1.,-1.74585086852502));
#46343=CARTESIAN_POINT('Ctrl Pts',(-0.751555614164482,1.,-1.74585086852502));
#46344=CARTESIAN_POINT('Ctrl Pts',(-0.750193435981249,-1.,-1.74080458267114));
#46345=CARTESIAN_POINT('Ctrl Pts',(-0.750193435981249,1.,-1.74080458267114));
#46346=CARTESIAN_POINT('Ctrl Pts',(-0.74858246295687,-1.,-1.7355035168033));
#46347=CARTESIAN_POINT('Ctrl Pts',(-0.74858246295687,1.,-1.7355035168033));
#46348=CARTESIAN_POINT('Ctrl Pts',(-0.746574710097752,-1.,-1.72958533647714));
#46349=CARTESIAN_POINT('Ctrl Pts',(-0.746574710097752,1.,-1.72958533647714));
#46350=CARTESIAN_POINT('Ctrl Pts',(-0.744021445433093,-1.,-1.72268229916769));
#46351=CARTESIAN_POINT('Ctrl Pts',(-0.744021445433093,1.,-1.72268229916769));
#46352=CARTESIAN_POINT('Ctrl Pts',(-0.74079516202821,-1.,-1.71447789751001));
#46353=CARTESIAN_POINT('Ctrl Pts',(-0.74079516202821,1.,-1.71447789751001));
#46354=CARTESIAN_POINT('Ctrl Pts',(-0.736799665716932,-1.,-1.70473309004249));
#46355=CARTESIAN_POINT('Ctrl Pts',(-0.736799665716932,1.,-1.70473309004249));
#46356=CARTESIAN_POINT('Ctrl Pts',(-0.731963238685357,-1.,-1.69326921972915));
#46357=CARTESIAN_POINT('Ctrl Pts',(-0.731963238685357,1.,-1.69326921972915));
#46358=CARTESIAN_POINT('Ctrl Pts',(-0.726235967982445,-1.,-1.67996158451922));
#46359=CARTESIAN_POINT('Ctrl Pts',(-0.726235967982445,1.,-1.67996158451922));
#46360=CARTESIAN_POINT('Ctrl Pts',(-0.71958543378795,-1.,-1.66472880551777));
#46361=CARTESIAN_POINT('Ctrl Pts',(-0.71958543378795,1.,-1.66472880551777));
#46362=CARTESIAN_POINT('Ctrl Pts',(-0.711993139340447,-1.,-1.64752408828442));
#46363=CARTESIAN_POINT('Ctrl Pts',(-0.711993139340447,1.,-1.64752408828442));
#46364=CARTESIAN_POINT('Ctrl Pts',(-0.705159151977294,-1.,-1.6321654166204));
#46365=CARTESIAN_POINT('Ctrl Pts',(-0.705159151977294,1.,-1.6321654166204));
#46366=CARTESIAN_POINT('Ctrl Pts',(-0.699605146398837,-1.,-1.61974673471117));
#46367=CARTESIAN_POINT('Ctrl Pts',(-0.699605146398837,1.,-1.61974673471117));
#46368=CARTESIAN_POINT('Ctrl Pts',(-0.69571209787897,-1.,-1.61106790957619));
#46369=CARTESIAN_POINT('Ctrl Pts',(-0.69571209787897,1.,-1.61106790957619));
#46370=CARTESIAN_POINT('Ctrl Pts',(-0.693717979106305,-1.,-1.60662857109684));
#46371=CARTESIAN_POINT('Ctrl Pts',(-0.693717979106305,1.,-1.60662857109684));
#46372=CARTESIAN_POINT('',(-0.745574324794401,1.,-2.0698113262342));
#46373=CARTESIAN_POINT('Ctrl Pts',(-0.745574324794401,1.,-2.0698113262342));
#46374=CARTESIAN_POINT('Ctrl Pts',(-0.745832791378367,1.,-2.06854248895728));
#46375=CARTESIAN_POINT('Ctrl Pts',(-0.7463458715442,1.,-2.06600523016815));
#46376=CARTESIAN_POINT('Ctrl Pts',(-0.747103932787919,1.,-2.06220058927826));
#46377=CARTESIAN_POINT('Ctrl Pts',(-0.748091554183802,1.,-2.05713023031006));
#46378=CARTESIAN_POINT('Ctrl Pts',(-0.749287468665046,1.,-2.05079645592154));
#46379=CARTESIAN_POINT('Ctrl Pts',(-0.750444657875576,1.,-2.04446689147979));
#46380=CARTESIAN_POINT('Ctrl Pts',(-0.751562963361115,1.,-2.03814160092099));
#46381=CARTESIAN_POINT('Ctrl Pts',(-0.752642180487211,1.,-2.03182068456221));
#46382=CARTESIAN_POINT('Ctrl Pts',(-0.753682061112768,1.,-2.02550428623313));
#46383=CARTESIAN_POINT('Ctrl Pts',(-0.754682330722816,1.,-2.01919259405809));
#46384=CARTESIAN_POINT('Ctrl Pts',(-0.755642704957865,1.,-2.01288584328084));
#46385=CARTESIAN_POINT('Ctrl Pts',(-0.75656290464667,1.,-2.0065843158773));
#46386=CARTESIAN_POINT('Ctrl Pts',(-0.757442676862724,1.,-2.00028834739178));
#46387=CARTESIAN_POINT('Ctrl Pts',(-0.758281796766761,1.,-1.99399831098817));
#46388=CARTESIAN_POINT('Ctrl Pts',(-0.759080037802488,1.,-1.98771456680874));
#46389=CARTESIAN_POINT('Ctrl Pts',(-0.75983714745219,1.,-1.98143741418172));
#46390=CARTESIAN_POINT('Ctrl Pts',(-0.760552825409757,1.,-1.97516705321494));
#46391=CARTESIAN_POINT('Ctrl Pts',(-0.76122669048382,1.,-1.96890351582499));
#46392=CARTESIAN_POINT('Ctrl Pts',(-0.761858300014423,1.,-1.96264672744186));
#46393=CARTESIAN_POINT('Ctrl Pts',(-0.762447203806179,1.,-1.95639665309869));
#46394=CARTESIAN_POINT('Ctrl Pts',(-0.762992990878769,1.,-1.95015342590024));
#46395=CARTESIAN_POINT('Ctrl Pts',(-0.763495333538629,1.,-1.9439174661764));
#46396=CARTESIAN_POINT('Ctrl Pts',(-0.763954049121458,1.,-1.93768964875886));
#46397=CARTESIAN_POINT('Ctrl Pts',(-0.764369010673941,1.,-1.93147105496382));
#46398=CARTESIAN_POINT('Ctrl Pts',(-0.764740025488211,1.,-1.92526263537048));
#46399=CARTESIAN_POINT('Ctrl Pts',(-0.765066729667088,1.,-1.91906491634196));
#46400=CARTESIAN_POINT('Ctrl Pts',(-0.765348465884722,1.,-1.91287765805169));
#46401=CARTESIAN_POINT('Ctrl Pts',(-0.765584196937919,1.,-1.90669961402356));
#46402=CARTESIAN_POINT('Ctrl Pts',(-0.765772772593386,1.,-1.90052930393596));
#46403=CARTESIAN_POINT('Ctrl Pts',(-0.765913193856978,1.,-1.89436577771388));
#46404=CARTESIAN_POINT('Ctrl Pts',(-0.766004837062091,1.,-1.88820926433409));
#46405=CARTESIAN_POINT('Ctrl Pts',(-0.766047794851865,1.,-1.88206215302561));
#46406=CARTESIAN_POINT('Ctrl Pts',(-0.766042837036744,1.,-1.87592888967883));
#46407=CARTESIAN_POINT('Ctrl Pts',(-0.765990708546091,1.,-1.86981398314341));
#46408=CARTESIAN_POINT('Ctrl Pts',(-0.765891519092547,1.,-1.86372027063312));
#46409=CARTESIAN_POINT('Ctrl Pts',(-0.765744212909318,1.,-1.85764741390394));
#46410=CARTESIAN_POINT('Ctrl Pts',(-0.765545710619062,1.,-1.85158945130063));
#46411=CARTESIAN_POINT('Ctrl Pts',(-0.765291664862029,1.,-1.84553698875924));
#46412=CARTESIAN_POINT('Ctrl Pts',(-0.764978057881737,1.,-1.83948181064835));
#46413=CARTESIAN_POINT('Ctrl Pts',(-0.764602549687853,1.,-1.83342077227142));
#46414=CARTESIAN_POINT('Ctrl Pts',(-0.764165902605995,1.,-1.82735991200065));
#46415=CARTESIAN_POINT('Ctrl Pts',(-0.763673465462726,1.,-1.82131873145266));
#46416=CARTESIAN_POINT('Ctrl Pts',(-0.763132003836634,1.,-1.8153211840553));
#46417=CARTESIAN_POINT('Ctrl Pts',(-0.762546129463938,1.,-1.80938551463965));
#46418=CARTESIAN_POINT('Ctrl Pts',(-0.761915336443547,1.,-1.80351583877342));
#46419=CARTESIAN_POINT('Ctrl Pts',(-0.761229695230558,1.,-1.79768986997783));
#46420=CARTESIAN_POINT('Ctrl Pts',(-0.760469555880749,1.,-1.7918581561088));
#46421=CARTESIAN_POINT('Ctrl Pts',(-0.759614401110189,1.,-1.78596964884604));
#46422=CARTESIAN_POINT('Ctrl Pts',(-0.758650626677518,1.,-1.77999411220945));
#46423=CARTESIAN_POINT('Ctrl Pts',(-0.757578264077029,1.,-1.77394167108292));
#46424=CARTESIAN_POINT('Ctrl Pts',(-0.75642189602781,1.,-1.76789396002998));
#46425=CARTESIAN_POINT('Ctrl Pts',(-0.755220979974461,1.,-1.76197817240128));
#46426=CARTESIAN_POINT('Ctrl Pts',(-0.754009254027829,1.,-1.75631083600019));
#46427=CARTESIAN_POINT('Ctrl Pts',(-0.752797683531314,1.,-1.75095139468794));
#46428=CARTESIAN_POINT('Ctrl Pts',(-0.751555614164482,1.,-1.74585086852502));
#46429=CARTESIAN_POINT('Ctrl Pts',(-0.750193435981249,1.,-1.74080458267114));
#46430=CARTESIAN_POINT('Ctrl Pts',(-0.74858246295687,1.,-1.7355035168033));
#46431=CARTESIAN_POINT('Ctrl Pts',(-0.746574710097752,1.,-1.72958533647714));
#46432=CARTESIAN_POINT('Ctrl Pts',(-0.744021445433093,1.,-1.72268229916769));
#46433=CARTESIAN_POINT('Ctrl Pts',(-0.74079516202821,1.,-1.71447789751001));
#46434=CARTESIAN_POINT('Ctrl Pts',(-0.736799665716932,1.,-1.70473309004249));
#46435=CARTESIAN_POINT('Ctrl Pts',(-0.731963238685357,1.,-1.69326921972915));
#46436=CARTESIAN_POINT('Ctrl Pts',(-0.726235967982445,1.,-1.67996158451922));
#46437=CARTESIAN_POINT('Ctrl Pts',(-0.71958543378795,1.,-1.66472880551777));
#46438=CARTESIAN_POINT('Ctrl Pts',(-0.711993139340447,1.,-1.64752408828442));
#46439=CARTESIAN_POINT('Ctrl Pts',(-0.705159151977294,1.,-1.6321654166204));
#46440=CARTESIAN_POINT('Ctrl Pts',(-0.699605146398837,1.,-1.61974673471117));
#46441=CARTESIAN_POINT('Ctrl Pts',(-0.69571209787897,1.,-1.61106790957619));
#46442=CARTESIAN_POINT('Ctrl Pts',(-0.693717979106305,1.,-1.60662857109684));
#46443=CARTESIAN_POINT('',(-0.745574324794401,0.,-2.0698113262342));
#46444=CARTESIAN_POINT('Origin',(-0.61342227326009,0.,-2.11275013067528));
#46445=CARTESIAN_POINT('',(-0.61342227326009,1.,-2.11275013067528));
#46446=CARTESIAN_POINT('',(-0.745574324794401,1.,-2.0698113262342));
#46447=CARTESIAN_POINT('',(-0.61342227326009,0.,-2.11275013067528));
#46448=CARTESIAN_POINT('Ctrl Pts',(-0.383122945602004,-1.,-1.7075470150345));
#46449=CARTESIAN_POINT('Ctrl Pts',(-0.383122945602004,1.,-1.7075470150345));
#46450=CARTESIAN_POINT('Ctrl Pts',(-0.384119047315542,-1.,-1.71231062891958));
#46451=CARTESIAN_POINT('Ctrl Pts',(-0.384119047315542,1.,-1.71231062891958));
#46452=CARTESIAN_POINT('Ctrl Pts',(-0.38607079032701,-1.,-1.72162022246158));
#46453=CARTESIAN_POINT('Ctrl Pts',(-0.38607079032701,1.,-1.72162022246158));
#46454=CARTESIAN_POINT('Ctrl Pts',(-0.388877023509191,-1.,-1.7349317097561));
#46455=CARTESIAN_POINT('Ctrl Pts',(-0.388877023509191,1.,-1.7349317097561));
#46456=CARTESIAN_POINT('Ctrl Pts',(-0.392375812294307,-1.,-1.75137405313962));
#46457=CARTESIAN_POINT('Ctrl Pts',(-0.392375812294307,1.,-1.75137405313962));
#46458=CARTESIAN_POINT('Ctrl Pts',(-0.39634619612042,-1.,-1.7697556004756));
#46459=CARTESIAN_POINT('Ctrl Pts',(-0.39634619612042,1.,-1.7697556004756));
#46460=CARTESIAN_POINT('Ctrl Pts',(-0.39991940378308,-1.,-1.78598826347533));
#46461=CARTESIAN_POINT('Ctrl Pts',(-0.39991940378308,1.,-1.78598826347533));
#46462=CARTESIAN_POINT('Ctrl Pts',(-0.403107976170441,-1.,-1.80012077176221));
#46463=CARTESIAN_POINT('Ctrl Pts',(-0.403107976170441,1.,-1.80012077176221));
#46464=CARTESIAN_POINT('Ctrl Pts',(-0.405933518411838,-1.,-1.81223801813988));
#46465=CARTESIAN_POINT('Ctrl Pts',(-0.405933518411838,1.,-1.81223801813988));
#46466=CARTESIAN_POINT('Ctrl Pts',(-0.408428948108533,-1.,-1.8224702267854));
#46467=CARTESIAN_POINT('Ctrl Pts',(-0.408428948108533,1.,-1.8224702267854));
#46468=CARTESIAN_POINT('Ctrl Pts',(-0.410641256301675,-1.,-1.83100408895216));
#46469=CARTESIAN_POINT('Ctrl Pts',(-0.410641256301675,1.,-1.83100408895216));
#46470=CARTESIAN_POINT('Ctrl Pts',(-0.412633125322162,-1.,-1.83808953475839));
#46471=CARTESIAN_POINT('Ctrl Pts',(-0.412633125322162,1.,-1.83808953475839));
#46472=CARTESIAN_POINT('Ctrl Pts',(-0.41448743825434,-1.,-1.8440575707371));
#46473=CARTESIAN_POINT('Ctrl Pts',(-0.41448743825434,1.,-1.8440575707371));
#46474=CARTESIAN_POINT('Ctrl Pts',(-0.416300022038864,-1.,-1.84929312929882));
#46475=CARTESIAN_POINT('Ctrl Pts',(-0.416300022038864,1.,-1.84929312929882));
#46476=CARTESIAN_POINT('Ctrl Pts',(-0.418164129143534,-1.,-1.85417632856234));
#46477=CARTESIAN_POINT('Ctrl Pts',(-0.418164129143534,1.,-1.85417632856234));
#46478=CARTESIAN_POINT('Ctrl Pts',(-0.420157287975619,-1.,-1.85903281096686));
#46479=CARTESIAN_POINT('Ctrl Pts',(-0.420157287975619,1.,-1.85903281096686));
#46480=CARTESIAN_POINT('Ctrl Pts',(-0.422327307418275,-1.,-1.86408083334028));
#46481=CARTESIAN_POINT('Ctrl Pts',(-0.422327307418275,1.,-1.86408083334028));
#46482=CARTESIAN_POINT('Ctrl Pts',(-0.424678177291359,-1.,-1.86937803944323));
#46483=CARTESIAN_POINT('Ctrl Pts',(-0.424678177291359,1.,-1.86937803944323));
#46484=CARTESIAN_POINT('Ctrl Pts',(-0.427183828519102,-1.,-1.87486989291484));
#46485=CARTESIAN_POINT('Ctrl Pts',(-0.427183828519102,1.,-1.87486989291484));
#46486=CARTESIAN_POINT('Ctrl Pts',(-0.429803062482344,-1.,-1.88044229001832));
#46487=CARTESIAN_POINT('Ctrl Pts',(-0.429803062482344,1.,-1.88044229001832));
#46488=CARTESIAN_POINT('Ctrl Pts',(-0.432493038548748,-1.,-1.88596913666793));
#46489=CARTESIAN_POINT('Ctrl Pts',(-0.432493038548748,1.,-1.88596913666793));
#46490=CARTESIAN_POINT('Ctrl Pts',(-0.435225660963383,-1.,-1.89136993975504));
#46491=CARTESIAN_POINT('Ctrl Pts',(-0.435225660963383,1.,-1.89136993975504));
#46492=CARTESIAN_POINT('Ctrl Pts',(-0.437995003948244,-1.,-1.89663648956466));
#46493=CARTESIAN_POINT('Ctrl Pts',(-0.437995003948244,1.,-1.89663648956466));
#46494=CARTESIAN_POINT('Ctrl Pts',(-0.440807833704038,-1.,-1.90180124389086));
#46495=CARTESIAN_POINT('Ctrl Pts',(-0.440807833704038,1.,-1.90180124389086));
#46496=CARTESIAN_POINT('Ctrl Pts',(-0.443677556849151,-1.,-1.90691756144898));
#46497=CARTESIAN_POINT('Ctrl Pts',(-0.443677556849151,1.,-1.90691756144898));
#46498=CARTESIAN_POINT('Ctrl Pts',(-0.446617343485711,-1.,-1.9120369998112));
#46499=CARTESIAN_POINT('Ctrl Pts',(-0.446617343485711,1.,-1.9120369998112));
#46500=CARTESIAN_POINT('Ctrl Pts',(-0.449632260106662,-1.,-1.91718342555755));
#46501=CARTESIAN_POINT('Ctrl Pts',(-0.449632260106662,1.,-1.91718342555755));
#46502=CARTESIAN_POINT('Ctrl Pts',(-0.452719478359432,-1.,-1.92235380648502));
#46503=CARTESIAN_POINT('Ctrl Pts',(-0.452719478359432,1.,-1.92235380648502));
#46504=CARTESIAN_POINT('Ctrl Pts',(-0.455872005174371,-1.,-1.92753067150476));
#46505=CARTESIAN_POINT('Ctrl Pts',(-0.455872005174371,1.,-1.92753067150476));
#46506=CARTESIAN_POINT('Ctrl Pts',(-0.459081234547926,-1.,-1.93269066517934));
#46507=CARTESIAN_POINT('Ctrl Pts',(-0.459081234547926,1.,-1.93269066517934));
#46508=CARTESIAN_POINT('Ctrl Pts',(-0.462340031009056,-1.,-1.93781486640821));
#46509=CARTESIAN_POINT('Ctrl Pts',(-0.462340031009056,1.,-1.93781486640821));
#46510=CARTESIAN_POINT('Ctrl Pts',(-0.46564546202603,-1.,-1.9428979419619));
#46511=CARTESIAN_POINT('Ctrl Pts',(-0.46564546202603,1.,-1.9428979419619));
#46512=CARTESIAN_POINT('Ctrl Pts',(-0.468997482913135,-1.,-1.94794381136514));
#46513=CARTESIAN_POINT('Ctrl Pts',(-0.468997482913135,1.,-1.94794381136514));
#46514=CARTESIAN_POINT('Ctrl Pts',(-0.472397672264072,-1.,-1.95296148278133));
#46515=CARTESIAN_POINT('Ctrl Pts',(-0.472397672264072,1.,-1.95296148278133));
#46516=CARTESIAN_POINT('Ctrl Pts',(-0.475848034683176,-1.,-1.95796111148177));
#46517=CARTESIAN_POINT('Ctrl Pts',(-0.475848034683176,1.,-1.95796111148177));
#46518=CARTESIAN_POINT('Ctrl Pts',(-0.479349583074855,-1.,-1.96294933055943));
#46519=CARTESIAN_POINT('Ctrl Pts',(-0.479349583074855,1.,-1.96294933055943));
#46520=CARTESIAN_POINT('Ctrl Pts',(-0.482901662120691,-1.,-1.96792703422362));
#46521=CARTESIAN_POINT('Ctrl Pts',(-0.482901662120691,1.,-1.96792703422362));
#46522=CARTESIAN_POINT('Ctrl Pts',(-0.486502692907659,-1.,-1.97289186263272));
#46523=CARTESIAN_POINT('Ctrl Pts',(-0.486502692907659,1.,-1.97289186263272));
#46524=CARTESIAN_POINT('Ctrl Pts',(-0.490150627860952,-1.,-1.97783973019229));
#46525=CARTESIAN_POINT('Ctrl Pts',(-0.490150627860952,1.,-1.97783973019229));
#46526=CARTESIAN_POINT('Ctrl Pts',(-0.493843476541495,-1.,-1.98276658761821));
#46527=CARTESIAN_POINT('Ctrl Pts',(-0.493843476541495,1.,-1.98276658761821));
#46528=CARTESIAN_POINT('Ctrl Pts',(-0.497579909545574,-1.,-1.98767044752932));
#46529=CARTESIAN_POINT('Ctrl Pts',(-0.497579909545574,1.,-1.98767044752932));
#46530=CARTESIAN_POINT('Ctrl Pts',(-0.501359287727146,-1.,-1.99255149126155));
#46531=CARTESIAN_POINT('Ctrl Pts',(-0.501359287727146,1.,-1.99255149126155));
#46532=CARTESIAN_POINT('Ctrl Pts',(-0.505181361323026,-1.,-1.99741107463572));
#46533=CARTESIAN_POINT('Ctrl Pts',(-0.505181361323026,1.,-1.99741107463572));
#46534=CARTESIAN_POINT('Ctrl Pts',(-0.509046069886157,-1.,-2.00225107134734));
#46535=CARTESIAN_POINT('Ctrl Pts',(-0.509046069886157,1.,-2.00225107134734));
#46536=CARTESIAN_POINT('Ctrl Pts',(-0.512953306961792,-1.,-2.00707309946949));
#46537=CARTESIAN_POINT('Ctrl Pts',(-0.512953306961792,1.,-2.00707309946949));
#46538=CARTESIAN_POINT('Ctrl Pts',(-0.516902681728687,-1.,-2.01187773939242));
#46539=CARTESIAN_POINT('Ctrl Pts',(-0.516902681728687,1.,-2.01187773939242));
#46540=CARTESIAN_POINT('Ctrl Pts',(-0.52089359039937,-1.,-2.01666477917286));
#46541=CARTESIAN_POINT('Ctrl Pts',(-0.52089359039937,1.,-2.01666477917286));
#46542=CARTESIAN_POINT('Ctrl Pts',(-0.524925318333476,-1.,-2.02143356304698));
#46543=CARTESIAN_POINT('Ctrl Pts',(-0.524925318333476,1.,-2.02143356304698));
#46544=CARTESIAN_POINT('Ctrl Pts',(-0.528997127241914,-1.,-2.0261832908329));
#46545=CARTESIAN_POINT('Ctrl Pts',(-0.528997127241914,1.,-2.0261832908329));
#46546=CARTESIAN_POINT('Ctrl Pts',(-0.533108355132977,-1.,-2.03091336214426));
#46547=CARTESIAN_POINT('Ctrl Pts',(-0.533108355132977,1.,-2.03091336214426));
#46548=CARTESIAN_POINT('Ctrl Pts',(-0.537258489833262,-1.,-2.03562362954037));
#46549=CARTESIAN_POINT('Ctrl Pts',(-0.537258489833262,1.,-2.03562362954037));
#46550=CARTESIAN_POINT('Ctrl Pts',(-0.541447120615659,-1.,-2.04031422690527));
#46551=CARTESIAN_POINT('Ctrl Pts',(-0.541447120615659,1.,-2.04031422690527));
#46552=CARTESIAN_POINT('Ctrl Pts',(-0.54567390381743,-1.,-2.04498544714588));
#46553=CARTESIAN_POINT('Ctrl Pts',(-0.54567390381743,1.,-2.04498544714588));
#46554=CARTESIAN_POINT('Ctrl Pts',(-0.549938525150295,-1.,-2.04963761077958));
#46555=CARTESIAN_POINT('Ctrl Pts',(-0.549938525150295,1.,-2.04963761077958));
#46556=CARTESIAN_POINT('Ctrl Pts',(-0.554240657463906,-1.,-2.05427091604413));
#46557=CARTESIAN_POINT('Ctrl Pts',(-0.554240657463906,1.,-2.05427091604413));
#46558=CARTESIAN_POINT('Ctrl Pts',(-0.558579940185151,-1.,-2.05888537756462));
#46559=CARTESIAN_POINT('Ctrl Pts',(-0.558579940185151,1.,-2.05888537756462));
#46560=CARTESIAN_POINT('Ctrl Pts',(-0.562955993082261,-1.,-2.06348090160589));
#46561=CARTESIAN_POINT('Ctrl Pts',(-0.562955993082261,1.,-2.06348090160589));
#46562=CARTESIAN_POINT('Ctrl Pts',(-0.567368421181087,-1.,-2.06805732997334));
#46563=CARTESIAN_POINT('Ctrl Pts',(-0.567368421181087,1.,-2.06805732997334));
#46564=CARTESIAN_POINT('Ctrl Pts',(-0.571816823242603,-1.,-2.07261449292824));
#46565=CARTESIAN_POINT('Ctrl Pts',(-0.571816823242603,1.,-2.07261449292824));
#46566=CARTESIAN_POINT('Ctrl Pts',(-0.576300797416844,-1.,-2.07715226767559));
#46567=CARTESIAN_POINT('Ctrl Pts',(-0.576300797416844,1.,-2.07715226767559));
#46568=CARTESIAN_POINT('Ctrl Pts',(-0.580819952108063,-1.,-2.08167059018418));
#46569=CARTESIAN_POINT('Ctrl Pts',(-0.580819952108063,1.,-2.08167059018418));
#46570=CARTESIAN_POINT('Ctrl Pts',(-0.585373918991617,-1.,-2.08616943727951));
#46571=CARTESIAN_POINT('Ctrl Pts',(-0.585373918991617,1.,-2.08616943727951));
#46572=CARTESIAN_POINT('Ctrl Pts',(-0.589962365403406,-1.,-2.09064881812129));
#46573=CARTESIAN_POINT('Ctrl Pts',(-0.589962365403406,1.,-2.09064881812129));
#46574=CARTESIAN_POINT('Ctrl Pts',(-0.594585006052162,-1.,-2.0951087622027));
#46575=CARTESIAN_POINT('Ctrl Pts',(-0.594585006052162,1.,-2.0951087622027));
#46576=CARTESIAN_POINT('Ctrl Pts',(-0.599241616420533,-1.,-2.0995493086477));
#46577=CARTESIAN_POINT('Ctrl Pts',(-0.599241616420533,1.,-2.0995493086477));
#46578=CARTESIAN_POINT('Ctrl Pts',(-0.60393203073603,-1.,-2.10397049886949));
#46579=CARTESIAN_POINT('Ctrl Pts',(-0.60393203073603,1.,-2.10397049886949));
#46580=CARTESIAN_POINT('Ctrl Pts',(-0.607711315454876,-1.,-2.1074919961518));
#46581=CARTESIAN_POINT('Ctrl Pts',(-0.607711315454876,1.,-2.1074919961518));
#46582=CARTESIAN_POINT('Ctrl Pts',(-0.610560911689899,-1.,-2.11012443807238));
#46583=CARTESIAN_POINT('Ctrl Pts',(-0.610560911689899,1.,-2.11012443807238));
#46584=CARTESIAN_POINT('Ctrl Pts',(-0.6124673655618,-1.,-2.11187554259986));
#46585=CARTESIAN_POINT('Ctrl Pts',(-0.6124673655618,1.,-2.11187554259986));
#46586=CARTESIAN_POINT('Ctrl Pts',(-0.61342227326009,-1.,-2.11275013067528));
#46587=CARTESIAN_POINT('Ctrl Pts',(-0.61342227326009,1.,-2.11275013067528));
#46588=CARTESIAN_POINT('',(-0.383122945602004,1.,-1.7075470150345));
#46589=CARTESIAN_POINT('Ctrl Pts',(-0.383122945602004,1.,-1.7075470150345));
#46590=CARTESIAN_POINT('Ctrl Pts',(-0.384119047315542,1.,-1.71231062891958));
#46591=CARTESIAN_POINT('Ctrl Pts',(-0.38607079032701,1.,-1.72162022246158));
#46592=CARTESIAN_POINT('Ctrl Pts',(-0.388877023509191,1.,-1.7349317097561));
#46593=CARTESIAN_POINT('Ctrl Pts',(-0.392375812294307,1.,-1.75137405313962));
#46594=CARTESIAN_POINT('Ctrl Pts',(-0.39634619612042,1.,-1.7697556004756));
#46595=CARTESIAN_POINT('Ctrl Pts',(-0.39991940378308,1.,-1.78598826347533));
#46596=CARTESIAN_POINT('Ctrl Pts',(-0.403107976170441,1.,-1.80012077176221));
#46597=CARTESIAN_POINT('Ctrl Pts',(-0.405933518411838,1.,-1.81223801813988));
#46598=CARTESIAN_POINT('Ctrl Pts',(-0.408428948108533,1.,-1.8224702267854));
#46599=CARTESIAN_POINT('Ctrl Pts',(-0.410641256301675,1.,-1.83100408895216));
#46600=CARTESIAN_POINT('Ctrl Pts',(-0.412633125322162,1.,-1.83808953475839));
#46601=CARTESIAN_POINT('Ctrl Pts',(-0.41448743825434,1.,-1.8440575707371));
#46602=CARTESIAN_POINT('Ctrl Pts',(-0.416300022038864,1.,-1.84929312929882));
#46603=CARTESIAN_POINT('Ctrl Pts',(-0.418164129143534,1.,-1.85417632856234));
#46604=CARTESIAN_POINT('Ctrl Pts',(-0.420157287975619,1.,-1.85903281096686));
#46605=CARTESIAN_POINT('Ctrl Pts',(-0.422327307418275,1.,-1.86408083334028));
#46606=CARTESIAN_POINT('Ctrl Pts',(-0.424678177291359,1.,-1.86937803944323));
#46607=CARTESIAN_POINT('Ctrl Pts',(-0.427183828519102,1.,-1.87486989291484));
#46608=CARTESIAN_POINT('Ctrl Pts',(-0.429803062482344,1.,-1.88044229001832));
#46609=CARTESIAN_POINT('Ctrl Pts',(-0.432493038548748,1.,-1.88596913666793));
#46610=CARTESIAN_POINT('Ctrl Pts',(-0.435225660963383,1.,-1.89136993975504));
#46611=CARTESIAN_POINT('Ctrl Pts',(-0.437995003948244,1.,-1.89663648956466));
#46612=CARTESIAN_POINT('Ctrl Pts',(-0.440807833704038,1.,-1.90180124389086));
#46613=CARTESIAN_POINT('Ctrl Pts',(-0.443677556849151,1.,-1.90691756144898));
#46614=CARTESIAN_POINT('Ctrl Pts',(-0.446617343485711,1.,-1.9120369998112));
#46615=CARTESIAN_POINT('Ctrl Pts',(-0.449632260106662,1.,-1.91718342555755));
#46616=CARTESIAN_POINT('Ctrl Pts',(-0.452719478359432,1.,-1.92235380648502));
#46617=CARTESIAN_POINT('Ctrl Pts',(-0.455872005174371,1.,-1.92753067150476));
#46618=CARTESIAN_POINT('Ctrl Pts',(-0.459081234547926,1.,-1.93269066517934));
#46619=CARTESIAN_POINT('Ctrl Pts',(-0.462340031009056,1.,-1.93781486640821));
#46620=CARTESIAN_POINT('Ctrl Pts',(-0.46564546202603,1.,-1.9428979419619));
#46621=CARTESIAN_POINT('Ctrl Pts',(-0.468997482913135,1.,-1.94794381136514));
#46622=CARTESIAN_POINT('Ctrl Pts',(-0.472397672264072,1.,-1.95296148278133));
#46623=CARTESIAN_POINT('Ctrl Pts',(-0.475848034683176,1.,-1.95796111148177));
#46624=CARTESIAN_POINT('Ctrl Pts',(-0.479349583074855,1.,-1.96294933055943));
#46625=CARTESIAN_POINT('Ctrl Pts',(-0.482901662120691,1.,-1.96792703422362));
#46626=CARTESIAN_POINT('Ctrl Pts',(-0.486502692907659,1.,-1.97289186263272));
#46627=CARTESIAN_POINT('Ctrl Pts',(-0.490150627860952,1.,-1.97783973019229));
#46628=CARTESIAN_POINT('Ctrl Pts',(-0.493843476541495,1.,-1.98276658761821));
#46629=CARTESIAN_POINT('Ctrl Pts',(-0.497579909545574,1.,-1.98767044752932));
#46630=CARTESIAN_POINT('Ctrl Pts',(-0.501359287727146,1.,-1.99255149126155));
#46631=CARTESIAN_POINT('Ctrl Pts',(-0.505181361323026,1.,-1.99741107463572));
#46632=CARTESIAN_POINT('Ctrl Pts',(-0.509046069886157,1.,-2.00225107134734));
#46633=CARTESIAN_POINT('Ctrl Pts',(-0.512953306961792,1.,-2.00707309946949));
#46634=CARTESIAN_POINT('Ctrl Pts',(-0.516902681728687,1.,-2.01187773939242));
#46635=CARTESIAN_POINT('Ctrl Pts',(-0.52089359039937,1.,-2.01666477917286));
#46636=CARTESIAN_POINT('Ctrl Pts',(-0.524925318333476,1.,-2.02143356304698));
#46637=CARTESIAN_POINT('Ctrl Pts',(-0.528997127241914,1.,-2.0261832908329));
#46638=CARTESIAN_POINT('Ctrl Pts',(-0.533108355132977,1.,-2.03091336214426));
#46639=CARTESIAN_POINT('Ctrl Pts',(-0.537258489833262,1.,-2.03562362954037));
#46640=CARTESIAN_POINT('Ctrl Pts',(-0.541447120615659,1.,-2.04031422690527));
#46641=CARTESIAN_POINT('Ctrl Pts',(-0.54567390381743,1.,-2.04498544714588));
#46642=CARTESIAN_POINT('Ctrl Pts',(-0.549938525150295,1.,-2.04963761077958));
#46643=CARTESIAN_POINT('Ctrl Pts',(-0.554240657463906,1.,-2.05427091604413));
#46644=CARTESIAN_POINT('Ctrl Pts',(-0.558579940185151,1.,-2.05888537756462));
#46645=CARTESIAN_POINT('Ctrl Pts',(-0.562955993082261,1.,-2.06348090160589));
#46646=CARTESIAN_POINT('Ctrl Pts',(-0.567368421181087,1.,-2.06805732997334));
#46647=CARTESIAN_POINT('Ctrl Pts',(-0.571816823242603,1.,-2.07261449292824));
#46648=CARTESIAN_POINT('Ctrl Pts',(-0.576300797416844,1.,-2.07715226767559));
#46649=CARTESIAN_POINT('Ctrl Pts',(-0.580819952108063,1.,-2.08167059018418));
#46650=CARTESIAN_POINT('Ctrl Pts',(-0.585373918991617,1.,-2.08616943727951));
#46651=CARTESIAN_POINT('Ctrl Pts',(-0.589962365403406,1.,-2.09064881812129));
#46652=CARTESIAN_POINT('Ctrl Pts',(-0.594585006052162,1.,-2.0951087622027));
#46653=CARTESIAN_POINT('Ctrl Pts',(-0.599241616420533,1.,-2.0995493086477));
#46654=CARTESIAN_POINT('Ctrl Pts',(-0.60393203073603,1.,-2.10397049886949));
#46655=CARTESIAN_POINT('Ctrl Pts',(-0.607711315454876,1.,-2.1074919961518));
#46656=CARTESIAN_POINT('Ctrl Pts',(-0.610560911689899,1.,-2.11012443807238));
#46657=CARTESIAN_POINT('Ctrl Pts',(-0.6124673655618,1.,-2.11187554259986));
#46658=CARTESIAN_POINT('Ctrl Pts',(-0.61342227326009,1.,-2.11275013067528));
#46659=CARTESIAN_POINT('',(-0.383122945602003,0.,-1.7075470150345));
#46660=CARTESIAN_POINT('Origin',(0.,0.,0.));
#46661=CARTESIAN_POINT('',(-0.163289472382896,1.,-1.74236521665491));
#46662=CARTESIAN_POINT('Origin',(0.,1.,0.));
#46663=CARTESIAN_POINT('',(-0.163289472382896,0.,-1.74236521665491));
#46664=CARTESIAN_POINT('Ctrl Pts',(-0.0694764450219581,-1.,-2.19890268624765));
#46665=CARTESIAN_POINT('Ctrl Pts',(-0.0694764450219581,1.,-2.19890268624765));
#46666=CARTESIAN_POINT('Ctrl Pts',(-0.070114353632549,-1.,-2.19777582085423));
#46667=CARTESIAN_POINT('Ctrl Pts',(-0.070114353632549,1.,-2.19777582085423));
#46668=CARTESIAN_POINT('Ctrl Pts',(-0.0713863779526154,-1.,-2.19552129484002));
#46669=CARTESIAN_POINT('Ctrl Pts',(-0.0713863779526154,1.,-2.19552129484002));
#46670=CARTESIAN_POINT('Ctrl Pts',(-0.0732830357306725,-1.,-2.19213712013662));
#46671=CARTESIAN_POINT('Ctrl Pts',(-0.0732830357306725,1.,-2.19213712013662));
#46672=CARTESIAN_POINT('Ctrl Pts',(-0.0757891465836148,-1.,-2.1876201139953));
#46673=CARTESIAN_POINT('Ctrl Pts',(-0.0757891465836148,1.,-2.1876201139953));
#46674=CARTESIAN_POINT('Ctrl Pts',(-0.0788837727685243,-1.,-2.18196589448887));
#46675=CARTESIAN_POINT('Ctrl Pts',(-0.0788837727685243,1.,-2.18196589448887));
#46676=CARTESIAN_POINT('Ctrl Pts',(-0.0819402680872765,-1.,-2.176303712113));
#46677=CARTESIAN_POINT('Ctrl Pts',(-0.0819402680872765,1.,-2.176303712113));
#46678=CARTESIAN_POINT('Ctrl Pts',(-0.0849584620835372,-1.,-2.17063357870952));
#46679=CARTESIAN_POINT('Ctrl Pts',(-0.0849584620835372,1.,-2.17063357870952));
#46680=CARTESIAN_POINT('Ctrl Pts',(-0.0879381291386923,-1.,-2.16495552645014));
#46681=CARTESIAN_POINT('Ctrl Pts',(-0.0879381291386923,1.,-2.16495552645014));
#46682=CARTESIAN_POINT('Ctrl Pts',(-0.0908789888107265,-1.,-2.15926961544516));
#46683=CARTESIAN_POINT('Ctrl Pts',(-0.0908789888107265,1.,-2.15926961544516));
#46684=CARTESIAN_POINT('Ctrl Pts',(-0.0937807218867643,-1.,-2.1535759397817));
#46685=CARTESIAN_POINT('Ctrl Pts',(-0.0937807218867643,1.,-2.1535759397817));
#46686=CARTESIAN_POINT('Ctrl Pts',(-0.0966429852305459,-1.,-2.14787463531795));
#46687=CARTESIAN_POINT('Ctrl Pts',(-0.0966429852305459,1.,-2.14787463531795));
#46688=CARTESIAN_POINT('Ctrl Pts',(-0.0994654261990915,-1.,-2.14216588396025));
#46689=CARTESIAN_POINT('Ctrl Pts',(-0.0994654261990915,1.,-2.14216588396025));
#46690=CARTESIAN_POINT('Ctrl Pts',(-0.1022477005561,-1.,-2.13644992667165));
#46691=CARTESIAN_POINT('Ctrl Pts',(-0.1022477005561,1.,-2.13644992667165));
#46692=CARTESIAN_POINT('Ctrl Pts',(-0.104989479152739,-1.,-2.13072704887293));
#46693=CARTESIAN_POINT('Ctrl Pts',(-0.104989479152739,1.,-2.13072704887293));
#46694=CARTESIAN_POINT('Ctrl Pts',(-0.10769043523109,-1.,-2.12499752307));
#46695=CARTESIAN_POINT('Ctrl Pts',(-0.10769043523109,1.,-2.12499752307));
#46696=CARTESIAN_POINT('Ctrl Pts',(-0.110350236135025,-1.,-2.11926155590865));
#46697=CARTESIAN_POINT('Ctrl Pts',(-0.110350236135025,1.,-2.11926155590865));
#46698=CARTESIAN_POINT('Ctrl Pts',(-0.112968534419737,-1.,-2.11351924490306));
#46699=CARTESIAN_POINT('Ctrl Pts',(-0.112968534419737,1.,-2.11351924490306));
#46700=CARTESIAN_POINT('Ctrl Pts',(-0.115544957687926,-1.,-2.10777050261309));
#46701=CARTESIAN_POINT('Ctrl Pts',(-0.115544957687926,1.,-2.10777050261309));
#46702=CARTESIAN_POINT('Ctrl Pts',(-0.118079107988355,-1.,-2.102015121329));
#46703=CARTESIAN_POINT('Ctrl Pts',(-0.118079107988355,1.,-2.102015121329));
#46704=CARTESIAN_POINT('Ctrl Pts',(-0.120570567965122,-1.,-2.0962529286773));
#46705=CARTESIAN_POINT('Ctrl Pts',(-0.120570567965122,1.,-2.0962529286773));
#46706=CARTESIAN_POINT('Ctrl Pts',(-0.123018905621083,-1.,-2.09048392424825));
#46707=CARTESIAN_POINT('Ctrl Pts',(-0.123018905621083,1.,-2.09048392424825));
#46708=CARTESIAN_POINT('Ctrl Pts',(-0.125423679412061,-1.,-2.08470840653643));
#46709=CARTESIAN_POINT('Ctrl Pts',(-0.125423679412061,1.,-2.08470840653643));
#46710=CARTESIAN_POINT('Ctrl Pts',(-0.12778444527612,-1.,-2.07892715110987));
#46711=CARTESIAN_POINT('Ctrl Pts',(-0.12778444527612,1.,-2.07892715110987));
#46712=CARTESIAN_POINT('Ctrl Pts',(-0.130100748328403,-1.,-2.07314114713063));
#46713=CARTESIAN_POINT('Ctrl Pts',(-0.130100748328403,1.,-2.07314114713063));
#46714=CARTESIAN_POINT('Ctrl Pts',(-0.13237211154771,-1.,-2.06735123910326));
#46715=CARTESIAN_POINT('Ctrl Pts',(-0.13237211154771,1.,-2.06735123910326));
#46716=CARTESIAN_POINT('Ctrl Pts',(-0.134598026192106,-1.,-2.06155781517842));
#46717=CARTESIAN_POINT('Ctrl Pts',(-0.134598026192106,1.,-2.06155781517842));
#46718=CARTESIAN_POINT('Ctrl Pts',(-0.136777941218044,-1.,-2.05576044414264));
#46719=CARTESIAN_POINT('Ctrl Pts',(-0.136777941218044,1.,-2.05576044414264));
#46720=CARTESIAN_POINT('Ctrl Pts',(-0.138911255368966,-1.,-2.04995762001328));
#46721=CARTESIAN_POINT('Ctrl Pts',(-0.138911255368966,1.,-2.04995762001328));
#46722=CARTESIAN_POINT('Ctrl Pts',(-0.140997332152546,-1.,-2.04414757947916));
#46723=CARTESIAN_POINT('Ctrl Pts',(-0.140997332152546,1.,-2.04414757947916));
#46724=CARTESIAN_POINT('Ctrl Pts',(-0.143035515058209,-1.,-2.03832911025912));
#46725=CARTESIAN_POINT('Ctrl Pts',(-0.143035515058209,1.,-2.03832911025912));
#46726=CARTESIAN_POINT('Ctrl Pts',(-0.145025140186057,-1.,-2.03250223739942));
#46727=CARTESIAN_POINT('Ctrl Pts',(-0.145025140186057,1.,-2.03250223739942));
#46728=CARTESIAN_POINT('Ctrl Pts',(-0.146965557332583,-1.,-2.02666926182017));
#46729=CARTESIAN_POINT('Ctrl Pts',(-0.146965557332583,1.,-2.02666926182017));
#46730=CARTESIAN_POINT('Ctrl Pts',(-0.148856124775337,-1.,-2.02083464969894));
#46731=CARTESIAN_POINT('Ctrl Pts',(-0.148856124775337,1.,-2.02083464969894));
#46732=CARTESIAN_POINT('Ctrl Pts',(-0.150696157673078,-1.,-2.01500291940238));
#46733=CARTESIAN_POINT('Ctrl Pts',(-0.150696157673078,1.,-2.01500291940238));
#46734=CARTESIAN_POINT('Ctrl Pts',(-0.15248488362145,-1.,-2.00917680318424));
#46735=CARTESIAN_POINT('Ctrl Pts',(-0.15248488362145,1.,-2.00917680318424));
#46736=CARTESIAN_POINT('Ctrl Pts',(-0.154221403049722,-1.,-2.00335565310543));
#46737=CARTESIAN_POINT('Ctrl Pts',(-0.154221403049722,1.,-2.00335565310543));
#46738=CARTESIAN_POINT('Ctrl Pts',(-0.155904629548783,-1.,-1.99753284771497));
#46739=CARTESIAN_POINT('Ctrl Pts',(-0.155904629548783,1.,-1.99753284771497));
#46740=CARTESIAN_POINT('Ctrl Pts',(-0.157533331459227,-1.,-1.99169810931908));
#46741=CARTESIAN_POINT('Ctrl Pts',(-0.157533331459227,1.,-1.99169810931908));
#46742=CARTESIAN_POINT('Ctrl Pts',(-0.159106226437299,-1.,-1.98584238283292));
#46743=CARTESIAN_POINT('Ctrl Pts',(-0.159106226437299,1.,-1.98584238283292));
#46744=CARTESIAN_POINT('Ctrl Pts',(-0.160622060784611,-1.,-1.97996195437559));
#46745=CARTESIAN_POINT('Ctrl Pts',(-0.160622060784611,1.,-1.97996195437559));
#46746=CARTESIAN_POINT('Ctrl Pts',(-0.162079693556289,-1.,-1.97406280235188));
#46747=CARTESIAN_POINT('Ctrl Pts',(-0.162079693556289,1.,-1.97406280235188));
#46748=CARTESIAN_POINT('Ctrl Pts',(-0.163478185457734,-1.,-1.96816512677967));
#46749=CARTESIAN_POINT('Ctrl Pts',(-0.163478185457734,1.,-1.96816512677967));
#46750=CARTESIAN_POINT('Ctrl Pts',(-0.164816568920269,-1.,-1.96229379940136));
#46751=CARTESIAN_POINT('Ctrl Pts',(-0.164816568920269,1.,-1.96229379940136));
#46752=CARTESIAN_POINT('Ctrl Pts',(-0.166093592002812,-1.,-1.9564675971873));
#46753=CARTESIAN_POINT('Ctrl Pts',(-0.166093592002812,1.,-1.9564675971873));
#46754=CARTESIAN_POINT('Ctrl Pts',(-0.167307501784475,-1.,-1.95069027794294));
#46755=CARTESIAN_POINT('Ctrl Pts',(-0.167307501784475,1.,-1.95069027794294));
#46756=CARTESIAN_POINT('Ctrl Pts',(-0.168455741607556,-1.,-1.94493757756931));
#46757=CARTESIAN_POINT('Ctrl Pts',(-0.168455741607556,1.,-1.94493757756931));
#46758=CARTESIAN_POINT('Ctrl Pts',(-0.169534904817491,-1.,-1.93915639211581));
#46759=CARTESIAN_POINT('Ctrl Pts',(-0.169534904817491,1.,-1.93915639211581));
#46760=CARTESIAN_POINT('Ctrl Pts',(-0.170541253116202,-1.,-1.93329183155539));
#46761=CARTESIAN_POINT('Ctrl Pts',(-0.170541253116202,1.,-1.93329183155539));
#46762=CARTESIAN_POINT('Ctrl Pts',(-0.171471191532988,-1.,-1.92731093582036));
#46763=CARTESIAN_POINT('Ctrl Pts',(-0.171471191532988,1.,-1.92731093582036));
#46764=CARTESIAN_POINT('Ctrl Pts',(-0.172321621259514,-1.,-1.9212233439798));
#46765=CARTESIAN_POINT('Ctrl Pts',(-0.172321621259514,1.,-1.9212233439798));
#46766=CARTESIAN_POINT('Ctrl Pts',(-0.173090695383496,-1.,-1.91511429159527));
#46767=CARTESIAN_POINT('Ctrl Pts',(-0.173090695383496,1.,-1.91511429159527));
#46768=CARTESIAN_POINT('Ctrl Pts',(-0.173776635257817,-1.,-1.90911693975267));
#46769=CARTESIAN_POINT('Ctrl Pts',(-0.173776635257817,1.,-1.90911693975267));
#46770=CARTESIAN_POINT('Ctrl Pts',(-0.174375518661085,-1.,-1.90335253862834));
#46771=CARTESIAN_POINT('Ctrl Pts',(-0.174375518661085,1.,-1.90335253862834));
#46772=CARTESIAN_POINT('Ctrl Pts',(-0.174879405091263,-1.,-1.89788101117132));
#46773=CARTESIAN_POINT('Ctrl Pts',(-0.174879405091263,1.,-1.89788101117132));
#46774=CARTESIAN_POINT('Ctrl Pts',(-0.175274276190844,-1.,-1.892646301985));
#46775=CARTESIAN_POINT('Ctrl Pts',(-0.175274276190844,1.,-1.892646301985));
#46776=CARTESIAN_POINT('Ctrl Pts',(-0.175538155840648,-1.,-1.88742606273259));
#46777=CARTESIAN_POINT('Ctrl Pts',(-0.175538155840648,1.,-1.88742606273259));
#46778=CARTESIAN_POINT('Ctrl Pts',(-0.175644148889699,-1.,-1.88188663145367));
#46779=CARTESIAN_POINT('Ctrl Pts',(-0.175644148889699,1.,-1.88188663145367));
#46780=CARTESIAN_POINT('Ctrl Pts',(-0.175563480746485,-1.,-1.87563767773588));
#46781=CARTESIAN_POINT('Ctrl Pts',(-0.175563480746485,1.,-1.87563767773588));
#46782=CARTESIAN_POINT('Ctrl Pts',(-0.175268337590758,-1.,-1.86828349694799));
#46783=CARTESIAN_POINT('Ctrl Pts',(-0.175268337590758,1.,-1.86828349694799));
#46784=CARTESIAN_POINT('Ctrl Pts',(-0.17473525927603,-1.,-1.85948367088837));
#46785=CARTESIAN_POINT('Ctrl Pts',(-0.17473525927603,1.,-1.85948367088837));
#46786=CARTESIAN_POINT('Ctrl Pts',(-0.173946627587731,-1.,-1.8489811319852));
#46787=CARTESIAN_POINT('Ctrl Pts',(-0.173946627587731,1.,-1.8489811319852));
#46788=CARTESIAN_POINT('Ctrl Pts',(-0.1728894428919,-1.,-1.83658380527692));
#46789=CARTESIAN_POINT('Ctrl Pts',(-0.1728894428919,1.,-1.83658380527692));
#46790=CARTESIAN_POINT('Ctrl Pts',(-0.171554770204119,-1.,-1.82215766811545));
#46791=CARTESIAN_POINT('Ctrl Pts',(-0.171554770204119,1.,-1.82215766811545));
#46792=CARTESIAN_POINT('Ctrl Pts',(-0.169936923904608,-1.,-1.80561530629706));
#46793=CARTESIAN_POINT('Ctrl Pts',(-0.169936923904608,1.,-1.80561530629706));
#46794=CARTESIAN_POINT('Ctrl Pts',(-0.168032772805197,-1.,-1.7869064998507));
#46795=CARTESIAN_POINT('Ctrl Pts',(-0.168032772805197,1.,-1.7869064998507));
#46796=CARTESIAN_POINT('Ctrl Pts',(-0.1662793551464,-1.,-1.77018771684844));
#46797=CARTESIAN_POINT('Ctrl Pts',(-0.1662793551464,1.,-1.77018771684844));
#46798=CARTESIAN_POINT('Ctrl Pts',(-0.164834765707158,-1.,-1.75666056638427));
#46799=CARTESIAN_POINT('Ctrl Pts',(-0.164834765707158,1.,-1.75666056638427));
#46800=CARTESIAN_POINT('Ctrl Pts',(-0.163814161002002,-1.,-1.7472034950333));
#46801=CARTESIAN_POINT('Ctrl Pts',(-0.163814161002002,1.,-1.7472034950333));
#46802=CARTESIAN_POINT('Ctrl Pts',(-0.163289472382896,-1.,-1.74236521665491));
#46803=CARTESIAN_POINT('Ctrl Pts',(-0.163289472382896,1.,-1.74236521665491));
#46804=CARTESIAN_POINT('',(-0.0694764450219581,1.,-2.19890268624765));
#46805=CARTESIAN_POINT('Ctrl Pts',(-0.0694764450219581,1.,-2.19890268624765));
#46806=CARTESIAN_POINT('Ctrl Pts',(-0.070114353632549,1.,-2.19777582085423));
#46807=CARTESIAN_POINT('Ctrl Pts',(-0.0713863779526154,1.,-2.19552129484002));
#46808=CARTESIAN_POINT('Ctrl Pts',(-0.0732830357306725,1.,-2.19213712013662));
#46809=CARTESIAN_POINT('Ctrl Pts',(-0.0757891465836148,1.,-2.1876201139953));
#46810=CARTESIAN_POINT('Ctrl Pts',(-0.0788837727685243,1.,-2.18196589448887));
#46811=CARTESIAN_POINT('Ctrl Pts',(-0.0819402680872765,1.,-2.176303712113));
#46812=CARTESIAN_POINT('Ctrl Pts',(-0.0849584620835372,1.,-2.17063357870952));
#46813=CARTESIAN_POINT('Ctrl Pts',(-0.0879381291386923,1.,-2.16495552645014));
#46814=CARTESIAN_POINT('Ctrl Pts',(-0.0908789888107265,1.,-2.15926961544516));
#46815=CARTESIAN_POINT('Ctrl Pts',(-0.0937807218867643,1.,-2.1535759397817));
#46816=CARTESIAN_POINT('Ctrl Pts',(-0.0966429852305459,1.,-2.14787463531795));
#46817=CARTESIAN_POINT('Ctrl Pts',(-0.0994654261990915,1.,-2.14216588396025));
#46818=CARTESIAN_POINT('Ctrl Pts',(-0.1022477005561,1.,-2.13644992667165));
#46819=CARTESIAN_POINT('Ctrl Pts',(-0.104989479152739,1.,-2.13072704887293));
#46820=CARTESIAN_POINT('Ctrl Pts',(-0.10769043523109,1.,-2.12499752307));
#46821=CARTESIAN_POINT('Ctrl Pts',(-0.110350236135025,1.,-2.11926155590865));
#46822=CARTESIAN_POINT('Ctrl Pts',(-0.112968534419737,1.,-2.11351924490306));
#46823=CARTESIAN_POINT('Ctrl Pts',(-0.115544957687926,1.,-2.10777050261309));
#46824=CARTESIAN_POINT('Ctrl Pts',(-0.118079107988355,1.,-2.102015121329));
#46825=CARTESIAN_POINT('Ctrl Pts',(-0.120570567965122,1.,-2.0962529286773));
#46826=CARTESIAN_POINT('Ctrl Pts',(-0.123018905621083,1.,-2.09048392424825));
#46827=CARTESIAN_POINT('Ctrl Pts',(-0.125423679412061,1.,-2.08470840653643));
#46828=CARTESIAN_POINT('Ctrl Pts',(-0.12778444527612,1.,-2.07892715110987));
#46829=CARTESIAN_POINT('Ctrl Pts',(-0.130100748328403,1.,-2.07314114713063));
#46830=CARTESIAN_POINT('Ctrl Pts',(-0.13237211154771,1.,-2.06735123910326));
#46831=CARTESIAN_POINT('Ctrl Pts',(-0.134598026192106,1.,-2.06155781517842));
#46832=CARTESIAN_POINT('Ctrl Pts',(-0.136777941218044,1.,-2.05576044414264));
#46833=CARTESIAN_POINT('Ctrl Pts',(-0.138911255368966,1.,-2.04995762001328));
#46834=CARTESIAN_POINT('Ctrl Pts',(-0.140997332152546,1.,-2.04414757947916));
#46835=CARTESIAN_POINT('Ctrl Pts',(-0.143035515058209,1.,-2.03832911025912));
#46836=CARTESIAN_POINT('Ctrl Pts',(-0.145025140186057,1.,-2.03250223739942));
#46837=CARTESIAN_POINT('Ctrl Pts',(-0.146965557332583,1.,-2.02666926182017));
#46838=CARTESIAN_POINT('Ctrl Pts',(-0.148856124775337,1.,-2.02083464969894));
#46839=CARTESIAN_POINT('Ctrl Pts',(-0.150696157673078,1.,-2.01500291940238));
#46840=CARTESIAN_POINT('Ctrl Pts',(-0.15248488362145,1.,-2.00917680318424));
#46841=CARTESIAN_POINT('Ctrl Pts',(-0.154221403049722,1.,-2.00335565310543));
#46842=CARTESIAN_POINT('Ctrl Pts',(-0.155904629548783,1.,-1.99753284771497));
#46843=CARTESIAN_POINT('Ctrl Pts',(-0.157533331459227,1.,-1.99169810931908));
#46844=CARTESIAN_POINT('Ctrl Pts',(-0.159106226437299,1.,-1.98584238283292));
#46845=CARTESIAN_POINT('Ctrl Pts',(-0.160622060784611,1.,-1.97996195437559));
#46846=CARTESIAN_POINT('Ctrl Pts',(-0.162079693556289,1.,-1.97406280235188));
#46847=CARTESIAN_POINT('Ctrl Pts',(-0.163478185457734,1.,-1.96816512677967));
#46848=CARTESIAN_POINT('Ctrl Pts',(-0.164816568920269,1.,-1.96229379940136));
#46849=CARTESIAN_POINT('Ctrl Pts',(-0.166093592002812,1.,-1.9564675971873));
#46850=CARTESIAN_POINT('Ctrl Pts',(-0.167307501784475,1.,-1.95069027794294));
#46851=CARTESIAN_POINT('Ctrl Pts',(-0.168455741607556,1.,-1.94493757756931));
#46852=CARTESIAN_POINT('Ctrl Pts',(-0.169534904817491,1.,-1.93915639211581));
#46853=CARTESIAN_POINT('Ctrl Pts',(-0.170541253116202,1.,-1.93329183155539));
#46854=CARTESIAN_POINT('Ctrl Pts',(-0.171471191532988,1.,-1.92731093582036));
#46855=CARTESIAN_POINT('Ctrl Pts',(-0.172321621259514,1.,-1.9212233439798));
#46856=CARTESIAN_POINT('Ctrl Pts',(-0.173090695383496,1.,-1.91511429159527));
#46857=CARTESIAN_POINT('Ctrl Pts',(-0.173776635257817,1.,-1.90911693975267));
#46858=CARTESIAN_POINT('Ctrl Pts',(-0.174375518661085,1.,-1.90335253862834));
#46859=CARTESIAN_POINT('Ctrl Pts',(-0.174879405091263,1.,-1.89788101117132));
#46860=CARTESIAN_POINT('Ctrl Pts',(-0.175274276190844,1.,-1.892646301985));
#46861=CARTESIAN_POINT('Ctrl Pts',(-0.175538155840648,1.,-1.88742606273259));
#46862=CARTESIAN_POINT('Ctrl Pts',(-0.175644148889699,1.,-1.88188663145367));
#46863=CARTESIAN_POINT('Ctrl Pts',(-0.175563480746485,1.,-1.87563767773588));
#46864=CARTESIAN_POINT('Ctrl Pts',(-0.175268337590758,1.,-1.86828349694799));
#46865=CARTESIAN_POINT('Ctrl Pts',(-0.17473525927603,1.,-1.85948367088837));
#46866=CARTESIAN_POINT('Ctrl Pts',(-0.173946627587731,1.,-1.8489811319852));
#46867=CARTESIAN_POINT('Ctrl Pts',(-0.1728894428919,1.,-1.83658380527692));
#46868=CARTESIAN_POINT('Ctrl Pts',(-0.171554770204119,1.,-1.82215766811545));
#46869=CARTESIAN_POINT('Ctrl Pts',(-0.169936923904608,1.,-1.80561530629706));
#46870=CARTESIAN_POINT('Ctrl Pts',(-0.168032772805197,1.,-1.7869064998507));
#46871=CARTESIAN_POINT('Ctrl Pts',(-0.1662793551464,1.,-1.77018771684844));
#46872=CARTESIAN_POINT('Ctrl Pts',(-0.164834765707158,1.,-1.75666056638427));
#46873=CARTESIAN_POINT('Ctrl Pts',(-0.163814161002002,1.,-1.7472034950333));
#46874=CARTESIAN_POINT('Ctrl Pts',(-0.163289472382896,1.,-1.74236521665491));
#46875=CARTESIAN_POINT('',(-0.0694764450219581,0.,-2.19890268624765));
#46876=CARTESIAN_POINT('Origin',(0.0694764450219584,0.,-2.19890268624765));
#46877=CARTESIAN_POINT('',(0.0694764450219584,1.,-2.19890268624765));
#46878=CARTESIAN_POINT('',(-0.0694764450219581,1.,-2.19890268624765));
#46879=CARTESIAN_POINT('',(0.0694764450219584,0.,-2.19890268624765));
#46880=CARTESIAN_POINT('Ctrl Pts',(0.163289472382896,-1.,-1.74236521665491));
#46881=CARTESIAN_POINT('Ctrl Pts',(0.163289472382896,1.,-1.74236521665491));
#46882=CARTESIAN_POINT('Ctrl Pts',(0.163814161002474,-1.,-1.74720349503904));
#46883=CARTESIAN_POINT('Ctrl Pts',(0.163814161002474,1.,-1.74720349503904));
#46884=CARTESIAN_POINT('Ctrl Pts',(0.164834765708484,-1.,-1.75666056640041));
#46885=CARTESIAN_POINT('Ctrl Pts',(0.164834765708484,1.,-1.75666056640041));
#46886=CARTESIAN_POINT('Ctrl Pts',(0.166279355148738,-1.,-1.77018771687692));
#46887=CARTESIAN_POINT('Ctrl Pts',(0.166279355148738,1.,-1.77018771687692));
#46888=CARTESIAN_POINT('Ctrl Pts',(0.16803277280837,-1.,-1.78690649988931));
#46889=CARTESIAN_POINT('Ctrl Pts',(0.16803277280837,1.,-1.78690649988931));
#46890=CARTESIAN_POINT('Ctrl Pts',(0.169936923908078,-1.,-1.80561530633924));
#46891=CARTESIAN_POINT('Ctrl Pts',(0.169936923908078,1.,-1.80561530633924));
#46892=CARTESIAN_POINT('Ctrl Pts',(0.171554770207306,-1.,-1.82215766815414));
#46893=CARTESIAN_POINT('Ctrl Pts',(0.171554770207306,1.,-1.82215766815414));
#46894=CARTESIAN_POINT('Ctrl Pts',(0.17288944289442,-1.,-1.83658380530747));
#46895=CARTESIAN_POINT('Ctrl Pts',(0.17288944289442,1.,-1.83658380530747));
#46896=CARTESIAN_POINT('Ctrl Pts',(0.173946627589401,-1.,-1.84898113200543));
#46897=CARTESIAN_POINT('Ctrl Pts',(0.173946627589401,1.,-1.84898113200543));
#46898=CARTESIAN_POINT('Ctrl Pts',(0.174735259276856,-1.,-1.85948367089838));
#46899=CARTESIAN_POINT('Ctrl Pts',(0.174735259276856,1.,-1.85948367089838));
#46900=CARTESIAN_POINT('Ctrl Pts',(0.175268337590901,-1.,-1.86828349694972));
#46901=CARTESIAN_POINT('Ctrl Pts',(0.175268337590901,1.,-1.86828349694972));
#46902=CARTESIAN_POINT('Ctrl Pts',(0.175563480746205,-1.,-1.87563767773249));
#46903=CARTESIAN_POINT('Ctrl Pts',(0.175563480746205,1.,-1.87563767773249));
#46904=CARTESIAN_POINT('Ctrl Pts',(0.175644148889271,-1.,-1.88188663144846));
#46905=CARTESIAN_POINT('Ctrl Pts',(0.175644148889271,1.,-1.88188663144846));
#46906=CARTESIAN_POINT('Ctrl Pts',(0.175538155840286,-1.,-1.88742606272818));
#46907=CARTESIAN_POINT('Ctrl Pts',(0.175538155840286,1.,-1.88742606272818));
#46908=CARTESIAN_POINT('Ctrl Pts',(0.175274276190664,-1.,-1.89264630198279));
#46909=CARTESIAN_POINT('Ctrl Pts',(0.175274276190664,1.,-1.89264630198279));
#46910=CARTESIAN_POINT('Ctrl Pts',(0.174879405091277,-1.,-1.89788101117148));
#46911=CARTESIAN_POINT('Ctrl Pts',(0.174879405091277,1.,-1.89788101117148));
#46912=CARTESIAN_POINT('Ctrl Pts',(0.174375518661222,-1.,-1.90335253863003));
#46913=CARTESIAN_POINT('Ctrl Pts',(0.174375518661222,1.,-1.90335253863003));
#46914=CARTESIAN_POINT('Ctrl Pts',(0.173776635257984,-1.,-1.90911693975475));
#46915=CARTESIAN_POINT('Ctrl Pts',(0.173776635257984,1.,-1.90911693975475));
#46916=CARTESIAN_POINT('Ctrl Pts',(0.173090695383619,-1.,-1.91511429159681));
#46917=CARTESIAN_POINT('Ctrl Pts',(0.173090695383619,1.,-1.91511429159681));
#46918=CARTESIAN_POINT('Ctrl Pts',(0.172321621259557,-1.,-1.92122334398034));
#46919=CARTESIAN_POINT('Ctrl Pts',(0.172321621259557,1.,-1.92122334398034));
#46920=CARTESIAN_POINT('Ctrl Pts',(0.17147119153296,-1.,-1.92731093582));
#46921=CARTESIAN_POINT('Ctrl Pts',(0.17147119153296,1.,-1.92731093582));
#46922=CARTESIAN_POINT('Ctrl Pts',(0.170541253116136,-1.,-1.93329183155455));
#46923=CARTESIAN_POINT('Ctrl Pts',(0.170541253116136,1.,-1.93329183155455));
#46924=CARTESIAN_POINT('Ctrl Pts',(0.169534904817425,-1.,-1.93915639211497));
#46925=CARTESIAN_POINT('Ctrl Pts',(0.169534904817425,1.,-1.93915639211497));
#46926=CARTESIAN_POINT('Ctrl Pts',(0.168455741607516,-1.,-1.94493757756879));
#46927=CARTESIAN_POINT('Ctrl Pts',(0.168455741607516,1.,-1.94493757756879));
#46928=CARTESIAN_POINT('Ctrl Pts',(0.167307501784469,-1.,-1.95069027794286));
#46929=CARTESIAN_POINT('Ctrl Pts',(0.167307501784469,1.,-1.95069027794286));
#46930=CARTESIAN_POINT('Ctrl Pts',(0.166093592002833,-1.,-1.95646759718755));
#46931=CARTESIAN_POINT('Ctrl Pts',(0.166093592002833,1.,-1.95646759718755));
#46932=CARTESIAN_POINT('Ctrl Pts',(0.1648165689203,-1.,-1.96229379940174));
#46933=CARTESIAN_POINT('Ctrl Pts',(0.1648165689203,1.,-1.96229379940174));
#46934=CARTESIAN_POINT('Ctrl Pts',(0.16347818545776,-1.,-1.96816512678));
#46935=CARTESIAN_POINT('Ctrl Pts',(0.16347818545776,1.,-1.96816512678));
#46936=CARTESIAN_POINT('Ctrl Pts',(0.162079693556302,-1.,-1.97406280235204));
#46937=CARTESIAN_POINT('Ctrl Pts',(0.162079693556302,1.,-1.97406280235204));
#46938=CARTESIAN_POINT('Ctrl Pts',(0.16062206078461,-1.,-1.97996195437557));
#46939=CARTESIAN_POINT('Ctrl Pts',(0.16062206078461,1.,-1.97996195437557));
#46940=CARTESIAN_POINT('Ctrl Pts',(0.159106226437288,-1.,-1.98584238283279));
#46941=CARTESIAN_POINT('Ctrl Pts',(0.159106226437288,1.,-1.98584238283279));
#46942=CARTESIAN_POINT('Ctrl Pts',(0.157533331459215,-1.,-1.99169810931893));
#46943=CARTESIAN_POINT('Ctrl Pts',(0.157533331459215,1.,-1.99169810931893));
#46944=CARTESIAN_POINT('Ctrl Pts',(0.155904629548774,-1.,-1.99753284771487));
#46945=CARTESIAN_POINT('Ctrl Pts',(0.155904629548774,1.,-1.99753284771487));
#46946=CARTESIAN_POINT('Ctrl Pts',(0.154221403049719,-1.,-2.00335565310539));
#46947=CARTESIAN_POINT('Ctrl Pts',(0.154221403049719,1.,-2.00335565310539));
#46948=CARTESIAN_POINT('Ctrl Pts',(0.152484883621452,-1.,-2.00917680318426));
#46949=CARTESIAN_POINT('Ctrl Pts',(0.152484883621452,1.,-2.00917680318426));
#46950=CARTESIAN_POINT('Ctrl Pts',(0.150696157673084,-1.,-2.01500291940243));
#46951=CARTESIAN_POINT('Ctrl Pts',(0.150696157673084,1.,-2.01500291940243));
#46952=CARTESIAN_POINT('Ctrl Pts',(0.148856124775343,-1.,-2.02083464969897));
#46953=CARTESIAN_POINT('Ctrl Pts',(0.148856124775343,1.,-2.02083464969897));
#46954=CARTESIAN_POINT('Ctrl Pts',(0.146965557332586,-1.,-2.02666926182017));
#46955=CARTESIAN_POINT('Ctrl Pts',(0.146965557332586,1.,-2.02666926182017));
#46956=CARTESIAN_POINT('Ctrl Pts',(0.145025140186058,-1.,-2.03250223739941));
#46957=CARTESIAN_POINT('Ctrl Pts',(0.145025140186058,1.,-2.03250223739941));
#46958=CARTESIAN_POINT('Ctrl Pts',(0.143035515058208,-1.,-2.03832911025913));
#46959=CARTESIAN_POINT('Ctrl Pts',(0.143035515058208,1.,-2.03832911025913));
#46960=CARTESIAN_POINT('Ctrl Pts',(0.140997332152545,-1.,-2.04414757947919));
#46961=CARTESIAN_POINT('Ctrl Pts',(0.140997332152545,1.,-2.04414757947919));
#46962=CARTESIAN_POINT('Ctrl Pts',(0.138911255368966,-1.,-2.04995762001333));
#46963=CARTESIAN_POINT('Ctrl Pts',(0.138911255368966,1.,-2.04995762001333));
#46964=CARTESIAN_POINT('Ctrl Pts',(0.136777941218044,-1.,-2.0557604441427));
#46965=CARTESIAN_POINT('Ctrl Pts',(0.136777941218044,1.,-2.0557604441427));
#46966=CARTESIAN_POINT('Ctrl Pts',(0.134598026192107,-1.,-2.06155781517844));
#46967=CARTESIAN_POINT('Ctrl Pts',(0.134598026192107,1.,-2.06155781517844));
#46968=CARTESIAN_POINT('Ctrl Pts',(0.13237211154771,-1.,-2.06735123910319));
#46969=CARTESIAN_POINT('Ctrl Pts',(0.13237211154771,1.,-2.06735123910319));
#46970=CARTESIAN_POINT('Ctrl Pts',(0.1301007483284,-1.,-2.07314114713047));
#46971=CARTESIAN_POINT('Ctrl Pts',(0.1301007483284,1.,-2.07314114713047));
#46972=CARTESIAN_POINT('Ctrl Pts',(0.127784445276116,-1.,-2.07892715110967));
#46973=CARTESIAN_POINT('Ctrl Pts',(0.127784445276116,1.,-2.07892715110967));
#46974=CARTESIAN_POINT('Ctrl Pts',(0.125423679412058,-1.,-2.08470840653628));
#46975=CARTESIAN_POINT('Ctrl Pts',(0.125423679412058,1.,-2.08470840653628));
#46976=CARTESIAN_POINT('Ctrl Pts',(0.123018905621083,-1.,-2.09048392424826));
#46977=CARTESIAN_POINT('Ctrl Pts',(0.123018905621083,1.,-2.09048392424826));
#46978=CARTESIAN_POINT('Ctrl Pts',(0.120570567965129,-1.,-2.09625292867756));
#46979=CARTESIAN_POINT('Ctrl Pts',(0.120570567965129,1.,-2.09625292867756));
#46980=CARTESIAN_POINT('Ctrl Pts',(0.118079107988368,-1.,-2.10201512132945));
#46981=CARTESIAN_POINT('Ctrl Pts',(0.118079107988368,1.,-2.10201512132945));
#46982=CARTESIAN_POINT('Ctrl Pts',(0.11554495768794,-1.,-2.10777050261359));
#46983=CARTESIAN_POINT('Ctrl Pts',(0.11554495768794,1.,-2.10777050261359));
#46984=CARTESIAN_POINT('Ctrl Pts',(0.112968534419746,-1.,-2.11351924490335));
#46985=CARTESIAN_POINT('Ctrl Pts',(0.112968534419746,1.,-2.11351924490335));
#46986=CARTESIAN_POINT('Ctrl Pts',(0.11035023613502,-1.,-2.11926155590849));
#46987=CARTESIAN_POINT('Ctrl Pts',(0.11035023613502,1.,-2.11926155590849));
#46988=CARTESIAN_POINT('Ctrl Pts',(0.107690435231068,-1.,-2.12499752306927));
#46989=CARTESIAN_POINT('Ctrl Pts',(0.107690435231068,1.,-2.12499752306927));
#46990=CARTESIAN_POINT('Ctrl Pts',(0.104989479152703,-1.,-2.1307270488718));
#46991=CARTESIAN_POINT('Ctrl Pts',(0.104989479152703,1.,-2.1307270488718));
#46992=CARTESIAN_POINT('Ctrl Pts',(0.102247700556064,-1.,-2.13644992667052));
#46993=CARTESIAN_POINT('Ctrl Pts',(0.102247700556064,1.,-2.13644992667052));
#46994=CARTESIAN_POINT('Ctrl Pts',(0.0994654261990743,-1.,-2.14216588395974));
#46995=CARTESIAN_POINT('Ctrl Pts',(0.0994654261990743,1.,-2.14216588395974));
#46996=CARTESIAN_POINT('Ctrl Pts',(0.0966429852305689,-1.,-2.14787463531864));
#46997=CARTESIAN_POINT('Ctrl Pts',(0.0966429852305689,1.,-2.14787463531864));
#46998=CARTESIAN_POINT('Ctrl Pts',(0.0937807218868345,-1.,-2.15357593978377));
#46999=CARTESIAN_POINT('Ctrl Pts',(0.0937807218868345,1.,-2.15357593978377));
#47000=CARTESIAN_POINT('Ctrl Pts',(0.0908789888108266,-1.,-2.15926961544808));
#47001=CARTESIAN_POINT('Ctrl Pts',(0.0908789888108266,1.,-2.15926961544808));
#47002=CARTESIAN_POINT('Ctrl Pts',(0.0879381291387823,-1.,-2.16495552645275));
#47003=CARTESIAN_POINT('Ctrl Pts',(0.0879381291387823,1.,-2.16495552645275));
#47004=CARTESIAN_POINT('Ctrl Pts',(0.0849584620835643,-1.,-2.17063357871031));
#47005=CARTESIAN_POINT('Ctrl Pts',(0.0849584620835643,1.,-2.17063357871031));
#47006=CARTESIAN_POINT('Ctrl Pts',(0.0819402680871939,-1.,-2.1763037121106));
#47007=CARTESIAN_POINT('Ctrl Pts',(0.0819402680871939,1.,-2.1763037121106));
#47008=CARTESIAN_POINT('Ctrl Pts',(0.0788837727683228,-1.,-2.18196589448304));
#47009=CARTESIAN_POINT('Ctrl Pts',(0.0788837727683228,1.,-2.18196589448304));
#47010=CARTESIAN_POINT('Ctrl Pts',(0.0757891465833411,-1.,-2.1876201139874));
#47011=CARTESIAN_POINT('Ctrl Pts',(0.0757891465833411,1.,-2.1876201139874));
#47012=CARTESIAN_POINT('Ctrl Pts',(0.0732830357304276,-1.,-2.19213712012956));
#47013=CARTESIAN_POINT('Ctrl Pts',(0.0732830357304276,1.,-2.19213712012956));
#47014=CARTESIAN_POINT('Ctrl Pts',(0.0713863779524627,-1.,-2.19552129483562));
#47015=CARTESIAN_POINT('Ctrl Pts',(0.0713863779524627,1.,-2.19552129483562));
#47016=CARTESIAN_POINT('Ctrl Pts',(0.0701143536324926,-1.,-2.19777582085261));
#47017=CARTESIAN_POINT('Ctrl Pts',(0.0701143536324926,1.,-2.19777582085261));
#47018=CARTESIAN_POINT('Ctrl Pts',(0.0694764450219584,-1.,-2.19890268624765));
#47019=CARTESIAN_POINT('Ctrl Pts',(0.0694764450219584,1.,-2.19890268624765));
#47020=CARTESIAN_POINT('',(0.163289472382896,1.,-1.74236521665491));
#47021=CARTESIAN_POINT('Ctrl Pts',(0.163289472382896,1.,-1.74236521665491));
#47022=CARTESIAN_POINT('Ctrl Pts',(0.163814161002474,1.,-1.74720349503904));
#47023=CARTESIAN_POINT('Ctrl Pts',(0.164834765708484,1.,-1.75666056640041));
#47024=CARTESIAN_POINT('Ctrl Pts',(0.166279355148738,1.,-1.77018771687692));
#47025=CARTESIAN_POINT('Ctrl Pts',(0.16803277280837,1.,-1.78690649988931));
#47026=CARTESIAN_POINT('Ctrl Pts',(0.169936923908078,1.,-1.80561530633924));
#47027=CARTESIAN_POINT('Ctrl Pts',(0.171554770207306,1.,-1.82215766815414));
#47028=CARTESIAN_POINT('Ctrl Pts',(0.17288944289442,1.,-1.83658380530747));
#47029=CARTESIAN_POINT('Ctrl Pts',(0.173946627589401,1.,-1.84898113200543));
#47030=CARTESIAN_POINT('Ctrl Pts',(0.174735259276856,1.,-1.85948367089838));
#47031=CARTESIAN_POINT('Ctrl Pts',(0.175268337590901,1.,-1.86828349694972));
#47032=CARTESIAN_POINT('Ctrl Pts',(0.175563480746205,1.,-1.87563767773249));
#47033=CARTESIAN_POINT('Ctrl Pts',(0.175644148889271,1.,-1.88188663144846));
#47034=CARTESIAN_POINT('Ctrl Pts',(0.175538155840286,1.,-1.88742606272818));
#47035=CARTESIAN_POINT('Ctrl Pts',(0.175274276190664,1.,-1.89264630198279));
#47036=CARTESIAN_POINT('Ctrl Pts',(0.174879405091277,1.,-1.89788101117148));
#47037=CARTESIAN_POINT('Ctrl Pts',(0.174375518661222,1.,-1.90335253863003));
#47038=CARTESIAN_POINT('Ctrl Pts',(0.173776635257984,1.,-1.90911693975475));
#47039=CARTESIAN_POINT('Ctrl Pts',(0.173090695383619,1.,-1.91511429159681));
#47040=CARTESIAN_POINT('Ctrl Pts',(0.172321621259557,1.,-1.92122334398034));
#47041=CARTESIAN_POINT('Ctrl Pts',(0.17147119153296,1.,-1.92731093582));
#47042=CARTESIAN_POINT('Ctrl Pts',(0.170541253116136,1.,-1.93329183155455));
#47043=CARTESIAN_POINT('Ctrl Pts',(0.169534904817425,1.,-1.93915639211497));
#47044=CARTESIAN_POINT('Ctrl Pts',(0.168455741607516,1.,-1.94493757756879));
#47045=CARTESIAN_POINT('Ctrl Pts',(0.167307501784469,1.,-1.95069027794286));
#47046=CARTESIAN_POINT('Ctrl Pts',(0.166093592002833,1.,-1.95646759718755));
#47047=CARTESIAN_POINT('Ctrl Pts',(0.1648165689203,1.,-1.96229379940174));
#47048=CARTESIAN_POINT('Ctrl Pts',(0.16347818545776,1.,-1.96816512678));
#47049=CARTESIAN_POINT('Ctrl Pts',(0.162079693556302,1.,-1.97406280235204));
#47050=CARTESIAN_POINT('Ctrl Pts',(0.16062206078461,1.,-1.97996195437557));
#47051=CARTESIAN_POINT('Ctrl Pts',(0.159106226437288,1.,-1.98584238283279));
#47052=CARTESIAN_POINT('Ctrl Pts',(0.157533331459215,1.,-1.99169810931893));
#47053=CARTESIAN_POINT('Ctrl Pts',(0.155904629548774,1.,-1.99753284771487));
#47054=CARTESIAN_POINT('Ctrl Pts',(0.154221403049719,1.,-2.00335565310539));
#47055=CARTESIAN_POINT('Ctrl Pts',(0.152484883621452,1.,-2.00917680318426));
#47056=CARTESIAN_POINT('Ctrl Pts',(0.150696157673084,1.,-2.01500291940243));
#47057=CARTESIAN_POINT('Ctrl Pts',(0.148856124775343,1.,-2.02083464969897));
#47058=CARTESIAN_POINT('Ctrl Pts',(0.146965557332586,1.,-2.02666926182017));
#47059=CARTESIAN_POINT('Ctrl Pts',(0.145025140186058,1.,-2.03250223739941));
#47060=CARTESIAN_POINT('Ctrl Pts',(0.143035515058208,1.,-2.03832911025913));
#47061=CARTESIAN_POINT('Ctrl Pts',(0.140997332152545,1.,-2.04414757947919));
#47062=CARTESIAN_POINT('Ctrl Pts',(0.138911255368966,1.,-2.04995762001333));
#47063=CARTESIAN_POINT('Ctrl Pts',(0.136777941218044,1.,-2.0557604441427));
#47064=CARTESIAN_POINT('Ctrl Pts',(0.134598026192107,1.,-2.06155781517844));
#47065=CARTESIAN_POINT('Ctrl Pts',(0.13237211154771,1.,-2.06735123910319));
#47066=CARTESIAN_POINT('Ctrl Pts',(0.1301007483284,1.,-2.07314114713047));
#47067=CARTESIAN_POINT('Ctrl Pts',(0.127784445276116,1.,-2.07892715110967));
#47068=CARTESIAN_POINT('Ctrl Pts',(0.125423679412058,1.,-2.08470840653628));
#47069=CARTESIAN_POINT('Ctrl Pts',(0.123018905621083,1.,-2.09048392424826));
#47070=CARTESIAN_POINT('Ctrl Pts',(0.120570567965129,1.,-2.09625292867756));
#47071=CARTESIAN_POINT('Ctrl Pts',(0.118079107988368,1.,-2.10201512132945));
#47072=CARTESIAN_POINT('Ctrl Pts',(0.11554495768794,1.,-2.10777050261359));
#47073=CARTESIAN_POINT('Ctrl Pts',(0.112968534419746,1.,-2.11351924490335));
#47074=CARTESIAN_POINT('Ctrl Pts',(0.11035023613502,1.,-2.11926155590849));
#47075=CARTESIAN_POINT('Ctrl Pts',(0.107690435231068,1.,-2.12499752306927));
#47076=CARTESIAN_POINT('Ctrl Pts',(0.104989479152703,1.,-2.1307270488718));
#47077=CARTESIAN_POINT('Ctrl Pts',(0.102247700556064,1.,-2.13644992667052));
#47078=CARTESIAN_POINT('Ctrl Pts',(0.0994654261990743,1.,-2.14216588395974));
#47079=CARTESIAN_POINT('Ctrl Pts',(0.0966429852305689,1.,-2.14787463531864));
#47080=CARTESIAN_POINT('Ctrl Pts',(0.0937807218868345,1.,-2.15357593978377));
#47081=CARTESIAN_POINT('Ctrl Pts',(0.0908789888108266,1.,-2.15926961544808));
#47082=CARTESIAN_POINT('Ctrl Pts',(0.0879381291387823,1.,-2.16495552645275));
#47083=CARTESIAN_POINT('Ctrl Pts',(0.0849584620835643,1.,-2.17063357871031));
#47084=CARTESIAN_POINT('Ctrl Pts',(0.0819402680871939,1.,-2.1763037121106));
#47085=CARTESIAN_POINT('Ctrl Pts',(0.0788837727683228,1.,-2.18196589448304));
#47086=CARTESIAN_POINT('Ctrl Pts',(0.0757891465833411,1.,-2.1876201139874));
#47087=CARTESIAN_POINT('Ctrl Pts',(0.0732830357304276,1.,-2.19213712012956));
#47088=CARTESIAN_POINT('Ctrl Pts',(0.0713863779524627,1.,-2.19552129483562));
#47089=CARTESIAN_POINT('Ctrl Pts',(0.0701143536324926,1.,-2.19777582085261));
#47090=CARTESIAN_POINT('Ctrl Pts',(0.0694764450219584,1.,-2.19890268624765));
#47091=CARTESIAN_POINT('',(0.163289472382896,0.,-1.74236521665491));
#47092=CARTESIAN_POINT('Origin',(0.,0.,0.));
#47093=CARTESIAN_POINT('',(0.383122945602004,1.,-1.7075470150345));
#47094=CARTESIAN_POINT('Origin',(0.,1.,0.));
#47095=CARTESIAN_POINT('',(0.383122945602004,0.,-1.7075470150345));
#47096=CARTESIAN_POINT('Ctrl Pts',(0.61342227326009,-1.,-2.11275013067528));
#47097=CARTESIAN_POINT('Ctrl Pts',(0.61342227326009,1.,-2.11275013067528));
#47098=CARTESIAN_POINT('Ctrl Pts',(0.61246736556225,-1.,-2.11187554260142));
#47099=CARTESIAN_POINT('Ctrl Pts',(0.61246736556225,1.,-2.11187554260142));
#47100=CARTESIAN_POINT('Ctrl Pts',(0.610560911691113,-1.,-2.11012443807661));
#47101=CARTESIAN_POINT('Ctrl Pts',(0.610560911691113,1.,-2.11012443807661));
#47102=CARTESIAN_POINT('Ctrl Pts',(0.607711315456826,-1.,-2.10749199615859));
#47103=CARTESIAN_POINT('Ctrl Pts',(0.607711315456826,1.,-2.10749199615859));
#47104=CARTESIAN_POINT('Ctrl Pts',(0.603932030738212,-1.,-2.10397049887709));
#47105=CARTESIAN_POINT('Ctrl Pts',(0.603932030738212,1.,-2.10397049887709));
#47106=CARTESIAN_POINT('Ctrl Pts',(0.599241616422144,-1.,-2.09954930865331));
#47107=CARTESIAN_POINT('Ctrl Pts',(0.599241616422144,1.,-2.09954930865331));
#47108=CARTESIAN_POINT('Ctrl Pts',(0.594585006052823,-1.,-2.09510876220501));
#47109=CARTESIAN_POINT('Ctrl Pts',(0.594585006052823,1.,-2.09510876220501));
#47110=CARTESIAN_POINT('Ctrl Pts',(0.589962365403189,-1.,-2.09064881812053));
#47111=CARTESIAN_POINT('Ctrl Pts',(0.589962365403189,1.,-2.09064881812053));
#47112=CARTESIAN_POINT('Ctrl Pts',(0.585373918990895,-1.,-2.086169437277));
#47113=CARTESIAN_POINT('Ctrl Pts',(0.585373918990895,1.,-2.086169437277));
#47114=CARTESIAN_POINT('Ctrl Pts',(0.580819952107256,-1.,-2.08167059018138));
#47115=CARTESIAN_POINT('Ctrl Pts',(0.580819952107256,1.,-2.08167059018138));
#47116=CARTESIAN_POINT('Ctrl Pts',(0.576300797416274,-1.,-2.07715226767361));
#47117=CARTESIAN_POINT('Ctrl Pts',(0.576300797416274,1.,-2.07715226767361));
#47118=CARTESIAN_POINT('Ctrl Pts',(0.571816823242411,-1.,-2.07261449292758));
#47119=CARTESIAN_POINT('Ctrl Pts',(0.571816823242411,1.,-2.07261449292758));
#47120=CARTESIAN_POINT('Ctrl Pts',(0.567368421181229,-1.,-2.06805732997383));
#47121=CARTESIAN_POINT('Ctrl Pts',(0.567368421181229,1.,-2.06805732997383));
#47122=CARTESIAN_POINT('Ctrl Pts',(0.562955993082574,-1.,-2.06348090160697));
#47123=CARTESIAN_POINT('Ctrl Pts',(0.562955993082574,1.,-2.06348090160697));
#47124=CARTESIAN_POINT('Ctrl Pts',(0.558579940185467,-1.,-2.05888537756571));
#47125=CARTESIAN_POINT('Ctrl Pts',(0.558579940185467,1.,-2.05888537756571));
#47126=CARTESIAN_POINT('Ctrl Pts',(0.554240657464109,-1.,-2.05427091604482));
#47127=CARTESIAN_POINT('Ctrl Pts',(0.554240657464109,1.,-2.05427091604482));
#47128=CARTESIAN_POINT('Ctrl Pts',(0.549938525150342,-1.,-2.04963761077974));
#47129=CARTESIAN_POINT('Ctrl Pts',(0.549938525150342,1.,-2.04963761077974));
#47130=CARTESIAN_POINT('Ctrl Pts',(0.545673903817348,-1.,-2.0449854471456));
#47131=CARTESIAN_POINT('Ctrl Pts',(0.545673903817348,1.,-2.0449854471456));
#47132=CARTESIAN_POINT('Ctrl Pts',(0.54144712061552,-1.,-2.0403142269048));
#47133=CARTESIAN_POINT('Ctrl Pts',(0.54144712061552,1.,-2.0403142269048));
#47134=CARTESIAN_POINT('Ctrl Pts',(0.537258489833134,-1.,-2.03562362953993));
#47135=CARTESIAN_POINT('Ctrl Pts',(0.537258489833134,1.,-2.03562362953993));
#47136=CARTESIAN_POINT('Ctrl Pts',(0.533108355132905,-1.,-2.03091336214401));
#47137=CARTESIAN_POINT('Ctrl Pts',(0.533108355132905,1.,-2.03091336214401));
#47138=CARTESIAN_POINT('Ctrl Pts',(0.52899712724191,-1.,-2.02618329083289));
#47139=CARTESIAN_POINT('Ctrl Pts',(0.52899712724191,1.,-2.02618329083289));
#47140=CARTESIAN_POINT('Ctrl Pts',(0.524925318333518,-1.,-2.02143356304712));
#47141=CARTESIAN_POINT('Ctrl Pts',(0.524925318333518,1.,-2.02143356304712));
#47142=CARTESIAN_POINT('Ctrl Pts',(0.520893590399428,-1.,-2.01666477917306));
#47143=CARTESIAN_POINT('Ctrl Pts',(0.520893590399428,1.,-2.01666477917306));
#47144=CARTESIAN_POINT('Ctrl Pts',(0.516902681728733,-1.,-2.01187773939257));
#47145=CARTESIAN_POINT('Ctrl Pts',(0.516902681728733,1.,-2.01187773939257));
#47146=CARTESIAN_POINT('Ctrl Pts',(0.512953306961813,-1.,-2.00707309946955));
#47147=CARTESIAN_POINT('Ctrl Pts',(0.512953306961813,1.,-2.00707309946955));
#47148=CARTESIAN_POINT('Ctrl Pts',(0.509046069886152,-1.,-2.00225107134733));
#47149=CARTESIAN_POINT('Ctrl Pts',(0.509046069886152,1.,-2.00225107134733));
#47150=CARTESIAN_POINT('Ctrl Pts',(0.505181361323011,-1.,-1.99741107463567));
#47151=CARTESIAN_POINT('Ctrl Pts',(0.505181361323011,1.,-1.99741107463567));
#47152=CARTESIAN_POINT('Ctrl Pts',(0.501359287727129,-1.,-1.9925514912615));
#47153=CARTESIAN_POINT('Ctrl Pts',(0.501359287727129,1.,-1.9925514912615));
#47154=CARTESIAN_POINT('Ctrl Pts',(0.497579909545564,-1.,-1.98767044752929));
#47155=CARTESIAN_POINT('Ctrl Pts',(0.497579909545564,1.,-1.98767044752929));
#47156=CARTESIAN_POINT('Ctrl Pts',(0.493843476541492,-1.,-1.9827665876182));
#47157=CARTESIAN_POINT('Ctrl Pts',(0.493843476541492,1.,-1.9827665876182));
#47158=CARTESIAN_POINT('Ctrl Pts',(0.490150627860955,-1.,-1.97783973019229));
#47159=CARTESIAN_POINT('Ctrl Pts',(0.490150627860955,1.,-1.97783973019229));
#47160=CARTESIAN_POINT('Ctrl Pts',(0.486502692907661,-1.,-1.97289186263272));
#47161=CARTESIAN_POINT('Ctrl Pts',(0.486502692907661,1.,-1.97289186263272));
#47162=CARTESIAN_POINT('Ctrl Pts',(0.482901662120686,-1.,-1.96792703422358));
#47163=CARTESIAN_POINT('Ctrl Pts',(0.482901662120686,1.,-1.96792703422358));
#47164=CARTESIAN_POINT('Ctrl Pts',(0.479349583074846,-1.,-1.96294933055938));
#47165=CARTESIAN_POINT('Ctrl Pts',(0.479349583074846,1.,-1.96294933055938));
#47166=CARTESIAN_POINT('Ctrl Pts',(0.475848034683171,-1.,-1.95796111148175));
#47167=CARTESIAN_POINT('Ctrl Pts',(0.475848034683171,1.,-1.95796111148175));
#47168=CARTESIAN_POINT('Ctrl Pts',(0.472397672264079,-1.,-1.95296148278136));
#47169=CARTESIAN_POINT('Ctrl Pts',(0.472397672264079,1.,-1.95296148278136));
#47170=CARTESIAN_POINT('Ctrl Pts',(0.468997482913158,-1.,-1.94794381136524));
#47171=CARTESIAN_POINT('Ctrl Pts',(0.468997482913158,1.,-1.94794381136524));
#47172=CARTESIAN_POINT('Ctrl Pts',(0.465645462026064,-1.,-1.94289794196205));
#47173=CARTESIAN_POINT('Ctrl Pts',(0.465645462026064,1.,-1.94289794196205));
#47174=CARTESIAN_POINT('Ctrl Pts',(0.462340031009087,-1.,-1.93781486640834));
#47175=CARTESIAN_POINT('Ctrl Pts',(0.462340031009087,1.,-1.93781486640834));
#47176=CARTESIAN_POINT('Ctrl Pts',(0.459081234547931,-1.,-1.93269066517936));
#47177=CARTESIAN_POINT('Ctrl Pts',(0.459081234547931,1.,-1.93269066517936));
#47178=CARTESIAN_POINT('Ctrl Pts',(0.455872005174335,-1.,-1.92753067150461));
#47179=CARTESIAN_POINT('Ctrl Pts',(0.455872005174335,1.,-1.92753067150461));
#47180=CARTESIAN_POINT('Ctrl Pts',(0.452719478359356,-1.,-1.9223538064847));
#47181=CARTESIAN_POINT('Ctrl Pts',(0.452719478359356,1.,-1.9223538064847));
#47182=CARTESIAN_POINT('Ctrl Pts',(0.449632260106572,-1.,-1.91718342555717));
#47183=CARTESIAN_POINT('Ctrl Pts',(0.449632260106572,1.,-1.91718342555717));
#47184=CARTESIAN_POINT('Ctrl Pts',(0.446617343485651,-1.,-1.91203699981095));
#47185=CARTESIAN_POINT('Ctrl Pts',(0.446617343485651,1.,-1.91203699981095));
#47186=CARTESIAN_POINT('Ctrl Pts',(0.44367755684917,-1.,-1.90691756144906));
#47187=CARTESIAN_POINT('Ctrl Pts',(0.44367755684917,1.,-1.90691756144906));
#47188=CARTESIAN_POINT('Ctrl Pts',(0.44080783370416,-1.,-1.90180124389137));
#47189=CARTESIAN_POINT('Ctrl Pts',(0.44080783370416,1.,-1.90180124389137));
#47190=CARTESIAN_POINT('Ctrl Pts',(0.437995003948443,-1.,-1.89663648956549));
#47191=CARTESIAN_POINT('Ctrl Pts',(0.437995003948443,1.,-1.89663648956549));
#47192=CARTESIAN_POINT('Ctrl Pts',(0.43522566096358,-1.,-1.89136993975585));
#47193=CARTESIAN_POINT('Ctrl Pts',(0.43522566096358,1.,-1.89136993975585));
#47194=CARTESIAN_POINT('Ctrl Pts',(0.432493038548833,-1.,-1.88596913666828));
#47195=CARTESIAN_POINT('Ctrl Pts',(0.432493038548833,1.,-1.88596913666828));
#47196=CARTESIAN_POINT('Ctrl Pts',(0.429803062482217,-1.,-1.88044229001779));
#47197=CARTESIAN_POINT('Ctrl Pts',(0.429803062482217,1.,-1.88044229001779));
#47198=CARTESIAN_POINT('Ctrl Pts',(0.427183828518743,-1.,-1.87486989291334));
#47199=CARTESIAN_POINT('Ctrl Pts',(0.427183828518743,1.,-1.87486989291334));
#47200=CARTESIAN_POINT('Ctrl Pts',(0.424678177290876,-1.,-1.8693780394412));
#47201=CARTESIAN_POINT('Ctrl Pts',(0.424678177290876,1.,-1.8693780394412));
#47202=CARTESIAN_POINT('Ctrl Pts',(0.422327307417884,-1.,-1.86408083333863));
#47203=CARTESIAN_POINT('Ctrl Pts',(0.422327307417884,1.,-1.86408083333863));
#47204=CARTESIAN_POINT('Ctrl Pts',(0.420157287975583,-1.,-1.8590328109667));
#47205=CARTESIAN_POINT('Ctrl Pts',(0.420157287975583,1.,-1.8590328109667));
#47206=CARTESIAN_POINT('Ctrl Pts',(0.418164129144045,-1.,-1.8541763285645));
#47207=CARTESIAN_POINT('Ctrl Pts',(0.418164129144045,1.,-1.8541763285645));
#47208=CARTESIAN_POINT('Ctrl Pts',(0.416300022039885,-1.,-1.84929312930314));
#47209=CARTESIAN_POINT('Ctrl Pts',(0.416300022039885,1.,-1.84929312930314));
#47210=CARTESIAN_POINT('Ctrl Pts',(0.414487438255542,-1.,-1.84405757074218));
#47211=CARTESIAN_POINT('Ctrl Pts',(0.414487438255542,1.,-1.84405757074218));
#47212=CARTESIAN_POINT('Ctrl Pts',(0.412633125322945,-1.,-1.8380895347617));
#47213=CARTESIAN_POINT('Ctrl Pts',(0.412633125322945,1.,-1.8380895347617));
#47214=CARTESIAN_POINT('Ctrl Pts',(0.410641256301276,-1.,-1.83100408895047));
#47215=CARTESIAN_POINT('Ctrl Pts',(0.410641256301276,1.,-1.83100408895047));
#47216=CARTESIAN_POINT('Ctrl Pts',(0.408428948106227,-1.,-1.82247022677562));
#47217=CARTESIAN_POINT('Ctrl Pts',(0.408428948106227,1.,-1.82247022677562));
#47218=CARTESIAN_POINT('Ctrl Pts',(0.405933518407175,-1.,-1.81223801812013));
#47219=CARTESIAN_POINT('Ctrl Pts',(0.405933518407175,1.,-1.81223801812013));
#47220=CARTESIAN_POINT('Ctrl Pts',(0.403107976163396,-1.,-1.80012077173238));
#47221=CARTESIAN_POINT('Ctrl Pts',(0.403107976163396,1.,-1.80012077173238));
#47222=CARTESIAN_POINT('Ctrl Pts',(0.399919403774155,-1.,-1.78598826343754));
#47223=CARTESIAN_POINT('Ctrl Pts',(0.399919403774155,1.,-1.78598826343754));
#47224=CARTESIAN_POINT('Ctrl Pts',(0.396346196110688,-1.,-1.76975560043442));
#47225=CARTESIAN_POINT('Ctrl Pts',(0.396346196110688,1.,-1.76975560043442));
#47226=CARTESIAN_POINT('Ctrl Pts',(0.392375812285395,-1.,-1.75137405310193));
#47227=CARTESIAN_POINT('Ctrl Pts',(0.392375812285395,1.,-1.75137405310193));
#47228=CARTESIAN_POINT('Ctrl Pts',(0.388877023502615,-1.,-1.73493170972829));
#47229=CARTESIAN_POINT('Ctrl Pts',(0.388877023502615,1.,-1.73493170972829));
#47230=CARTESIAN_POINT('Ctrl Pts',(0.386070790323281,-1.,-1.72162022244582));
#47231=CARTESIAN_POINT('Ctrl Pts',(0.386070790323281,1.,-1.72162022244582));
#47232=CARTESIAN_POINT('Ctrl Pts',(0.384119047314215,-1.,-1.71231062891398));
#47233=CARTESIAN_POINT('Ctrl Pts',(0.384119047314215,1.,-1.71231062891398));
#47234=CARTESIAN_POINT('Ctrl Pts',(0.383122945602004,-1.,-1.7075470150345));
#47235=CARTESIAN_POINT('Ctrl Pts',(0.383122945602004,1.,-1.7075470150345));
#47236=CARTESIAN_POINT('',(0.61342227326009,1.,-2.11275013067528));
#47237=CARTESIAN_POINT('Ctrl Pts',(0.61342227326009,1.,-2.11275013067528));
#47238=CARTESIAN_POINT('Ctrl Pts',(0.61246736556225,1.,-2.11187554260142));
#47239=CARTESIAN_POINT('Ctrl Pts',(0.610560911691113,1.,-2.11012443807661));
#47240=CARTESIAN_POINT('Ctrl Pts',(0.607711315456826,1.,-2.10749199615859));
#47241=CARTESIAN_POINT('Ctrl Pts',(0.603932030738212,1.,-2.10397049887709));
#47242=CARTESIAN_POINT('Ctrl Pts',(0.599241616422144,1.,-2.09954930865331));
#47243=CARTESIAN_POINT('Ctrl Pts',(0.594585006052823,1.,-2.09510876220501));
#47244=CARTESIAN_POINT('Ctrl Pts',(0.589962365403189,1.,-2.09064881812053));
#47245=CARTESIAN_POINT('Ctrl Pts',(0.585373918990895,1.,-2.086169437277));
#47246=CARTESIAN_POINT('Ctrl Pts',(0.580819952107256,1.,-2.08167059018138));
#47247=CARTESIAN_POINT('Ctrl Pts',(0.576300797416274,1.,-2.07715226767361));
#47248=CARTESIAN_POINT('Ctrl Pts',(0.571816823242411,1.,-2.07261449292758));
#47249=CARTESIAN_POINT('Ctrl Pts',(0.567368421181229,1.,-2.06805732997383));
#47250=CARTESIAN_POINT('Ctrl Pts',(0.562955993082574,1.,-2.06348090160697));
#47251=CARTESIAN_POINT('Ctrl Pts',(0.558579940185467,1.,-2.05888537756571));
#47252=CARTESIAN_POINT('Ctrl Pts',(0.554240657464109,1.,-2.05427091604482));
#47253=CARTESIAN_POINT('Ctrl Pts',(0.549938525150342,1.,-2.04963761077974));
#47254=CARTESIAN_POINT('Ctrl Pts',(0.545673903817348,1.,-2.0449854471456));
#47255=CARTESIAN_POINT('Ctrl Pts',(0.54144712061552,1.,-2.0403142269048));
#47256=CARTESIAN_POINT('Ctrl Pts',(0.537258489833134,1.,-2.03562362953993));
#47257=CARTESIAN_POINT('Ctrl Pts',(0.533108355132905,1.,-2.03091336214401));
#47258=CARTESIAN_POINT('Ctrl Pts',(0.52899712724191,1.,-2.02618329083289));
#47259=CARTESIAN_POINT('Ctrl Pts',(0.524925318333518,1.,-2.02143356304712));
#47260=CARTESIAN_POINT('Ctrl Pts',(0.520893590399428,1.,-2.01666477917306));
#47261=CARTESIAN_POINT('Ctrl Pts',(0.516902681728733,1.,-2.01187773939257));
#47262=CARTESIAN_POINT('Ctrl Pts',(0.512953306961813,1.,-2.00707309946955));
#47263=CARTESIAN_POINT('Ctrl Pts',(0.509046069886152,1.,-2.00225107134733));
#47264=CARTESIAN_POINT('Ctrl Pts',(0.505181361323011,1.,-1.99741107463567));
#47265=CARTESIAN_POINT('Ctrl Pts',(0.501359287727129,1.,-1.9925514912615));
#47266=CARTESIAN_POINT('Ctrl Pts',(0.497579909545564,1.,-1.98767044752929));
#47267=CARTESIAN_POINT('Ctrl Pts',(0.493843476541492,1.,-1.9827665876182));
#47268=CARTESIAN_POINT('Ctrl Pts',(0.490150627860955,1.,-1.97783973019229));
#47269=CARTESIAN_POINT('Ctrl Pts',(0.486502692907661,1.,-1.97289186263272));
#47270=CARTESIAN_POINT('Ctrl Pts',(0.482901662120686,1.,-1.96792703422358));
#47271=CARTESIAN_POINT('Ctrl Pts',(0.479349583074846,1.,-1.96294933055938));
#47272=CARTESIAN_POINT('Ctrl Pts',(0.475848034683171,1.,-1.95796111148175));
#47273=CARTESIAN_POINT('Ctrl Pts',(0.472397672264079,1.,-1.95296148278136));
#47274=CARTESIAN_POINT('Ctrl Pts',(0.468997482913158,1.,-1.94794381136524));
#47275=CARTESIAN_POINT('Ctrl Pts',(0.465645462026064,1.,-1.94289794196205));
#47276=CARTESIAN_POINT('Ctrl Pts',(0.462340031009087,1.,-1.93781486640834));
#47277=CARTESIAN_POINT('Ctrl Pts',(0.459081234547931,1.,-1.93269066517936));
#47278=CARTESIAN_POINT('Ctrl Pts',(0.455872005174335,1.,-1.92753067150461));
#47279=CARTESIAN_POINT('Ctrl Pts',(0.452719478359356,1.,-1.9223538064847));
#47280=CARTESIAN_POINT('Ctrl Pts',(0.449632260106572,1.,-1.91718342555717));
#47281=CARTESIAN_POINT('Ctrl Pts',(0.446617343485651,1.,-1.91203699981095));
#47282=CARTESIAN_POINT('Ctrl Pts',(0.44367755684917,1.,-1.90691756144906));
#47283=CARTESIAN_POINT('Ctrl Pts',(0.44080783370416,1.,-1.90180124389137));
#47284=CARTESIAN_POINT('Ctrl Pts',(0.437995003948443,1.,-1.89663648956549));
#47285=CARTESIAN_POINT('Ctrl Pts',(0.43522566096358,1.,-1.89136993975585));
#47286=CARTESIAN_POINT('Ctrl Pts',(0.432493038548833,1.,-1.88596913666828));
#47287=CARTESIAN_POINT('Ctrl Pts',(0.429803062482217,1.,-1.88044229001779));
#47288=CARTESIAN_POINT('Ctrl Pts',(0.427183828518743,1.,-1.87486989291334));
#47289=CARTESIAN_POINT('Ctrl Pts',(0.424678177290876,1.,-1.8693780394412));
#47290=CARTESIAN_POINT('Ctrl Pts',(0.422327307417884,1.,-1.86408083333863));
#47291=CARTESIAN_POINT('Ctrl Pts',(0.420157287975583,1.,-1.8590328109667));
#47292=CARTESIAN_POINT('Ctrl Pts',(0.418164129144045,1.,-1.8541763285645));
#47293=CARTESIAN_POINT('Ctrl Pts',(0.416300022039885,1.,-1.84929312930314));
#47294=CARTESIAN_POINT('Ctrl Pts',(0.414487438255542,1.,-1.84405757074218));
#47295=CARTESIAN_POINT('Ctrl Pts',(0.412633125322945,1.,-1.8380895347617));
#47296=CARTESIAN_POINT('Ctrl Pts',(0.410641256301276,1.,-1.83100408895047));
#47297=CARTESIAN_POINT('Ctrl Pts',(0.408428948106227,1.,-1.82247022677562));
#47298=CARTESIAN_POINT('Ctrl Pts',(0.405933518407175,1.,-1.81223801812013));
#47299=CARTESIAN_POINT('Ctrl Pts',(0.403107976163396,1.,-1.80012077173238));
#47300=CARTESIAN_POINT('Ctrl Pts',(0.399919403774155,1.,-1.78598826343754));
#47301=CARTESIAN_POINT('Ctrl Pts',(0.396346196110688,1.,-1.76975560043442));
#47302=CARTESIAN_POINT('Ctrl Pts',(0.392375812285395,1.,-1.75137405310193));
#47303=CARTESIAN_POINT('Ctrl Pts',(0.388877023502615,1.,-1.73493170972829));
#47304=CARTESIAN_POINT('Ctrl Pts',(0.386070790323281,1.,-1.72162022244582));
#47305=CARTESIAN_POINT('Ctrl Pts',(0.384119047314215,1.,-1.71231062891398));
#47306=CARTESIAN_POINT('Ctrl Pts',(0.383122945602004,1.,-1.7075470150345));
#47307=CARTESIAN_POINT('',(0.61342227326009,0.,-2.11275013067528));
#47308=CARTESIAN_POINT('Origin',(0.745574324794401,0.,-2.0698113262342));
#47309=CARTESIAN_POINT('',(0.745574324794401,1.,-2.0698113262342));
#47310=CARTESIAN_POINT('',(0.61342227326009,1.,-2.11275013067528));
#47311=CARTESIAN_POINT('',(0.745574324794401,0.,-2.0698113262342));
#47312=CARTESIAN_POINT('Ctrl Pts',(0.693717979106306,-1.,-1.60662857109684));
#47313=CARTESIAN_POINT('Ctrl Pts',(0.693717979106306,1.,-1.60662857109684));
#47314=CARTESIAN_POINT('Ctrl Pts',(0.695712097881194,-1.,-1.61106790958151));
#47315=CARTESIAN_POINT('Ctrl Pts',(0.695712097881194,1.,-1.61106790958151));
#47316=CARTESIAN_POINT('Ctrl Pts',(0.699605146405088,-1.,-1.61974673472612));
#47317=CARTESIAN_POINT('Ctrl Pts',(0.699605146405088,1.,-1.61974673472612));
#47318=CARTESIAN_POINT('Ctrl Pts',(0.705159151988319,-1.,-1.63216541664676));
#47319=CARTESIAN_POINT('Ctrl Pts',(0.705159151988319,1.,-1.63216541664676));
#47320=CARTESIAN_POINT('Ctrl Pts',(0.711993139355394,-1.,-1.64752408832016));
#47321=CARTESIAN_POINT('Ctrl Pts',(0.711993139355394,1.,-1.64752408832016));
#47322=CARTESIAN_POINT('Ctrl Pts',(0.719585433804282,-1.,-1.6647288055568));
#47323=CARTESIAN_POINT('Ctrl Pts',(0.719585433804282,1.,-1.6647288055568));
#47324=CARTESIAN_POINT('Ctrl Pts',(0.726235967997433,-1.,-1.67996158455503));
#47325=CARTESIAN_POINT('Ctrl Pts',(0.726235967997433,1.,-1.67996158455503));
#47326=CARTESIAN_POINT('Ctrl Pts',(0.731963238697195,-1.,-1.69326921975743));
#47327=CARTESIAN_POINT('Ctrl Pts',(0.731963238697195,1.,-1.69326921975743));
#47328=CARTESIAN_POINT('Ctrl Pts',(0.736799665724771,-1.,-1.70473309006121));
#47329=CARTESIAN_POINT('Ctrl Pts',(0.736799665724771,1.,-1.70473309006121));
#47330=CARTESIAN_POINT('Ctrl Pts',(0.740795162032087,-1.,-1.71447789751927));
#47331=CARTESIAN_POINT('Ctrl Pts',(0.740795162032087,1.,-1.71447789751927));
#47332=CARTESIAN_POINT('Ctrl Pts',(0.744021445433764,-1.,-1.7226822991693));
#47333=CARTESIAN_POINT('Ctrl Pts',(0.744021445433764,1.,-1.7226822991693));
#47334=CARTESIAN_POINT('Ctrl Pts',(0.746574710096436,-1.,-1.72958533647399));
#47335=CARTESIAN_POINT('Ctrl Pts',(0.746574710096436,1.,-1.72958533647399));
#47336=CARTESIAN_POINT('Ctrl Pts',(0.748582462954854,-1.,-1.73550351679848));
#47337=CARTESIAN_POINT('Ctrl Pts',(0.748582462954854,1.,-1.73550351679848));
#47338=CARTESIAN_POINT('Ctrl Pts',(0.75019343597954,-1.,-1.74080458266705));
#47339=CARTESIAN_POINT('Ctrl Pts',(0.75019343597954,1.,-1.74080458266705));
#47340=CARTESIAN_POINT('Ctrl Pts',(0.751555614163629,-1.,-1.74585086852298));
#47341=CARTESIAN_POINT('Ctrl Pts',(0.751555614163629,1.,-1.74585086852298));
#47342=CARTESIAN_POINT('Ctrl Pts',(0.752797683531377,-1.,-1.75095139468809));
#47343=CARTESIAN_POINT('Ctrl Pts',(0.752797683531377,1.,-1.75095139468809));
#47344=CARTESIAN_POINT('Ctrl Pts',(0.75400925402848,-1.,-1.75631083600175));
#47345=CARTESIAN_POINT('Ctrl Pts',(0.75400925402848,1.,-1.75631083600175));
#47346=CARTESIAN_POINT('Ctrl Pts',(0.755220979975262,-1.,-1.7619781724032));
#47347=CARTESIAN_POINT('Ctrl Pts',(0.755220979975262,1.,-1.7619781724032));
#47348=CARTESIAN_POINT('Ctrl Pts',(0.756421896028403,-1.,-1.76789396003141));
#47349=CARTESIAN_POINT('Ctrl Pts',(0.756421896028403,1.,-1.76789396003141));
#47350=CARTESIAN_POINT('Ctrl Pts',(0.757578264077238,-1.,-1.77394167108342));
#47351=CARTESIAN_POINT('Ctrl Pts',(0.757578264077238,1.,-1.77394167108342));
#47352=CARTESIAN_POINT('Ctrl Pts',(0.75865062667738,-1.,-1.77999411220912));
#47353=CARTESIAN_POINT('Ctrl Pts',(0.75865062667738,1.,-1.77999411220912));
#47354=CARTESIAN_POINT('Ctrl Pts',(0.759614401109868,-1.,-1.78596964884527));
#47355=CARTESIAN_POINT('Ctrl Pts',(0.759614401109868,1.,-1.78596964884527));
#47356=CARTESIAN_POINT('Ctrl Pts',(0.760469555880425,-1.,-1.79185815610802));
#47357=CARTESIAN_POINT('Ctrl Pts',(0.760469555880425,1.,-1.79185815610802));
#47358=CARTESIAN_POINT('Ctrl Pts',(0.761229695230359,-1.,-1.79768986997735));
#47359=CARTESIAN_POINT('Ctrl Pts',(0.761229695230359,1.,-1.79768986997735));
#47360=CARTESIAN_POINT('Ctrl Pts',(0.761915336443515,-1.,-1.80351583877334));
#47361=CARTESIAN_POINT('Ctrl Pts',(0.761915336443515,1.,-1.80351583877334));
#47362=CARTESIAN_POINT('Ctrl Pts',(0.762546129464036,-1.,-1.80938551463989));
#47363=CARTESIAN_POINT('Ctrl Pts',(0.762546129464036,1.,-1.80938551463989));
#47364=CARTESIAN_POINT('Ctrl Pts',(0.763132003836783,-1.,-1.81532118405566));
#47365=CARTESIAN_POINT('Ctrl Pts',(0.763132003836783,1.,-1.81532118405566));
#47366=CARTESIAN_POINT('Ctrl Pts',(0.763673465462854,-1.,-1.82131873145297));
#47367=CARTESIAN_POINT('Ctrl Pts',(0.763673465462854,1.,-1.82131873145297));
#47368=CARTESIAN_POINT('Ctrl Pts',(0.764165902606055,-1.,-1.8273599120008));
#47369=CARTESIAN_POINT('Ctrl Pts',(0.764165902606055,1.,-1.8273599120008));
#47370=CARTESIAN_POINT('Ctrl Pts',(0.764602549687845,-1.,-1.8334207722714));
#47371=CARTESIAN_POINT('Ctrl Pts',(0.764602549687845,1.,-1.8334207722714));
#47372=CARTESIAN_POINT('Ctrl Pts',(0.764978057881687,-1.,-1.83948181064823));
#47373=CARTESIAN_POINT('Ctrl Pts',(0.764978057881687,1.,-1.83948181064823));
#47374=CARTESIAN_POINT('Ctrl Pts',(0.765291664861971,-1.,-1.84553698875911));
#47375=CARTESIAN_POINT('Ctrl Pts',(0.765291664861971,1.,-1.84553698875911));
#47376=CARTESIAN_POINT('Ctrl Pts',(0.765545710619023,-1.,-1.85158945130054));
#47377=CARTESIAN_POINT('Ctrl Pts',(0.765545710619023,1.,-1.85158945130054));
#47378=CARTESIAN_POINT('Ctrl Pts',(0.765744212909305,-1.,-1.85764741390391));
#47379=CARTESIAN_POINT('Ctrl Pts',(0.765744212909305,1.,-1.85764741390391));
#47380=CARTESIAN_POINT('Ctrl Pts',(0.765891519092557,-1.,-1.86372027063315));
#47381=CARTESIAN_POINT('Ctrl Pts',(0.765891519092557,1.,-1.86372027063315));
#47382=CARTESIAN_POINT('Ctrl Pts',(0.765990708546111,-1.,-1.86981398314345));
#47383=CARTESIAN_POINT('Ctrl Pts',(0.765990708546111,1.,-1.86981398314345));
#47384=CARTESIAN_POINT('Ctrl Pts',(0.766042837036759,-1.,-1.87592888967886));
#47385=CARTESIAN_POINT('Ctrl Pts',(0.766042837036759,1.,-1.87592888967886));
#47386=CARTESIAN_POINT('Ctrl Pts',(0.766047794851868,-1.,-1.88206215302561));
#47387=CARTESIAN_POINT('Ctrl Pts',(0.766047794851868,1.,-1.88206215302561));
#47388=CARTESIAN_POINT('Ctrl Pts',(0.76600483706209,-1.,-1.88820926433409));
#47389=CARTESIAN_POINT('Ctrl Pts',(0.76600483706209,1.,-1.88820926433409));
#47390=CARTESIAN_POINT('Ctrl Pts',(0.765913193856979,-1.,-1.89436577771389));
#47391=CARTESIAN_POINT('Ctrl Pts',(0.765913193856979,1.,-1.89436577771389));
#47392=CARTESIAN_POINT('Ctrl Pts',(0.765772772593395,-1.,-1.90052930393599));
#47393=CARTESIAN_POINT('Ctrl Pts',(0.765772772593395,1.,-1.90052930393599));
#47394=CARTESIAN_POINT('Ctrl Pts',(0.765584196937936,-1.,-1.90669961402362));
#47395=CARTESIAN_POINT('Ctrl Pts',(0.765584196937936,1.,-1.90669961402362));
#47396=CARTESIAN_POINT('Ctrl Pts',(0.765348465884739,-1.,-1.91287765805174));
#47397=CARTESIAN_POINT('Ctrl Pts',(0.765348465884739,1.,-1.91287765805174));
#47398=CARTESIAN_POINT('Ctrl Pts',(0.765066729667095,-1.,-1.91906491634197));
#47399=CARTESIAN_POINT('Ctrl Pts',(0.765066729667095,1.,-1.91906491634197));
#47400=CARTESIAN_POINT('Ctrl Pts',(0.764740025488189,-1.,-1.92526263537041));
#47401=CARTESIAN_POINT('Ctrl Pts',(0.764740025488189,1.,-1.92526263537041));
#47402=CARTESIAN_POINT('Ctrl Pts',(0.764369010673889,-1.,-1.93147105496367));
#47403=CARTESIAN_POINT('Ctrl Pts',(0.764369010673889,1.,-1.93147105496367));
#47404=CARTESIAN_POINT('Ctrl Pts',(0.763954049121393,-1.,-1.93768964875867));
#47405=CARTESIAN_POINT('Ctrl Pts',(0.763954049121393,1.,-1.93768964875867));
#47406=CARTESIAN_POINT('Ctrl Pts',(0.76349533353858,-1.,-1.94391746617626));
#47407=CARTESIAN_POINT('Ctrl Pts',(0.76349533353858,1.,-1.94391746617626));
#47408=CARTESIAN_POINT('Ctrl Pts',(0.762992990878774,-1.,-1.95015342590025));
#47409=CARTESIAN_POINT('Ctrl Pts',(0.762992990878774,1.,-1.95015342590025));
#47410=CARTESIAN_POINT('Ctrl Pts',(0.762447203806263,-1.,-1.95639665309893));
#47411=CARTESIAN_POINT('Ctrl Pts',(0.762447203806263,1.,-1.95639665309893));
#47412=CARTESIAN_POINT('Ctrl Pts',(0.761858300014575,-1.,-1.96264672744229));
#47413=CARTESIAN_POINT('Ctrl Pts',(0.761858300014575,1.,-1.96264672744229));
#47414=CARTESIAN_POINT('Ctrl Pts',(0.761226690483986,-1.,-1.96890351582545));
#47415=CARTESIAN_POINT('Ctrl Pts',(0.761226690483986,1.,-1.96890351582545));
#47416=CARTESIAN_POINT('Ctrl Pts',(0.760552825409855,-1.,-1.97516705321521));
#47417=CARTESIAN_POINT('Ctrl Pts',(0.760552825409855,1.,-1.97516705321521));
#47418=CARTESIAN_POINT('Ctrl Pts',(0.759837147452135,-1.,-1.98143741418156));
#47419=CARTESIAN_POINT('Ctrl Pts',(0.759837147452135,1.,-1.98143741418156));
#47420=CARTESIAN_POINT('Ctrl Pts',(0.759080037802242,-1.,-1.98771456680806));
#47421=CARTESIAN_POINT('Ctrl Pts',(0.759080037802242,1.,-1.98771456680806));
#47422=CARTESIAN_POINT('Ctrl Pts',(0.758281796766377,-1.,-1.9939983109871));
#47423=CARTESIAN_POINT('Ctrl Pts',(0.758281796766377,1.,-1.9939983109871));
#47424=CARTESIAN_POINT('Ctrl Pts',(0.757442676862341,-1.,-2.00028834739072));
#47425=CARTESIAN_POINT('Ctrl Pts',(0.757442676862341,1.,-2.00028834739072));
#47426=CARTESIAN_POINT('Ctrl Pts',(0.756562904646496,-1.,-2.00658431587682));
#47427=CARTESIAN_POINT('Ctrl Pts',(0.756562904646496,1.,-2.00658431587682));
#47428=CARTESIAN_POINT('Ctrl Pts',(0.7556427049581,-1.,-2.01288584328149));
#47429=CARTESIAN_POINT('Ctrl Pts',(0.7556427049581,1.,-2.01288584328149));
#47430=CARTESIAN_POINT('Ctrl Pts',(0.75468233072352,-1.,-2.01919259406003));
#47431=CARTESIAN_POINT('Ctrl Pts',(0.75468233072352,1.,-2.01919259406003));
#47432=CARTESIAN_POINT('Ctrl Pts',(0.753682061113765,-1.,-2.02550428623587));
#47433=CARTESIAN_POINT('Ctrl Pts',(0.753682061113765,1.,-2.02550428623587));
#47434=CARTESIAN_POINT('Ctrl Pts',(0.752642180488104,-1.,-2.03182068456467));
#47435=CARTESIAN_POINT('Ctrl Pts',(0.752642180488104,1.,-2.03182068456467));
#47436=CARTESIAN_POINT('Ctrl Pts',(0.751562963361383,-1.,-2.03814160092173));
#47437=CARTESIAN_POINT('Ctrl Pts',(0.751562963361383,1.,-2.03814160092173));
#47438=CARTESIAN_POINT('Ctrl Pts',(0.750444657874758,-1.,-2.04446689147754));
#47439=CARTESIAN_POINT('Ctrl Pts',(0.750444657874758,1.,-2.04446689147754));
#47440=CARTESIAN_POINT('Ctrl Pts',(0.749287468663053,-1.,-2.05079645591606));
#47441=CARTESIAN_POINT('Ctrl Pts',(0.749287468663053,1.,-2.05079645591606));
#47442=CARTESIAN_POINT('Ctrl Pts',(0.748091554181101,-1.,-2.05713023030263));
#47443=CARTESIAN_POINT('Ctrl Pts',(0.748091554181101,1.,-2.05713023030263));
#47444=CARTESIAN_POINT('Ctrl Pts',(0.747103932785504,-1.,-2.06220058927162));
#47445=CARTESIAN_POINT('Ctrl Pts',(0.747103932785504,1.,-2.06220058927162));
#47446=CARTESIAN_POINT('Ctrl Pts',(0.746345871542695,-1.,-2.06600523016401));
#47447=CARTESIAN_POINT('Ctrl Pts',(0.746345871542695,1.,-2.06600523016401));
#47448=CARTESIAN_POINT('Ctrl Pts',(0.74583279137781,-1.,-2.06854248895575));
#47449=CARTESIAN_POINT('Ctrl Pts',(0.74583279137781,1.,-2.06854248895575));
#47450=CARTESIAN_POINT('Ctrl Pts',(0.745574324794401,-1.,-2.0698113262342));
#47451=CARTESIAN_POINT('Ctrl Pts',(0.745574324794401,1.,-2.0698113262342));
#47452=CARTESIAN_POINT('',(0.693717979106306,1.,-1.60662857109684));
#47453=CARTESIAN_POINT('Ctrl Pts',(0.693717979106306,1.,-1.60662857109684));
#47454=CARTESIAN_POINT('Ctrl Pts',(0.695712097881194,1.,-1.61106790958151));
#47455=CARTESIAN_POINT('Ctrl Pts',(0.699605146405088,1.,-1.61974673472612));
#47456=CARTESIAN_POINT('Ctrl Pts',(0.705159151988319,1.,-1.63216541664676));
#47457=CARTESIAN_POINT('Ctrl Pts',(0.711993139355394,1.,-1.64752408832016));
#47458=CARTESIAN_POINT('Ctrl Pts',(0.719585433804282,1.,-1.6647288055568));
#47459=CARTESIAN_POINT('Ctrl Pts',(0.726235967997433,1.,-1.67996158455503));
#47460=CARTESIAN_POINT('Ctrl Pts',(0.731963238697195,1.,-1.69326921975743));
#47461=CARTESIAN_POINT('Ctrl Pts',(0.736799665724771,1.,-1.70473309006121));
#47462=CARTESIAN_POINT('Ctrl Pts',(0.740795162032087,1.,-1.71447789751927));
#47463=CARTESIAN_POINT('Ctrl Pts',(0.744021445433764,1.,-1.7226822991693));
#47464=CARTESIAN_POINT('Ctrl Pts',(0.746574710096436,1.,-1.72958533647399));
#47465=CARTESIAN_POINT('Ctrl Pts',(0.748582462954854,1.,-1.73550351679848));
#47466=CARTESIAN_POINT('Ctrl Pts',(0.75019343597954,1.,-1.74080458266705));
#47467=CARTESIAN_POINT('Ctrl Pts',(0.751555614163629,1.,-1.74585086852298));
#47468=CARTESIAN_POINT('Ctrl Pts',(0.752797683531377,1.,-1.75095139468809));
#47469=CARTESIAN_POINT('Ctrl Pts',(0.75400925402848,1.,-1.75631083600175));
#47470=CARTESIAN_POINT('Ctrl Pts',(0.755220979975262,1.,-1.7619781724032));
#47471=CARTESIAN_POINT('Ctrl Pts',(0.756421896028403,1.,-1.76789396003141));
#47472=CARTESIAN_POINT('Ctrl Pts',(0.757578264077238,1.,-1.77394167108342));
#47473=CARTESIAN_POINT('Ctrl Pts',(0.75865062667738,1.,-1.77999411220912));
#47474=CARTESIAN_POINT('Ctrl Pts',(0.759614401109868,1.,-1.78596964884527));
#47475=CARTESIAN_POINT('Ctrl Pts',(0.760469555880425,1.,-1.79185815610802));
#47476=CARTESIAN_POINT('Ctrl Pts',(0.761229695230359,1.,-1.79768986997735));
#47477=CARTESIAN_POINT('Ctrl Pts',(0.761915336443515,1.,-1.80351583877334));
#47478=CARTESIAN_POINT('Ctrl Pts',(0.762546129464036,1.,-1.80938551463989));
#47479=CARTESIAN_POINT('Ctrl Pts',(0.763132003836783,1.,-1.81532118405566));
#47480=CARTESIAN_POINT('Ctrl Pts',(0.763673465462854,1.,-1.82131873145297));
#47481=CARTESIAN_POINT('Ctrl Pts',(0.764165902606055,1.,-1.8273599120008));
#47482=CARTESIAN_POINT('Ctrl Pts',(0.764602549687845,1.,-1.8334207722714));
#47483=CARTESIAN_POINT('Ctrl Pts',(0.764978057881687,1.,-1.83948181064823));
#47484=CARTESIAN_POINT('Ctrl Pts',(0.765291664861971,1.,-1.84553698875911));
#47485=CARTESIAN_POINT('Ctrl Pts',(0.765545710619023,1.,-1.85158945130054));
#47486=CARTESIAN_POINT('Ctrl Pts',(0.765744212909305,1.,-1.85764741390391));
#47487=CARTESIAN_POINT('Ctrl Pts',(0.765891519092557,1.,-1.86372027063315));
#47488=CARTESIAN_POINT('Ctrl Pts',(0.765990708546111,1.,-1.86981398314345));
#47489=CARTESIAN_POINT('Ctrl Pts',(0.766042837036759,1.,-1.87592888967886));
#47490=CARTESIAN_POINT('Ctrl Pts',(0.766047794851868,1.,-1.88206215302561));
#47491=CARTESIAN_POINT('Ctrl Pts',(0.76600483706209,1.,-1.88820926433409));
#47492=CARTESIAN_POINT('Ctrl Pts',(0.765913193856979,1.,-1.89436577771389));
#47493=CARTESIAN_POINT('Ctrl Pts',(0.765772772593395,1.,-1.90052930393599));
#47494=CARTESIAN_POINT('Ctrl Pts',(0.765584196937936,1.,-1.90669961402362));
#47495=CARTESIAN_POINT('Ctrl Pts',(0.765348465884739,1.,-1.91287765805174));
#47496=CARTESIAN_POINT('Ctrl Pts',(0.765066729667095,1.,-1.91906491634197));
#47497=CARTESIAN_POINT('Ctrl Pts',(0.764740025488189,1.,-1.92526263537041));
#47498=CARTESIAN_POINT('Ctrl Pts',(0.764369010673889,1.,-1.93147105496367));
#47499=CARTESIAN_POINT('Ctrl Pts',(0.763954049121393,1.,-1.93768964875867));
#47500=CARTESIAN_POINT('Ctrl Pts',(0.76349533353858,1.,-1.94391746617626));
#47501=CARTESIAN_POINT('Ctrl Pts',(0.762992990878774,1.,-1.95015342590025));
#47502=CARTESIAN_POINT('Ctrl Pts',(0.762447203806263,1.,-1.95639665309893));
#47503=CARTESIAN_POINT('Ctrl Pts',(0.761858300014575,1.,-1.96264672744229));
#47504=CARTESIAN_POINT('Ctrl Pts',(0.761226690483986,1.,-1.96890351582545));
#47505=CARTESIAN_POINT('Ctrl Pts',(0.760552825409855,1.,-1.97516705321521));
#47506=CARTESIAN_POINT('Ctrl Pts',(0.759837147452135,1.,-1.98143741418156));
#47507=CARTESIAN_POINT('Ctrl Pts',(0.759080037802242,1.,-1.98771456680806));
#47508=CARTESIAN_POINT('Ctrl Pts',(0.758281796766377,1.,-1.9939983109871));
#47509=CARTESIAN_POINT('Ctrl Pts',(0.757442676862341,1.,-2.00028834739072));
#47510=CARTESIAN_POINT('Ctrl Pts',(0.756562904646496,1.,-2.00658431587682));
#47511=CARTESIAN_POINT('Ctrl Pts',(0.7556427049581,1.,-2.01288584328149));
#47512=CARTESIAN_POINT('Ctrl Pts',(0.75468233072352,1.,-2.01919259406003));
#47513=CARTESIAN_POINT('Ctrl Pts',(0.753682061113765,1.,-2.02550428623587));
#47514=CARTESIAN_POINT('Ctrl Pts',(0.752642180488104,1.,-2.03182068456467));
#47515=CARTESIAN_POINT('Ctrl Pts',(0.751562963361383,1.,-2.03814160092173));
#47516=CARTESIAN_POINT('Ctrl Pts',(0.750444657874758,1.,-2.04446689147754));
#47517=CARTESIAN_POINT('Ctrl Pts',(0.749287468663053,1.,-2.05079645591606));
#47518=CARTESIAN_POINT('Ctrl Pts',(0.748091554181101,1.,-2.05713023030263));
#47519=CARTESIAN_POINT('Ctrl Pts',(0.747103932785504,1.,-2.06220058927162));
#47520=CARTESIAN_POINT('Ctrl Pts',(0.746345871542695,1.,-2.06600523016401));
#47521=CARTESIAN_POINT('Ctrl Pts',(0.74583279137781,1.,-2.06854248895575));
#47522=CARTESIAN_POINT('Ctrl Pts',(0.745574324794401,1.,-2.0698113262342));
#47523=CARTESIAN_POINT('',(0.693717979106306,0.,-1.60662857109684));
#47524=CARTESIAN_POINT('Origin',(0.,0.,0.));
#47525=CARTESIAN_POINT('',(0.892032620296855,1.,-1.5055822144029));
#47526=CARTESIAN_POINT('Origin',(0.,1.,0.));
#47527=CARTESIAN_POINT('',(0.892032620296855,0.,-1.5055822144029));
#47528=CARTESIAN_POINT('Ctrl Pts',(1.23627494547115,-1.,-1.81978687191668));
#47529=CARTESIAN_POINT('Ctrl Pts',(1.23627494547115,1.,-1.81978687191668));
#47530=CARTESIAN_POINT('Ctrl Pts',(1.23509651170476,-1.,-1.81925017193666));
#47531=CARTESIAN_POINT('Ctrl Pts',(1.23509651170476,1.,-1.81925017193666));
#47532=CARTESIAN_POINT('Ctrl Pts',(1.2327422452705,-1.,-1.81817389921279));
#47533=CARTESIAN_POINT('Ctrl Pts',(1.2327422452705,1.,-1.81817389921279));
#47534=CARTESIAN_POINT('Ctrl Pts',(1.2292186489137,-1.,-1.8165508718364));
#47535=CARTESIAN_POINT('Ctrl Pts',(1.2292186489137,1.,-1.8165508718364));
#47536=CARTESIAN_POINT('Ctrl Pts',(1.2245361330495,-1.,-1.81436959210434));
#47537=CARTESIAN_POINT('Ctrl Pts',(1.2245361330495,1.,-1.81436959210434));
#47538=CARTESIAN_POINT('Ctrl Pts',(1.21870906103557,-1.,-1.81161420806656));
#47539=CARTESIAN_POINT('Ctrl Pts',(1.21870906103557,1.,-1.81161420806656));
#47540=CARTESIAN_POINT('Ctrl Pts',(1.21290815708314,-1.,-1.80882996917129));
#47541=CARTESIAN_POINT('Ctrl Pts',(1.21290815708314,1.,-1.80882996917129));
#47542=CARTESIAN_POINT('Ctrl Pts',(1.20713356605475,-1.,-1.80601678480707));
#47543=CARTESIAN_POINT('Ctrl Pts',(1.20713356605475,1.,-1.80601678480707));
#47544=CARTESIAN_POINT('Ctrl Pts',(1.20138548938974,-1.,-1.80317454838603));
#47545=CARTESIAN_POINT('Ctrl Pts',(1.20138548938974,1.,-1.80317454838603));
#47546=CARTESIAN_POINT('Ctrl Pts',(1.19566418930242,-1.,-1.80030314369879));
#47547=CARTESIAN_POINT('Ctrl Pts',(1.19566418930242,1.,-1.80030314369879));
#47548=CARTESIAN_POINT('Ctrl Pts',(1.18996997934445,-1.,-1.79740245923478));
#47549=CARTESIAN_POINT('Ctrl Pts',(1.18996997934445,1.,-1.79740245923478));
#47550=CARTESIAN_POINT('Ctrl Pts',(1.18430321697432,-1.,-1.79447240321515));
#47551=CARTESIAN_POINT('Ctrl Pts',(1.18430321697432,1.,-1.79447240321515));
#47552=CARTESIAN_POINT('Ctrl Pts',(1.17866429440809,-1.,-1.79151291552689));
#47553=CARTESIAN_POINT('Ctrl Pts',(1.17866429440809,1.,-1.79151291552689));
#47554=CARTESIAN_POINT('Ctrl Pts',(1.17305363177328,-1.,-1.78852398877617));
#47555=CARTESIAN_POINT('Ctrl Pts',(1.17305363177328,1.,-1.78852398877617));
#47556=CARTESIAN_POINT('Ctrl Pts',(1.16747166312303,-1.,-1.78550566040443));
#47557=CARTESIAN_POINT('Ctrl Pts',(1.16747166312303,1.,-1.78550566040443));
#47558=CARTESIAN_POINT('Ctrl Pts',(1.16191881298499,-1.,-1.78245795881009));
#47559=CARTESIAN_POINT('Ctrl Pts',(1.16191881298499,1.,-1.78245795881009));
#47560=CARTESIAN_POINT('Ctrl Pts',(1.15639547194698,-1.,-1.77938085564275));
#47561=CARTESIAN_POINT('Ctrl Pts',(1.15639547194698,1.,-1.77938085564275));
#47562=CARTESIAN_POINT('Ctrl Pts',(1.15090197841514,-1.,-1.7762742255701));
#47563=CARTESIAN_POINT('Ctrl Pts',(1.15090197841514,1.,-1.7762742255701));
#47564=CARTESIAN_POINT('Ctrl Pts',(1.1454385822692,-1.,-1.77313777896194));
#47565=CARTESIAN_POINT('Ctrl Pts',(1.1454385822692,1.,-1.77313777896194));
#47566=CARTESIAN_POINT('Ctrl Pts',(1.14000548336975,-1.,-1.76997111386769));
#47567=CARTESIAN_POINT('Ctrl Pts',(1.14000548336975,1.,-1.76997111386769));
#47568=CARTESIAN_POINT('Ctrl Pts',(1.1346029180462,-1.,-1.76677384551862));
#47569=CARTESIAN_POINT('Ctrl Pts',(1.1346029180462,1.,-1.76677384551862));
#47570=CARTESIAN_POINT('Ctrl Pts',(1.12923123555075,-1.,-1.7635457196617));
#47571=CARTESIAN_POINT('Ctrl Pts',(1.12923123555075,1.,-1.7635457196617));
#47572=CARTESIAN_POINT('Ctrl Pts',(1.12389096855086,-1.,-1.76028671825096));
#47573=CARTESIAN_POINT('Ctrl Pts',(1.12389096855086,1.,-1.76028671825096));
#47574=CARTESIAN_POINT('Ctrl Pts',(1.11858293216763,-1.,-1.75699720772105));
#47575=CARTESIAN_POINT('Ctrl Pts',(1.11858293216763,1.,-1.75699720772105));
#47576=CARTESIAN_POINT('Ctrl Pts',(1.11330807582551,-1.,-1.7536777209463));
#47577=CARTESIAN_POINT('Ctrl Pts',(1.11330807582551,1.,-1.7536777209463));
#47578=CARTESIAN_POINT('Ctrl Pts',(1.10806728183007,-1.,-1.7503286607592));
#47579=CARTESIAN_POINT('Ctrl Pts',(1.10806728183007,1.,-1.7503286607592));
#47580=CARTESIAN_POINT('Ctrl Pts',(1.10286118991143,-1.,-1.74695004214923));
#47581=CARTESIAN_POINT('Ctrl Pts',(1.10286118991143,1.,-1.74695004214923));
#47582=CARTESIAN_POINT('Ctrl Pts',(1.09768999241225,-1.,-1.74354119236208));
#47583=CARTESIAN_POINT('Ctrl Pts',(1.09768999241225,1.,-1.74354119236208));
#47584=CARTESIAN_POINT('Ctrl Pts',(1.09255329056493,-1.,-1.74010053962247));
#47585=CARTESIAN_POINT('Ctrl Pts',(1.09255329056493,1.,-1.74010053962247));
#47586=CARTESIAN_POINT('Ctrl Pts',(1.08745056285427,-1.,-1.73662628326091));
#47587=CARTESIAN_POINT('Ctrl Pts',(1.08745056285427,1.,-1.73662628326091));
#47588=CARTESIAN_POINT('Ctrl Pts',(1.08238162784749,-1.,-1.73311705663407));
#47589=CARTESIAN_POINT('Ctrl Pts',(1.08238162784749,1.,-1.73311705663407));
#47590=CARTESIAN_POINT('Ctrl Pts',(1.0773470373727,-1.,-1.72957248977424));
#47591=CARTESIAN_POINT('Ctrl Pts',(1.0773470373727,1.,-1.72957248977424));
#47592=CARTESIAN_POINT('Ctrl Pts',(1.07234866990252,-1.,-1.72599406198488));
#47593=CARTESIAN_POINT('Ctrl Pts',(1.07234866990252,1.,-1.72599406198488));
#47594=CARTESIAN_POINT('Ctrl Pts',(1.06738966975462,-1.,-1.72238500928453));
#47595=CARTESIAN_POINT('Ctrl Pts',(1.06738966975462,1.,-1.72238500928453));
#47596=CARTESIAN_POINT('Ctrl Pts',(1.06247324680647,-1.,-1.71874858456904));
#47597=CARTESIAN_POINT('Ctrl Pts',(1.06247324680647,1.,-1.71874858456904));
#47598=CARTESIAN_POINT('Ctrl Pts',(1.05760163192479,-1.,-1.7150865442702));
#47599=CARTESIAN_POINT('Ctrl Pts',(1.05760163192479,1.,-1.7150865442702));
#47600=CARTESIAN_POINT('Ctrl Pts',(1.05277517202855,-1.,-1.71139783543989));
#47601=CARTESIAN_POINT('Ctrl Pts',(1.05277517202855,1.,-1.71139783543989));
#47602=CARTESIAN_POINT('Ctrl Pts',(1.04799085404995,-1.,-1.70767646263649));
#47603=CARTESIAN_POINT('Ctrl Pts',(1.04799085404995,1.,-1.70767646263649));
#47604=CARTESIAN_POINT('Ctrl Pts',(1.04324363334554,-1.,-1.70391338707982));
#47605=CARTESIAN_POINT('Ctrl Pts',(1.04324363334554,1.,-1.70391338707982));
#47606=CARTESIAN_POINT('Ctrl Pts',(1.03852922490789,-1.,-1.70010052930962));
#47607=CARTESIAN_POINT('Ctrl Pts',(1.03852922490789,1.,-1.70010052930962));
#47608=CARTESIAN_POINT('Ctrl Pts',(1.03384646003588,-1.,-1.69623414782771));
#47609=CARTESIAN_POINT('Ctrl Pts',(1.03384646003588,1.,-1.69623414782771));
#47610=CARTESIAN_POINT('Ctrl Pts',(1.02919977579147,-1.,-1.69231840863458));
#47611=CARTESIAN_POINT('Ctrl Pts',(1.02919977579147,1.,-1.69231840863458));
#47612=CARTESIAN_POINT('Ctrl Pts',(1.02460180535255,-1.,-1.68836910178447));
#47613=CARTESIAN_POINT('Ctrl Pts',(1.02460180535255,1.,-1.68836910178447));
#47614=CARTESIAN_POINT('Ctrl Pts',(1.02006795074201,-1.,-1.68440578021706));
#47615=CARTESIAN_POINT('Ctrl Pts',(1.02006795074201,1.,-1.68440578021706));
#47616=CARTESIAN_POINT('Ctrl Pts',(1.01561026162773,-1.,-1.68044289894798));
#47617=CARTESIAN_POINT('Ctrl Pts',(1.01561026162773,1.,-1.68044289894798));
#47618=CARTESIAN_POINT('Ctrl Pts',(1.01123236493511,-1.,-1.67648246776464));
#47619=CARTESIAN_POINT('Ctrl Pts',(1.01123236493511,1.,-1.67648246776464));
#47620=CARTESIAN_POINT('Ctrl Pts',(1.00692206696414,-1.,-1.67250335383293));
#47621=CARTESIAN_POINT('Ctrl Pts',(1.00692206696414,1.,-1.67250335383293));
#47622=CARTESIAN_POINT('Ctrl Pts',(1.00265091003727,-1.,-1.66846059277303));
#47623=CARTESIAN_POINT('Ctrl Pts',(1.00265091003727,1.,-1.66846059277303));
#47624=CARTESIAN_POINT('Ctrl Pts',(0.998389654952757,-1.,-1.66430758030376));
#47625=CARTESIAN_POINT('Ctrl Pts',(0.998389654952757,1.,-1.66430758030376));
#47626=CARTESIAN_POINT('Ctrl Pts',(0.994121836661305,-1.,-1.66001553809947));
#47627=CARTESIAN_POINT('Ctrl Pts',(0.994121836661305,1.,-1.66001553809947));
#47628=CARTESIAN_POINT('Ctrl Pts',(0.989855627854164,-1.,-1.65559044289699));
#47629=CARTESIAN_POINT('Ctrl Pts',(0.989855627854164,1.,-1.65559044289699));
#47630=CARTESIAN_POINT('Ctrl Pts',(0.98564262292082,-1.,-1.65110016612638));
#47631=CARTESIAN_POINT('Ctrl Pts',(0.98564262292082,1.,-1.65110016612638));
#47632=CARTESIAN_POINT('Ctrl Pts',(0.981562530939489,-1.,-1.64665139190656));
#47633=CARTESIAN_POINT('Ctrl Pts',(0.981562530939489,1.,-1.64665139190656));
#47634=CARTESIAN_POINT('Ctrl Pts',(0.977689794119416,-1.,-1.64233990826687));
#47635=CARTESIAN_POINT('Ctrl Pts',(0.977689794119416,1.,-1.64233990826687));
#47636=CARTESIAN_POINT('Ctrl Pts',(0.974066058287418,-1.,-1.63820952658144));
#47637=CARTESIAN_POINT('Ctrl Pts',(0.974066058287418,1.,-1.63820952658144));
#47638=CARTESIAN_POINT('Ctrl Pts',(0.970669715997509,-1.,-1.63420665729798));
#47639=CARTESIAN_POINT('Ctrl Pts',(0.970669715997509,1.,-1.63420665729798));
#47640=CARTESIAN_POINT('Ctrl Pts',(0.967387853230345,-1.,-1.63013849959462));
#47641=CARTESIAN_POINT('Ctrl Pts',(0.967387853230345,1.,-1.63013849959462));
#47642=CARTESIAN_POINT('Ctrl Pts',(0.964046107040535,-1.,-1.62571930670187));
#47643=CARTESIAN_POINT('Ctrl Pts',(0.964046107040535,1.,-1.62571930670187));
#47644=CARTESIAN_POINT('Ctrl Pts',(0.960438326101728,-1.,-1.62061638140221));
#47645=CARTESIAN_POINT('Ctrl Pts',(0.960438326101728,1.,-1.62061638140221));
#47646=CARTESIAN_POINT('Ctrl Pts',(0.95635442292067,-1.,-1.61449324337085));
#47647=CARTESIAN_POINT('Ctrl Pts',(0.95635442292067,1.,-1.61449324337085));
#47648=CARTESIAN_POINT('Ctrl Pts',(0.951613284356035,-1.,-1.60706069896936));
#47649=CARTESIAN_POINT('Ctrl Pts',(0.951613284356035,1.,-1.60706069896936));
#47650=CARTESIAN_POINT('Ctrl Pts',(0.946078063315257,-1.,-1.59810042043673));
#47651=CARTESIAN_POINT('Ctrl Pts',(0.946078063315257,1.,-1.59810042043673));
#47652=CARTESIAN_POINT('Ctrl Pts',(0.939646377893399,-1.,-1.58744937487176));
#47653=CARTESIAN_POINT('Ctrl Pts',(0.939646377893399,1.,-1.58744937487176));
#47654=CARTESIAN_POINT('Ctrl Pts',(0.932246680108685,-1.,-1.57499388382243));
#47655=CARTESIAN_POINT('Ctrl Pts',(0.932246680108685,1.,-1.57499388382243));
#47656=CARTESIAN_POINT('Ctrl Pts',(0.923832188944341,-1.,-1.56065988578893));
#47657=CARTESIAN_POINT('Ctrl Pts',(0.923832188944341,1.,-1.56065988578893));
#47658=CARTESIAN_POINT('Ctrl Pts',(0.914375919026456,-1.,-1.54440491149498));
#47659=CARTESIAN_POINT('Ctrl Pts',(0.914375919026456,1.,-1.54440491149498));
#47660=CARTESIAN_POINT('Ctrl Pts',(0.905967409625651,-1.,-1.52984849887993));
#47661=CARTESIAN_POINT('Ctrl Pts',(0.905967409625651,1.,-1.52984849887993));
#47662=CARTESIAN_POINT('Ctrl Pts',(0.89918504748351,-1.,-1.51805569590094));
#47663=CARTESIAN_POINT('Ctrl Pts',(0.89918504748351,1.,-1.51805569590094));
#47664=CARTESIAN_POINT('Ctrl Pts',(0.894452006964543,-1.,-1.50980486806688));
#47665=CARTESIAN_POINT('Ctrl Pts',(0.894452006964543,1.,-1.50980486806688));
#47666=CARTESIAN_POINT('Ctrl Pts',(0.892032620296855,-1.,-1.5055822144029));
#47667=CARTESIAN_POINT('Ctrl Pts',(0.892032620296855,1.,-1.5055822144029));
#47668=CARTESIAN_POINT('',(1.23627494547115,1.,-1.81978687191668));
#47669=CARTESIAN_POINT('Ctrl Pts',(1.23627494547115,1.,-1.81978687191668));
#47670=CARTESIAN_POINT('Ctrl Pts',(1.23509651170476,1.,-1.81925017193666));
#47671=CARTESIAN_POINT('Ctrl Pts',(1.2327422452705,1.,-1.81817389921279));
#47672=CARTESIAN_POINT('Ctrl Pts',(1.2292186489137,1.,-1.8165508718364));
#47673=CARTESIAN_POINT('Ctrl Pts',(1.2245361330495,1.,-1.81436959210434));
#47674=CARTESIAN_POINT('Ctrl Pts',(1.21870906103557,1.,-1.81161420806656));
#47675=CARTESIAN_POINT('Ctrl Pts',(1.21290815708314,1.,-1.80882996917129));
#47676=CARTESIAN_POINT('Ctrl Pts',(1.20713356605475,1.,-1.80601678480707));
#47677=CARTESIAN_POINT('Ctrl Pts',(1.20138548938974,1.,-1.80317454838603));
#47678=CARTESIAN_POINT('Ctrl Pts',(1.19566418930242,1.,-1.80030314369879));
#47679=CARTESIAN_POINT('Ctrl Pts',(1.18996997934445,1.,-1.79740245923478));
#47680=CARTESIAN_POINT('Ctrl Pts',(1.18430321697432,1.,-1.79447240321515));
#47681=CARTESIAN_POINT('Ctrl Pts',(1.17866429440809,1.,-1.79151291552689));
#47682=CARTESIAN_POINT('Ctrl Pts',(1.17305363177328,1.,-1.78852398877617));
#47683=CARTESIAN_POINT('Ctrl Pts',(1.16747166312303,1.,-1.78550566040443));
#47684=CARTESIAN_POINT('Ctrl Pts',(1.16191881298499,1.,-1.78245795881009));
#47685=CARTESIAN_POINT('Ctrl Pts',(1.15639547194698,1.,-1.77938085564275));
#47686=CARTESIAN_POINT('Ctrl Pts',(1.15090197841514,1.,-1.7762742255701));
#47687=CARTESIAN_POINT('Ctrl Pts',(1.1454385822692,1.,-1.77313777896194));
#47688=CARTESIAN_POINT('Ctrl Pts',(1.14000548336975,1.,-1.76997111386769));
#47689=CARTESIAN_POINT('Ctrl Pts',(1.1346029180462,1.,-1.76677384551862));
#47690=CARTESIAN_POINT('Ctrl Pts',(1.12923123555075,1.,-1.7635457196617));
#47691=CARTESIAN_POINT('Ctrl Pts',(1.12389096855086,1.,-1.76028671825096));
#47692=CARTESIAN_POINT('Ctrl Pts',(1.11858293216763,1.,-1.75699720772105));
#47693=CARTESIAN_POINT('Ctrl Pts',(1.11330807582551,1.,-1.7536777209463));
#47694=CARTESIAN_POINT('Ctrl Pts',(1.10806728183007,1.,-1.7503286607592));
#47695=CARTESIAN_POINT('Ctrl Pts',(1.10286118991143,1.,-1.74695004214923));
#47696=CARTESIAN_POINT('Ctrl Pts',(1.09768999241225,1.,-1.74354119236208));
#47697=CARTESIAN_POINT('Ctrl Pts',(1.09255329056493,1.,-1.74010053962247));
#47698=CARTESIAN_POINT('Ctrl Pts',(1.08745056285427,1.,-1.73662628326091));
#47699=CARTESIAN_POINT('Ctrl Pts',(1.08238162784749,1.,-1.73311705663407));
#47700=CARTESIAN_POINT('Ctrl Pts',(1.0773470373727,1.,-1.72957248977424));
#47701=CARTESIAN_POINT('Ctrl Pts',(1.07234866990252,1.,-1.72599406198488));
#47702=CARTESIAN_POINT('Ctrl Pts',(1.06738966975462,1.,-1.72238500928453));
#47703=CARTESIAN_POINT('Ctrl Pts',(1.06247324680647,1.,-1.71874858456904));
#47704=CARTESIAN_POINT('Ctrl Pts',(1.05760163192479,1.,-1.7150865442702));
#47705=CARTESIAN_POINT('Ctrl Pts',(1.05277517202855,1.,-1.71139783543989));
#47706=CARTESIAN_POINT('Ctrl Pts',(1.04799085404995,1.,-1.70767646263649));
#47707=CARTESIAN_POINT('Ctrl Pts',(1.04324363334554,1.,-1.70391338707982));
#47708=CARTESIAN_POINT('Ctrl Pts',(1.03852922490789,1.,-1.70010052930962));
#47709=CARTESIAN_POINT('Ctrl Pts',(1.03384646003588,1.,-1.69623414782771));
#47710=CARTESIAN_POINT('Ctrl Pts',(1.02919977579147,1.,-1.69231840863458));
#47711=CARTESIAN_POINT('Ctrl Pts',(1.02460180535255,1.,-1.68836910178447));
#47712=CARTESIAN_POINT('Ctrl Pts',(1.02006795074201,1.,-1.68440578021706));
#47713=CARTESIAN_POINT('Ctrl Pts',(1.01561026162773,1.,-1.68044289894798));
#47714=CARTESIAN_POINT('Ctrl Pts',(1.01123236493511,1.,-1.67648246776464));
#47715=CARTESIAN_POINT('Ctrl Pts',(1.00692206696414,1.,-1.67250335383293));
#47716=CARTESIAN_POINT('Ctrl Pts',(1.00265091003727,1.,-1.66846059277303));
#47717=CARTESIAN_POINT('Ctrl Pts',(0.998389654952757,1.,-1.66430758030376));
#47718=CARTESIAN_POINT('Ctrl Pts',(0.994121836661305,1.,-1.66001553809947));
#47719=CARTESIAN_POINT('Ctrl Pts',(0.989855627854164,1.,-1.65559044289699));
#47720=CARTESIAN_POINT('Ctrl Pts',(0.98564262292082,1.,-1.65110016612638));
#47721=CARTESIAN_POINT('Ctrl Pts',(0.981562530939489,1.,-1.64665139190656));
#47722=CARTESIAN_POINT('Ctrl Pts',(0.977689794119416,1.,-1.64233990826687));
#47723=CARTESIAN_POINT('Ctrl Pts',(0.974066058287418,1.,-1.63820952658144));
#47724=CARTESIAN_POINT('Ctrl Pts',(0.970669715997509,1.,-1.63420665729798));
#47725=CARTESIAN_POINT('Ctrl Pts',(0.967387853230345,1.,-1.63013849959462));
#47726=CARTESIAN_POINT('Ctrl Pts',(0.964046107040535,1.,-1.62571930670187));
#47727=CARTESIAN_POINT('Ctrl Pts',(0.960438326101728,1.,-1.62061638140221));
#47728=CARTESIAN_POINT('Ctrl Pts',(0.95635442292067,1.,-1.61449324337085));
#47729=CARTESIAN_POINT('Ctrl Pts',(0.951613284356035,1.,-1.60706069896936));
#47730=CARTESIAN_POINT('Ctrl Pts',(0.946078063315257,1.,-1.59810042043673));
#47731=CARTESIAN_POINT('Ctrl Pts',(0.939646377893399,1.,-1.58744937487176));
#47732=CARTESIAN_POINT('Ctrl Pts',(0.932246680108685,1.,-1.57499388382243));
#47733=CARTESIAN_POINT('Ctrl Pts',(0.923832188944341,1.,-1.56065988578893));
#47734=CARTESIAN_POINT('Ctrl Pts',(0.914375919026456,1.,-1.54440491149498));
#47735=CARTESIAN_POINT('Ctrl Pts',(0.905967409625651,1.,-1.52984849887993));
#47736=CARTESIAN_POINT('Ctrl Pts',(0.89918504748351,1.,-1.51805569590094));
#47737=CARTESIAN_POINT('Ctrl Pts',(0.894452006964543,1.,-1.50980486806688));
#47738=CARTESIAN_POINT('Ctrl Pts',(0.892032620296855,1.,-1.5055822144029));
#47739=CARTESIAN_POINT('',(1.23627494547115,0.,-1.81978687191668));
#47740=CARTESIAN_POINT('Origin',(1.34869019493419,0.,-1.73811241238545));
#47741=CARTESIAN_POINT('',(1.34869019493419,1.,-1.73811241238545));
#47742=CARTESIAN_POINT('',(1.23627494547115,1.,-1.81978687191668));
#47743=CARTESIAN_POINT('',(1.34869019493419,0.,-1.73811241238545));
#47744=CARTESIAN_POINT('Ctrl Pts',(1.15624053661742,-1.,-1.31362392696032));
#47745=CARTESIAN_POINT('Ctrl Pts',(1.15624053661742,1.,-1.31362392696032));
#47746=CARTESIAN_POINT('Ctrl Pts',(1.15950888730809,-1.,-1.31722977216397));
#47747=CARTESIAN_POINT('Ctrl Pts',(1.15950888730809,1.,-1.31722977216397));
#47748=CARTESIAN_POINT('Ctrl Pts',(1.16589330093588,-1.,-1.32428080721772));
#47749=CARTESIAN_POINT('Ctrl Pts',(1.16589330093588,1.,-1.32428080721772));
#47750=CARTESIAN_POINT('Ctrl Pts',(1.17501305789857,-1.,-1.33437539347008));
#47751=CARTESIAN_POINT('Ctrl Pts',(1.17501305789857,1.,-1.33437539347008));
#47752=CARTESIAN_POINT('Ctrl Pts',(1.18625865667441,-1.,-1.34687054001093));
#47753=CARTESIAN_POINT('Ctrl Pts',(1.18625865667441,1.,-1.34687054001093));
#47754=CARTESIAN_POINT('Ctrl Pts',(1.1987959077932,-1.,-1.36088705043885));
#47755=CARTESIAN_POINT('Ctrl Pts',(1.1987959077932,1.,-1.36088705043885));
#47756=CARTESIAN_POINT('Ctrl Pts',(1.20982812925645,-1.,-1.37331915607905));
#47757=CARTESIAN_POINT('Ctrl Pts',(1.20982812925645,1.,-1.37331915607905));
#47758=CARTESIAN_POINT('Ctrl Pts',(1.21938737280852,-1.,-1.38420564527715));
#47759=CARTESIAN_POINT('Ctrl Pts',(1.21938737280852,1.,-1.38420564527715));
#47760=CARTESIAN_POINT('Ctrl Pts',(1.22752961899387,-1.,-1.39361389568796));
#47761=CARTESIAN_POINT('Ctrl Pts',(1.22752961899387,1.,-1.39361389568796));
#47762=CARTESIAN_POINT('Ctrl Pts',(1.23434087290423,-1.,-1.40164708206106));
#47763=CARTESIAN_POINT('Ctrl Pts',(1.23434087290423,1.,-1.40164708206106));
#47764=CARTESIAN_POINT('Ctrl Pts',(1.23994455029534,-1.,-1.40845295531283));
#47765=CARTESIAN_POINT('Ctrl Pts',(1.23994455029534,1.,-1.40845295531283));
#47766=CARTESIAN_POINT('Ctrl Pts',(1.24450600513056,-1.,-1.41422913175179));
#47767=CARTESIAN_POINT('Ctrl Pts',(1.24450600513056,1.,-1.41422913175179));
#47768=CARTESIAN_POINT('Ctrl Pts',(1.24824430986571,-1.,-1.41923722596025));
#47769=CARTESIAN_POINT('Ctrl Pts',(1.24824430986571,1.,-1.41923722596025));
#47770=CARTESIAN_POINT('Ctrl Pts',(1.2514145557001,-1.,-1.42378102115575));
#47771=CARTESIAN_POINT('Ctrl Pts',(1.2514145557001,1.,-1.42378102115575));
#47772=CARTESIAN_POINT('Ctrl Pts',(1.25426945222639,-1.,-1.42815938799387));
#47773=CARTESIAN_POINT('Ctrl Pts',(1.25426945222639,1.,-1.42815938799387));
#47774=CARTESIAN_POINT('Ctrl Pts',(1.25702687965755,-1.,-1.43262645609691));
#47775=CARTESIAN_POINT('Ctrl Pts',(1.25702687965755,1.,-1.43262645609691));
#47776=CARTESIAN_POINT('Ctrl Pts',(1.25983531012005,-1.,-1.43734919180848));
#47777=CARTESIAN_POINT('Ctrl Pts',(1.25983531012005,1.,-1.43734919180848));
#47778=CARTESIAN_POINT('Ctrl Pts',(1.26273903323858,-1.,-1.44236470511303));
#47779=CARTESIAN_POINT('Ctrl Pts',(1.26273903323858,1.,-1.44236470511303));
#47780=CARTESIAN_POINT('Ctrl Pts',(1.26570925118868,-1.,-1.44761985001662));
#47781=CARTESIAN_POINT('Ctrl Pts',(1.26570925118868,1.,-1.44761985001662));
#47782=CARTESIAN_POINT('Ctrl Pts',(1.2686778680489,-1.,-1.45301422764247));
#47783=CARTESIAN_POINT('Ctrl Pts',(1.2686778680489,1.,-1.45301422764247));
#47784=CARTESIAN_POINT('Ctrl Pts',(1.27156805265289,-1.,-1.45843906294697));
#47785=CARTESIAN_POINT('Ctrl Pts',(1.27156805265289,1.,-1.45843906294697));
#47786=CARTESIAN_POINT('Ctrl Pts',(1.27433119897822,-1.,-1.46382431332476));
#47787=CARTESIAN_POINT('Ctrl Pts',(1.27433119897822,1.,-1.46382431332476));
#47788=CARTESIAN_POINT('Ctrl Pts',(1.27696414831089,-1.,-1.46916035917133));
#47789=CARTESIAN_POINT('Ctrl Pts',(1.27696414831089,1.,-1.46916035917133));
#47790=CARTESIAN_POINT('Ctrl Pts',(1.2794891824849,-1.,-1.4744717526707));
#47791=CARTESIAN_POINT('Ctrl Pts',(1.2794891824849,1.,-1.4744717526707));
#47792=CARTESIAN_POINT('Ctrl Pts',(1.28194158939517,-1.,-1.47980070347096));
#47793=CARTESIAN_POINT('Ctrl Pts',(1.28194158939517,1.,-1.47980070347096));
#47794=CARTESIAN_POINT('Ctrl Pts',(1.28435533880201,-1.,-1.4851881711891));
#47795=CARTESIAN_POINT('Ctrl Pts',(1.28435533880201,1.,-1.4851881711891));
#47796=CARTESIAN_POINT('Ctrl Pts',(1.2867467611644,-1.,-1.4906522831278));
#47797=CARTESIAN_POINT('Ctrl Pts',(1.2867467611644,1.,-1.4906522831278));
#47798=CARTESIAN_POINT('Ctrl Pts',(1.28911506584254,-1.,-1.49618896881754));
#47799=CARTESIAN_POINT('Ctrl Pts',(1.28911506584254,1.,-1.49618896881754));
#47800=CARTESIAN_POINT('Ctrl Pts',(1.29145022885181,-1.,-1.50178230149776));
#47801=CARTESIAN_POINT('Ctrl Pts',(1.29145022885181,1.,-1.50178230149776));
#47802=CARTESIAN_POINT('Ctrl Pts',(1.29373841372842,-1.,-1.50741159078365));
#47803=CARTESIAN_POINT('Ctrl Pts',(1.29373841372842,1.,-1.50741159078365));
#47804=CARTESIAN_POINT('Ctrl Pts',(1.29596850710509,-1.,-1.51305994241402));
#47805=CARTESIAN_POINT('Ctrl Pts',(1.29596850710509,1.,-1.51305994241402));
#47806=CARTESIAN_POINT('Ctrl Pts',(1.29813791800747,-1.,-1.51872184912724));
#47807=CARTESIAN_POINT('Ctrl Pts',(1.29813791800747,1.,-1.51872184912724));
#47808=CARTESIAN_POINT('Ctrl Pts',(1.30024984366328,-1.,-1.52439957861062));
#47809=CARTESIAN_POINT('Ctrl Pts',(1.30024984366328,1.,-1.52439957861062));
#47810=CARTESIAN_POINT('Ctrl Pts',(1.30231064395568,-1.,-1.53009970283891));
#47811=CARTESIAN_POINT('Ctrl Pts',(1.30231064395568,1.,-1.53009970283891));
#47812=CARTESIAN_POINT('Ctrl Pts',(1.30432735639489,-1.,-1.53582981268977));
#47813=CARTESIAN_POINT('Ctrl Pts',(1.30432735639489,1.,-1.53582981268977));
#47814=CARTESIAN_POINT('Ctrl Pts',(1.30630475189556,-1.,-1.54159462645432));
#47815=CARTESIAN_POINT('Ctrl Pts',(1.30630475189556,1.,-1.54159462645432));
#47816=CARTESIAN_POINT('Ctrl Pts',(1.30824393907473,-1.,-1.54739413957185));
#47817=CARTESIAN_POINT('Ctrl Pts',(1.30824393907473,1.,-1.54739413957185));
#47818=CARTESIAN_POINT('Ctrl Pts',(1.31014393684222,-1.,-1.55322568759481));
#47819=CARTESIAN_POINT('Ctrl Pts',(1.31014393684222,1.,-1.55322568759481));
#47820=CARTESIAN_POINT('Ctrl Pts',(1.31200264341696,-1.,-1.55908521254821));
#47821=CARTESIAN_POINT('Ctrl Pts',(1.31200264341696,1.,-1.55908521254821));
#47822=CARTESIAN_POINT('Ctrl Pts',(1.31381795281002,-1.,-1.56496872402353));
#47823=CARTESIAN_POINT('Ctrl Pts',(1.31381795281002,1.,-1.56496872402353));
#47824=CARTESIAN_POINT('Ctrl Pts',(1.31558903860016,-1.,-1.57087397835723));
#47825=CARTESIAN_POINT('Ctrl Pts',(1.31558903860016,1.,-1.57087397835723));
#47826=CARTESIAN_POINT('Ctrl Pts',(1.31731642317187,-1.,-1.5768005650559));
#47827=CARTESIAN_POINT('Ctrl Pts',(1.31731642317187,1.,-1.5768005650559));
#47828=CARTESIAN_POINT('Ctrl Pts',(1.31900135021432,-1.,-1.58274907898834));
#47829=CARTESIAN_POINT('Ctrl Pts',(1.31900135021432,1.,-1.58274907898834));
#47830=CARTESIAN_POINT('Ctrl Pts',(1.32064537110892,-1.,-1.58872057258245));
#47831=CARTESIAN_POINT('Ctrl Pts',(1.32064537110892,1.,-1.58872057258245));
#47832=CARTESIAN_POINT('Ctrl Pts',(1.32224985747682,-1.,-1.59471591079403));
#47833=CARTESIAN_POINT('Ctrl Pts',(1.32224985747682,1.,-1.59471591079403));
#47834=CARTESIAN_POINT('Ctrl Pts',(1.32381550858256,-1.,-1.60073511858687));
#47835=CARTESIAN_POINT('Ctrl Pts',(1.32381550858256,1.,-1.60073511858687));
#47836=CARTESIAN_POINT('Ctrl Pts',(1.32534250785782,-1.,-1.60677758290954));
#47837=CARTESIAN_POINT('Ctrl Pts',(1.32534250785782,1.,-1.60677758290954));
#47838=CARTESIAN_POINT('Ctrl Pts',(1.32683074483356,-1.,-1.6128423401575));
#47839=CARTESIAN_POINT('Ctrl Pts',(1.32683074483356,1.,-1.6128423401575));
#47840=CARTESIAN_POINT('Ctrl Pts',(1.32828000610449,-1.,-1.61892832270724));
#47841=CARTESIAN_POINT('Ctrl Pts',(1.32828000610449,1.,-1.61892832270724));
#47842=CARTESIAN_POINT('Ctrl Pts',(1.3296901950568,-1.,-1.62503464209797));
#47843=CARTESIAN_POINT('Ctrl Pts',(1.3296901950568,1.,-1.62503464209797));
#47844=CARTESIAN_POINT('Ctrl Pts',(1.33106149345645,-1.,-1.63116079730923));
#47845=CARTESIAN_POINT('Ctrl Pts',(1.33106149345645,1.,-1.63116079730923));
#47846=CARTESIAN_POINT('Ctrl Pts',(1.33239425103724,-1.,-1.63730653475089));
#47847=CARTESIAN_POINT('Ctrl Pts',(1.33239425103724,1.,-1.63730653475089));
#47848=CARTESIAN_POINT('Ctrl Pts',(1.33368890676572,-1.,-1.6434717485603));
#47849=CARTESIAN_POINT('Ctrl Pts',(1.33368890676572,1.,-1.6434717485603));
#47850=CARTESIAN_POINT('Ctrl Pts',(1.33494590467993,-1.,-1.6496563728683));
#47851=CARTESIAN_POINT('Ctrl Pts',(1.33494590467993,1.,-1.6496563728683));
#47852=CARTESIAN_POINT('Ctrl Pts',(1.33616559745172,-1.,-1.65586025952593));
#47853=CARTESIAN_POINT('Ctrl Pts',(1.33616559745172,1.,-1.65586025952593));
#47854=CARTESIAN_POINT('Ctrl Pts',(1.33734820885262,-1.,-1.66208312541983));
#47855=CARTESIAN_POINT('Ctrl Pts',(1.33734820885262,1.,-1.66208312541983));
#47856=CARTESIAN_POINT('Ctrl Pts',(1.33849388654388,-1.,-1.66832460783989));
#47857=CARTESIAN_POINT('Ctrl Pts',(1.33849388654388,1.,-1.66832460783989));
#47858=CARTESIAN_POINT('Ctrl Pts',(1.3396027347034,-1.,-1.67458429426086));
#47859=CARTESIAN_POINT('Ctrl Pts',(1.3396027347034,1.,-1.67458429426086));
#47860=CARTESIAN_POINT('Ctrl Pts',(1.34067485185203,-1.,-1.68086176030362));
#47861=CARTESIAN_POINT('Ctrl Pts',(1.34067485185203,1.,-1.68086176030362));
#47862=CARTESIAN_POINT('Ctrl Pts',(1.341710374848,-1.,-1.68715660868764));
#47863=CARTESIAN_POINT('Ctrl Pts',(1.341710374848,1.,-1.68715660868764));
#47864=CARTESIAN_POINT('Ctrl Pts',(1.34270948206319,-1.,-1.6934684849687));
#47865=CARTESIAN_POINT('Ctrl Pts',(1.34270948206319,1.,-1.6934684849687));
#47866=CARTESIAN_POINT('Ctrl Pts',(1.34367237124483,-1.,-1.69979707754427));
#47867=CARTESIAN_POINT('Ctrl Pts',(1.34367237124483,1.,-1.69979707754427));
#47868=CARTESIAN_POINT('Ctrl Pts',(1.34459924533831,-1.,-1.70614212266738));
#47869=CARTESIAN_POINT('Ctrl Pts',(1.34459924533831,1.,-1.70614212266738));
#47870=CARTESIAN_POINT('Ctrl Pts',(1.34549029589416,-1.,-1.71250340686822));
#47871=CARTESIAN_POINT('Ctrl Pts',(1.34549029589416,1.,-1.71250340686822));
#47872=CARTESIAN_POINT('Ctrl Pts',(1.34634568653227,-1.,-1.7188807715049));
#47873=CARTESIAN_POINT('Ctrl Pts',(1.34634568653227,1.,-1.7188807715049));
#47874=CARTESIAN_POINT('Ctrl Pts',(1.34716554819527,-1.,-1.72527410680674));
#47875=CARTESIAN_POINT('Ctrl Pts',(1.34716554819527,1.,-1.72527410680674));
#47876=CARTESIAN_POINT('Ctrl Pts',(1.34779309152035,-1.,-1.7304014965394));
#47877=CARTESIAN_POINT('Ctrl Pts',(1.34779309152035,1.,-1.7304014965394));
#47878=CARTESIAN_POINT('Ctrl Pts',(1.34824783112887,-1.,-1.73425417885907));
#47879=CARTESIAN_POINT('Ctrl Pts',(1.34824783112887,1.,-1.73425417885907));
#47880=CARTESIAN_POINT('Ctrl Pts',(1.34854391898045,-1.,-1.73682580585691));
#47881=CARTESIAN_POINT('Ctrl Pts',(1.34854391898045,1.,-1.73682580585691));
#47882=CARTESIAN_POINT('Ctrl Pts',(1.34869019493419,-1.,-1.73811241238545));
#47883=CARTESIAN_POINT('Ctrl Pts',(1.34869019493419,1.,-1.73811241238545));
#47884=CARTESIAN_POINT('',(1.15624053661742,1.,-1.31362392696032));
#47885=CARTESIAN_POINT('Ctrl Pts',(1.15624053661742,1.,-1.31362392696032));
#47886=CARTESIAN_POINT('Ctrl Pts',(1.15950888730809,1.,-1.31722977216397));
#47887=CARTESIAN_POINT('Ctrl Pts',(1.16589330093588,1.,-1.32428080721772));
#47888=CARTESIAN_POINT('Ctrl Pts',(1.17501305789857,1.,-1.33437539347008));
#47889=CARTESIAN_POINT('Ctrl Pts',(1.18625865667441,1.,-1.34687054001093));
#47890=CARTESIAN_POINT('Ctrl Pts',(1.1987959077932,1.,-1.36088705043885));
#47891=CARTESIAN_POINT('Ctrl Pts',(1.20982812925645,1.,-1.37331915607905));
#47892=CARTESIAN_POINT('Ctrl Pts',(1.21938737280852,1.,-1.38420564527715));
#47893=CARTESIAN_POINT('Ctrl Pts',(1.22752961899387,1.,-1.39361389568796));
#47894=CARTESIAN_POINT('Ctrl Pts',(1.23434087290423,1.,-1.40164708206106));
#47895=CARTESIAN_POINT('Ctrl Pts',(1.23994455029534,1.,-1.40845295531283));
#47896=CARTESIAN_POINT('Ctrl Pts',(1.24450600513056,1.,-1.41422913175179));
#47897=CARTESIAN_POINT('Ctrl Pts',(1.24824430986571,1.,-1.41923722596025));
#47898=CARTESIAN_POINT('Ctrl Pts',(1.2514145557001,1.,-1.42378102115575));
#47899=CARTESIAN_POINT('Ctrl Pts',(1.25426945222639,1.,-1.42815938799387));
#47900=CARTESIAN_POINT('Ctrl Pts',(1.25702687965755,1.,-1.43262645609691));
#47901=CARTESIAN_POINT('Ctrl Pts',(1.25983531012005,1.,-1.43734919180848));
#47902=CARTESIAN_POINT('Ctrl Pts',(1.26273903323858,1.,-1.44236470511303));
#47903=CARTESIAN_POINT('Ctrl Pts',(1.26570925118868,1.,-1.44761985001662));
#47904=CARTESIAN_POINT('Ctrl Pts',(1.2686778680489,1.,-1.45301422764247));
#47905=CARTESIAN_POINT('Ctrl Pts',(1.27156805265289,1.,-1.45843906294697));
#47906=CARTESIAN_POINT('Ctrl Pts',(1.27433119897822,1.,-1.46382431332476));
#47907=CARTESIAN_POINT('Ctrl Pts',(1.27696414831089,1.,-1.46916035917133));
#47908=CARTESIAN_POINT('Ctrl Pts',(1.2794891824849,1.,-1.4744717526707));
#47909=CARTESIAN_POINT('Ctrl Pts',(1.28194158939517,1.,-1.47980070347096));
#47910=CARTESIAN_POINT('Ctrl Pts',(1.28435533880201,1.,-1.4851881711891));
#47911=CARTESIAN_POINT('Ctrl Pts',(1.2867467611644,1.,-1.4906522831278));
#47912=CARTESIAN_POINT('Ctrl Pts',(1.28911506584254,1.,-1.49618896881754));
#47913=CARTESIAN_POINT('Ctrl Pts',(1.29145022885181,1.,-1.50178230149776));
#47914=CARTESIAN_POINT('Ctrl Pts',(1.29373841372842,1.,-1.50741159078365));
#47915=CARTESIAN_POINT('Ctrl Pts',(1.29596850710509,1.,-1.51305994241402));
#47916=CARTESIAN_POINT('Ctrl Pts',(1.29813791800747,1.,-1.51872184912724));
#47917=CARTESIAN_POINT('Ctrl Pts',(1.30024984366328,1.,-1.52439957861062));
#47918=CARTESIAN_POINT('Ctrl Pts',(1.30231064395568,1.,-1.53009970283891));
#47919=CARTESIAN_POINT('Ctrl Pts',(1.30432735639489,1.,-1.53582981268977));
#47920=CARTESIAN_POINT('Ctrl Pts',(1.30630475189556,1.,-1.54159462645432));
#47921=CARTESIAN_POINT('Ctrl Pts',(1.30824393907473,1.,-1.54739413957185));
#47922=CARTESIAN_POINT('Ctrl Pts',(1.31014393684222,1.,-1.55322568759481));
#47923=CARTESIAN_POINT('Ctrl Pts',(1.31200264341696,1.,-1.55908521254821));
#47924=CARTESIAN_POINT('Ctrl Pts',(1.31381795281002,1.,-1.56496872402353));
#47925=CARTESIAN_POINT('Ctrl Pts',(1.31558903860016,1.,-1.57087397835723));
#47926=CARTESIAN_POINT('Ctrl Pts',(1.31731642317187,1.,-1.5768005650559));
#47927=CARTESIAN_POINT('Ctrl Pts',(1.31900135021432,1.,-1.58274907898834));
#47928=CARTESIAN_POINT('Ctrl Pts',(1.32064537110892,1.,-1.58872057258245));
#47929=CARTESIAN_POINT('Ctrl Pts',(1.32224985747682,1.,-1.59471591079403));
#47930=CARTESIAN_POINT('Ctrl Pts',(1.32381550858256,1.,-1.60073511858687));
#47931=CARTESIAN_POINT('Ctrl Pts',(1.32534250785782,1.,-1.60677758290954));
#47932=CARTESIAN_POINT('Ctrl Pts',(1.32683074483356,1.,-1.6128423401575));
#47933=CARTESIAN_POINT('Ctrl Pts',(1.32828000610449,1.,-1.61892832270724));
#47934=CARTESIAN_POINT('Ctrl Pts',(1.3296901950568,1.,-1.62503464209797));
#47935=CARTESIAN_POINT('Ctrl Pts',(1.33106149345645,1.,-1.63116079730923));
#47936=CARTESIAN_POINT('Ctrl Pts',(1.33239425103724,1.,-1.63730653475089));
#47937=CARTESIAN_POINT('Ctrl Pts',(1.33368890676572,1.,-1.6434717485603));
#47938=CARTESIAN_POINT('Ctrl Pts',(1.33494590467993,1.,-1.6496563728683));
#47939=CARTESIAN_POINT('Ctrl Pts',(1.33616559745172,1.,-1.65586025952593));
#47940=CARTESIAN_POINT('Ctrl Pts',(1.33734820885262,1.,-1.66208312541983));
#47941=CARTESIAN_POINT('Ctrl Pts',(1.33849388654388,1.,-1.66832460783989));
#47942=CARTESIAN_POINT('Ctrl Pts',(1.3396027347034,1.,-1.67458429426086));
#47943=CARTESIAN_POINT('Ctrl Pts',(1.34067485185203,1.,-1.68086176030362));
#47944=CARTESIAN_POINT('Ctrl Pts',(1.341710374848,1.,-1.68715660868764));
#47945=CARTESIAN_POINT('Ctrl Pts',(1.34270948206319,1.,-1.6934684849687));
#47946=CARTESIAN_POINT('Ctrl Pts',(1.34367237124483,1.,-1.69979707754427));
#47947=CARTESIAN_POINT('Ctrl Pts',(1.34459924533831,1.,-1.70614212266738));
#47948=CARTESIAN_POINT('Ctrl Pts',(1.34549029589416,1.,-1.71250340686822));
#47949=CARTESIAN_POINT('Ctrl Pts',(1.34634568653227,1.,-1.7188807715049));
#47950=CARTESIAN_POINT('Ctrl Pts',(1.34716554819527,1.,-1.72527410680674));
#47951=CARTESIAN_POINT('Ctrl Pts',(1.34779309152035,1.,-1.7304014965394));
#47952=CARTESIAN_POINT('Ctrl Pts',(1.34824783112887,1.,-1.73425417885907));
#47953=CARTESIAN_POINT('Ctrl Pts',(1.34854391898045,1.,-1.73682580585691));
#47954=CARTESIAN_POINT('Ctrl Pts',(1.34869019493419,1.,-1.73811241238545));
#47955=CARTESIAN_POINT('',(1.15624053661742,0.,-1.31362392696032));
#47956=CARTESIAN_POINT('Origin',(0.,0.,0.));
#47957=CARTESIAN_POINT('',(1.31362392696032,1.,-1.15624053661742));
#47958=CARTESIAN_POINT('Origin',(0.,1.,0.));
#47959=CARTESIAN_POINT('',(1.31362392696032,0.,-1.15624053661742));
#47960=CARTESIAN_POINT('Ctrl Pts',(1.73811241238545,-1.,-1.34869019493419));
#47961=CARTESIAN_POINT('Ctrl Pts',(1.73811241238545,1.,-1.34869019493419));
#47962=CARTESIAN_POINT('Ctrl Pts',(1.73682580585819,-1.,-1.34854391898145));
#47963=CARTESIAN_POINT('Ctrl Pts',(1.73682580585819,1.,-1.34854391898145));
#47964=CARTESIAN_POINT('Ctrl Pts',(1.73425417886254,-1.,-1.34824783113158));
#47965=CARTESIAN_POINT('Ctrl Pts',(1.73425417886254,1.,-1.34824783113158));
#47966=CARTESIAN_POINT('Ctrl Pts',(1.73040149654497,-1.,-1.3477930915247));
#47967=CARTESIAN_POINT('Ctrl Pts',(1.73040149654497,1.,-1.3477930915247));
#47968=CARTESIAN_POINT('Ctrl Pts',(1.72527410681298,-1.,-1.34716554820013));
#47969=CARTESIAN_POINT('Ctrl Pts',(1.72527410681298,1.,-1.34716554820013));
#47970=CARTESIAN_POINT('Ctrl Pts',(1.7188807715095,-1.,-1.34634568653586));
#47971=CARTESIAN_POINT('Ctrl Pts',(1.7188807715095,1.,-1.34634568653586));
#47972=CARTESIAN_POINT('Ctrl Pts',(1.71250340687011,-1.,-1.34549029589563));
#47973=CARTESIAN_POINT('Ctrl Pts',(1.71250340687011,1.,-1.34549029589563));
#47974=CARTESIAN_POINT('Ctrl Pts',(1.70614212266676,-1.,-1.34459924533783));
#47975=CARTESIAN_POINT('Ctrl Pts',(1.70614212266676,1.,-1.34459924533783));
#47976=CARTESIAN_POINT('Ctrl Pts',(1.69979707754221,-1.,-1.34367237124322));
#47977=CARTESIAN_POINT('Ctrl Pts',(1.69979707754221,1.,-1.34367237124322));
#47978=CARTESIAN_POINT('Ctrl Pts',(1.6934684849664,-1.,-1.34270948206139));
#47979=CARTESIAN_POINT('Ctrl Pts',(1.6934684849664,1.,-1.34270948206139));
#47980=CARTESIAN_POINT('Ctrl Pts',(1.68715660868602,-1.,-1.34171037484673));
#47981=CARTESIAN_POINT('Ctrl Pts',(1.68715660868602,1.,-1.34171037484673));
#47982=CARTESIAN_POINT('Ctrl Pts',(1.68086176030308,-1.,-1.3406748518516));
#47983=CARTESIAN_POINT('Ctrl Pts',(1.68086176030308,1.,-1.3406748518516));
#47984=CARTESIAN_POINT('Ctrl Pts',(1.67458429426126,-1.,-1.33960273470372));
#47985=CARTESIAN_POINT('Ctrl Pts',(1.67458429426126,1.,-1.33960273470372));
#47986=CARTESIAN_POINT('Ctrl Pts',(1.66832460784078,-1.,-1.33849388654458));
#47987=CARTESIAN_POINT('Ctrl Pts',(1.66832460784078,1.,-1.33849388654458));
#47988=CARTESIAN_POINT('Ctrl Pts',(1.66208312542073,-1.,-1.33734820885331));
#47989=CARTESIAN_POINT('Ctrl Pts',(1.66208312542073,1.,-1.33734820885331));
#47990=CARTESIAN_POINT('Ctrl Pts',(1.65586025952651,-1.,-1.33616559745217));
#47991=CARTESIAN_POINT('Ctrl Pts',(1.65586025952651,1.,-1.33616559745217));
#47992=CARTESIAN_POINT('Ctrl Pts',(1.64965637286843,-1.,-1.33494590468003));
#47993=CARTESIAN_POINT('Ctrl Pts',(1.64965637286843,1.,-1.33494590468003));
#47994=CARTESIAN_POINT('Ctrl Pts',(1.64347174856007,-1.,-1.33368890676554));
#47995=CARTESIAN_POINT('Ctrl Pts',(1.64347174856007,1.,-1.33368890676554));
#47996=CARTESIAN_POINT('Ctrl Pts',(1.63730653475049,-1.,-1.33239425103694));
#47997=CARTESIAN_POINT('Ctrl Pts',(1.63730653475049,1.,-1.33239425103694));
#47998=CARTESIAN_POINT('Ctrl Pts',(1.63116079730887,-1.,-1.33106149345618));
#47999=CARTESIAN_POINT('Ctrl Pts',(1.63116079730887,1.,-1.33106149345618));
#48000=CARTESIAN_POINT('Ctrl Pts',(1.62503464209777,-1.,-1.32969019505665));
#48001=CARTESIAN_POINT('Ctrl Pts',(1.62503464209777,1.,-1.32969019505665));
#48002=CARTESIAN_POINT('Ctrl Pts',(1.61892832270723,-1.,-1.32828000610448));
#48003=CARTESIAN_POINT('Ctrl Pts',(1.61892832270723,1.,-1.32828000610448));
#48004=CARTESIAN_POINT('Ctrl Pts',(1.61284234015762,-1.,-1.32683074483365));
#48005=CARTESIAN_POINT('Ctrl Pts',(1.61284234015762,1.,-1.32683074483365));
#48006=CARTESIAN_POINT('Ctrl Pts',(1.6067775829097,-1.,-1.32534250785794));
#48007=CARTESIAN_POINT('Ctrl Pts',(1.6067775829097,1.,-1.32534250785794));
#48008=CARTESIAN_POINT('Ctrl Pts',(1.600735118587,-1.,-1.32381550858266));
#48009=CARTESIAN_POINT('Ctrl Pts',(1.600735118587,1.,-1.32381550858266));
#48010=CARTESIAN_POINT('Ctrl Pts',(1.59471591079408,-1.,-1.32224985747686));
#48011=CARTESIAN_POINT('Ctrl Pts',(1.59471591079408,1.,-1.32224985747686));
#48012=CARTESIAN_POINT('Ctrl Pts',(1.58872057258244,-1.,-1.32064537110891));
#48013=CARTESIAN_POINT('Ctrl Pts',(1.58872057258244,1.,-1.32064537110891));
#48014=CARTESIAN_POINT('Ctrl Pts',(1.58274907898829,-1.,-1.31900135021428));
#48015=CARTESIAN_POINT('Ctrl Pts',(1.58274907898829,1.,-1.31900135021428));
#48016=CARTESIAN_POINT('Ctrl Pts',(1.57680056505585,-1.,-1.31731642317183));
#48017=CARTESIAN_POINT('Ctrl Pts',(1.57680056505585,1.,-1.31731642317183));
#48018=CARTESIAN_POINT('Ctrl Pts',(1.57087397835721,-1.,-1.31558903860015));
#48019=CARTESIAN_POINT('Ctrl Pts',(1.57087397835721,1.,-1.31558903860015));
#48020=CARTESIAN_POINT('Ctrl Pts',(1.56496872402352,-1.,-1.31381795281002));
#48021=CARTESIAN_POINT('Ctrl Pts',(1.56496872402352,1.,-1.31381795281002));
#48022=CARTESIAN_POINT('Ctrl Pts',(1.55908521254822,-1.,-1.31200264341696));
#48023=CARTESIAN_POINT('Ctrl Pts',(1.55908521254822,1.,-1.31200264341696));
#48024=CARTESIAN_POINT('Ctrl Pts',(1.55322568759481,-1.,-1.31014393684221));
#48025=CARTESIAN_POINT('Ctrl Pts',(1.55322568759481,1.,-1.31014393684221));
#48026=CARTESIAN_POINT('Ctrl Pts',(1.54739413957183,-1.,-1.30824393907471));
#48027=CARTESIAN_POINT('Ctrl Pts',(1.54739413957183,1.,-1.30824393907471));
#48028=CARTESIAN_POINT('Ctrl Pts',(1.54159462645428,-1.,-1.30630475189553));
#48029=CARTESIAN_POINT('Ctrl Pts',(1.54159462645428,1.,-1.30630475189553));
#48030=CARTESIAN_POINT('Ctrl Pts',(1.53582981268976,-1.,-1.30432735639487));
#48031=CARTESIAN_POINT('Ctrl Pts',(1.53582981268976,1.,-1.30432735639487));
#48032=CARTESIAN_POINT('Ctrl Pts',(1.53009970283893,-1.,-1.3023106439557));
#48033=CARTESIAN_POINT('Ctrl Pts',(1.53009970283893,1.,-1.3023106439557));
#48034=CARTESIAN_POINT('Ctrl Pts',(1.5243995786107,-1.,-1.30024984366334));
#48035=CARTESIAN_POINT('Ctrl Pts',(1.5243995786107,1.,-1.30024984366334));
#48036=CARTESIAN_POINT('Ctrl Pts',(1.51872184912735,-1.,-1.29813791800757));
#48037=CARTESIAN_POINT('Ctrl Pts',(1.51872184912735,1.,-1.29813791800757));
#48038=CARTESIAN_POINT('Ctrl Pts',(1.51305994241412,-1.,-1.29596850710518));
#48039=CARTESIAN_POINT('Ctrl Pts',(1.51305994241412,1.,-1.29596850710518));
#48040=CARTESIAN_POINT('Ctrl Pts',(1.50741159078367,-1.,-1.29373841372843));
#48041=CARTESIAN_POINT('Ctrl Pts',(1.50741159078367,1.,-1.29373841372843));
#48042=CARTESIAN_POINT('Ctrl Pts',(1.50178230149764,-1.,-1.29145022885171));
#48043=CARTESIAN_POINT('Ctrl Pts',(1.50178230149764,1.,-1.29145022885171));
#48044=CARTESIAN_POINT('Ctrl Pts',(1.49618896881729,-1.,-1.28911506584232));
#48045=CARTESIAN_POINT('Ctrl Pts',(1.49618896881729,1.,-1.28911506584232));
#48046=CARTESIAN_POINT('Ctrl Pts',(1.4906522831275,-1.,-1.28674676116415));
#48047=CARTESIAN_POINT('Ctrl Pts',(1.4906522831275,1.,-1.28674676116415));
#48048=CARTESIAN_POINT('Ctrl Pts',(1.48518817118891,-1.,-1.28435533880184));
#48049=CARTESIAN_POINT('Ctrl Pts',(1.48518817118891,1.,-1.28435533880184));
#48050=CARTESIAN_POINT('Ctrl Pts',(1.47980070347102,-1.,-1.28194158939522));
#48051=CARTESIAN_POINT('Ctrl Pts',(1.47980070347102,1.,-1.28194158939522));
#48052=CARTESIAN_POINT('Ctrl Pts',(1.4744717526711,-1.,-1.27948918248524));
#48053=CARTESIAN_POINT('Ctrl Pts',(1.4744717526711,1.,-1.27948918248524));
#48054=CARTESIAN_POINT('Ctrl Pts',(1.46916035917197,-1.,-1.27696414831144));
#48055=CARTESIAN_POINT('Ctrl Pts',(1.46916035917197,1.,-1.27696414831144));
#48056=CARTESIAN_POINT('Ctrl Pts',(1.4638243133254,-1.,-1.27433119897877));
#48057=CARTESIAN_POINT('Ctrl Pts',(1.4638243133254,1.,-1.27433119897877));
#48058=CARTESIAN_POINT('Ctrl Pts',(1.45843906294725,-1.,-1.27156805265312));
#48059=CARTESIAN_POINT('Ctrl Pts',(1.45843906294725,1.,-1.27156805265312));
#48060=CARTESIAN_POINT('Ctrl Pts',(1.45301422764205,-1.,-1.26867786804854));
#48061=CARTESIAN_POINT('Ctrl Pts',(1.45301422764205,1.,-1.26867786804854));
#48062=CARTESIAN_POINT('Ctrl Pts',(1.44761985001544,-1.,-1.26570925118767));
#48063=CARTESIAN_POINT('Ctrl Pts',(1.44761985001544,1.,-1.26570925118767));
#48064=CARTESIAN_POINT('Ctrl Pts',(1.44236470511145,-1.,-1.26273903323723));
#48065=CARTESIAN_POINT('Ctrl Pts',(1.44236470511145,1.,-1.26273903323723));
#48066=CARTESIAN_POINT('Ctrl Pts',(1.43734919180719,-1.,-1.25983531011894));
#48067=CARTESIAN_POINT('Ctrl Pts',(1.43734919180719,1.,-1.25983531011894));
#48068=CARTESIAN_POINT('Ctrl Pts',(1.43262645609679,-1.,-1.25702687965744));
#48069=CARTESIAN_POINT('Ctrl Pts',(1.43262645609679,1.,-1.25702687965744));
#48070=CARTESIAN_POINT('Ctrl Pts',(1.42815938799555,-1.,-1.25426945222783));
#48071=CARTESIAN_POINT('Ctrl Pts',(1.42815938799555,1.,-1.25426945222783));
#48072=CARTESIAN_POINT('Ctrl Pts',(1.42378102115911,-1.,-1.25141455570299));
#48073=CARTESIAN_POINT('Ctrl Pts',(1.42378102115911,1.,-1.25141455570299));
#48074=CARTESIAN_POINT('Ctrl Pts',(1.41923722596421,-1.,-1.24824430986911));
#48075=CARTESIAN_POINT('Ctrl Pts',(1.41923722596421,1.,-1.24824430986911));
#48076=CARTESIAN_POINT('Ctrl Pts',(1.41422913175437,-1.,-1.24450600513278));
#48077=CARTESIAN_POINT('Ctrl Pts',(1.41422913175437,1.,-1.24450600513278));
#48078=CARTESIAN_POINT('Ctrl Pts',(1.40845295531151,-1.,-1.23994455029421));
#48079=CARTESIAN_POINT('Ctrl Pts',(1.40845295531151,1.,-1.23994455029421));
#48080=CARTESIAN_POINT('Ctrl Pts',(1.40164708205345,-1.,-1.23434087289768));
#48081=CARTESIAN_POINT('Ctrl Pts',(1.40164708205345,1.,-1.23434087289768));
#48082=CARTESIAN_POINT('Ctrl Pts',(1.39361389567257,-1.,-1.22752961898063));
#48083=CARTESIAN_POINT('Ctrl Pts',(1.39361389567257,1.,-1.22752961898063));
#48084=CARTESIAN_POINT('Ctrl Pts',(1.38420564525391,-1.,-1.21938737278853));
#48085=CARTESIAN_POINT('Ctrl Pts',(1.38420564525391,1.,-1.21938737278853));
#48086=CARTESIAN_POINT('Ctrl Pts',(1.37331915604962,-1.,-1.20982812923113));
#48087=CARTESIAN_POINT('Ctrl Pts',(1.37331915604962,1.,-1.20982812923113));
#48088=CARTESIAN_POINT('Ctrl Pts',(1.36088705040677,-1.,-1.1987959077656));
#48089=CARTESIAN_POINT('Ctrl Pts',(1.36088705040677,1.,-1.1987959077656));
#48090=CARTESIAN_POINT('Ctrl Pts',(1.34687053998157,-1.,-1.18625865664915));
#48091=CARTESIAN_POINT('Ctrl Pts',(1.34687053998157,1.,-1.18625865664915));
#48092=CARTESIAN_POINT('Ctrl Pts',(1.33437539344842,-1.,-1.17501305787994));
#48093=CARTESIAN_POINT('Ctrl Pts',(1.33437539344842,1.,-1.17501305787994));
#48094=CARTESIAN_POINT('Ctrl Pts',(1.32428080720544,-1.,-1.16589330092532));
#48095=CARTESIAN_POINT('Ctrl Pts',(1.32428080720544,1.,-1.16589330092532));
#48096=CARTESIAN_POINT('Ctrl Pts',(1.3172297721596,-1.,-1.15950888730433));
#48097=CARTESIAN_POINT('Ctrl Pts',(1.3172297721596,1.,-1.15950888730433));
#48098=CARTESIAN_POINT('Ctrl Pts',(1.31362392696032,-1.,-1.15624053661742));
#48099=CARTESIAN_POINT('Ctrl Pts',(1.31362392696032,1.,-1.15624053661742));
#48100=CARTESIAN_POINT('',(1.73811241238545,1.,-1.34869019493419));
#48101=CARTESIAN_POINT('Ctrl Pts',(1.73811241238545,1.,-1.34869019493419));
#48102=CARTESIAN_POINT('Ctrl Pts',(1.73682580585819,1.,-1.34854391898145));
#48103=CARTESIAN_POINT('Ctrl Pts',(1.73425417886254,1.,-1.34824783113158));
#48104=CARTESIAN_POINT('Ctrl Pts',(1.73040149654497,1.,-1.3477930915247));
#48105=CARTESIAN_POINT('Ctrl Pts',(1.72527410681298,1.,-1.34716554820013));
#48106=CARTESIAN_POINT('Ctrl Pts',(1.7188807715095,1.,-1.34634568653586));
#48107=CARTESIAN_POINT('Ctrl Pts',(1.71250340687011,1.,-1.34549029589563));
#48108=CARTESIAN_POINT('Ctrl Pts',(1.70614212266676,1.,-1.34459924533783));
#48109=CARTESIAN_POINT('Ctrl Pts',(1.69979707754221,1.,-1.34367237124322));
#48110=CARTESIAN_POINT('Ctrl Pts',(1.6934684849664,1.,-1.34270948206139));
#48111=CARTESIAN_POINT('Ctrl Pts',(1.68715660868602,1.,-1.34171037484673));
#48112=CARTESIAN_POINT('Ctrl Pts',(1.68086176030308,1.,-1.3406748518516));
#48113=CARTESIAN_POINT('Ctrl Pts',(1.67458429426126,1.,-1.33960273470372));
#48114=CARTESIAN_POINT('Ctrl Pts',(1.66832460784078,1.,-1.33849388654458));
#48115=CARTESIAN_POINT('Ctrl Pts',(1.66208312542073,1.,-1.33734820885331));
#48116=CARTESIAN_POINT('Ctrl Pts',(1.65586025952651,1.,-1.33616559745217));
#48117=CARTESIAN_POINT('Ctrl Pts',(1.64965637286843,1.,-1.33494590468003));
#48118=CARTESIAN_POINT('Ctrl Pts',(1.64347174856007,1.,-1.33368890676554));
#48119=CARTESIAN_POINT('Ctrl Pts',(1.63730653475049,1.,-1.33239425103694));
#48120=CARTESIAN_POINT('Ctrl Pts',(1.63116079730887,1.,-1.33106149345618));
#48121=CARTESIAN_POINT('Ctrl Pts',(1.62503464209777,1.,-1.32969019505665));
#48122=CARTESIAN_POINT('Ctrl Pts',(1.61892832270723,1.,-1.32828000610448));
#48123=CARTESIAN_POINT('Ctrl Pts',(1.61284234015762,1.,-1.32683074483365));
#48124=CARTESIAN_POINT('Ctrl Pts',(1.6067775829097,1.,-1.32534250785794));
#48125=CARTESIAN_POINT('Ctrl Pts',(1.600735118587,1.,-1.32381550858266));
#48126=CARTESIAN_POINT('Ctrl Pts',(1.59471591079408,1.,-1.32224985747686));
#48127=CARTESIAN_POINT('Ctrl Pts',(1.58872057258244,1.,-1.32064537110891));
#48128=CARTESIAN_POINT('Ctrl Pts',(1.58274907898829,1.,-1.31900135021428));
#48129=CARTESIAN_POINT('Ctrl Pts',(1.57680056505585,1.,-1.31731642317183));
#48130=CARTESIAN_POINT('Ctrl Pts',(1.57087397835721,1.,-1.31558903860015));
#48131=CARTESIAN_POINT('Ctrl Pts',(1.56496872402352,1.,-1.31381795281002));
#48132=CARTESIAN_POINT('Ctrl Pts',(1.55908521254822,1.,-1.31200264341696));
#48133=CARTESIAN_POINT('Ctrl Pts',(1.55322568759481,1.,-1.31014393684221));
#48134=CARTESIAN_POINT('Ctrl Pts',(1.54739413957183,1.,-1.30824393907471));
#48135=CARTESIAN_POINT('Ctrl Pts',(1.54159462645428,1.,-1.30630475189553));
#48136=CARTESIAN_POINT('Ctrl Pts',(1.53582981268976,1.,-1.30432735639487));
#48137=CARTESIAN_POINT('Ctrl Pts',(1.53009970283893,1.,-1.3023106439557));
#48138=CARTESIAN_POINT('Ctrl Pts',(1.5243995786107,1.,-1.30024984366334));
#48139=CARTESIAN_POINT('Ctrl Pts',(1.51872184912735,1.,-1.29813791800757));
#48140=CARTESIAN_POINT('Ctrl Pts',(1.51305994241412,1.,-1.29596850710518));
#48141=CARTESIAN_POINT('Ctrl Pts',(1.50741159078367,1.,-1.29373841372843));
#48142=CARTESIAN_POINT('Ctrl Pts',(1.50178230149764,1.,-1.29145022885171));
#48143=CARTESIAN_POINT('Ctrl Pts',(1.49618896881729,1.,-1.28911506584232));
#48144=CARTESIAN_POINT('Ctrl Pts',(1.4906522831275,1.,-1.28674676116415));
#48145=CARTESIAN_POINT('Ctrl Pts',(1.48518817118891,1.,-1.28435533880184));
#48146=CARTESIAN_POINT('Ctrl Pts',(1.47980070347102,1.,-1.28194158939522));
#48147=CARTESIAN_POINT('Ctrl Pts',(1.4744717526711,1.,-1.27948918248524));
#48148=CARTESIAN_POINT('Ctrl Pts',(1.46916035917197,1.,-1.27696414831144));
#48149=CARTESIAN_POINT('Ctrl Pts',(1.4638243133254,1.,-1.27433119897877));
#48150=CARTESIAN_POINT('Ctrl Pts',(1.45843906294725,1.,-1.27156805265312));
#48151=CARTESIAN_POINT('Ctrl Pts',(1.45301422764205,1.,-1.26867786804854));
#48152=CARTESIAN_POINT('Ctrl Pts',(1.44761985001544,1.,-1.26570925118767));
#48153=CARTESIAN_POINT('Ctrl Pts',(1.44236470511145,1.,-1.26273903323723));
#48154=CARTESIAN_POINT('Ctrl Pts',(1.43734919180719,1.,-1.25983531011894));
#48155=CARTESIAN_POINT('Ctrl Pts',(1.43262645609679,1.,-1.25702687965744));
#48156=CARTESIAN_POINT('Ctrl Pts',(1.42815938799555,1.,-1.25426945222783));
#48157=CARTESIAN_POINT('Ctrl Pts',(1.42378102115911,1.,-1.25141455570299));
#48158=CARTESIAN_POINT('Ctrl Pts',(1.41923722596421,1.,-1.24824430986911));
#48159=CARTESIAN_POINT('Ctrl Pts',(1.41422913175437,1.,-1.24450600513278));
#48160=CARTESIAN_POINT('Ctrl Pts',(1.40845295531151,1.,-1.23994455029421));
#48161=CARTESIAN_POINT('Ctrl Pts',(1.40164708205345,1.,-1.23434087289768));
#48162=CARTESIAN_POINT('Ctrl Pts',(1.39361389567257,1.,-1.22752961898063));
#48163=CARTESIAN_POINT('Ctrl Pts',(1.38420564525391,1.,-1.21938737278853));
#48164=CARTESIAN_POINT('Ctrl Pts',(1.37331915604962,1.,-1.20982812923113));
#48165=CARTESIAN_POINT('Ctrl Pts',(1.36088705040677,1.,-1.1987959077656));
#48166=CARTESIAN_POINT('Ctrl Pts',(1.34687053998157,1.,-1.18625865664915));
#48167=CARTESIAN_POINT('Ctrl Pts',(1.33437539344842,1.,-1.17501305787994));
#48168=CARTESIAN_POINT('Ctrl Pts',(1.32428080720544,1.,-1.16589330092532));
#48169=CARTESIAN_POINT('Ctrl Pts',(1.3172297721596,1.,-1.15950888730433));
#48170=CARTESIAN_POINT('Ctrl Pts',(1.31362392696032,1.,-1.15624053661742));
#48171=CARTESIAN_POINT('',(1.73811241238545,0.,-1.34869019493419));
#48172=CARTESIAN_POINT('Origin',(1.81978687191668,0.,-1.23627494547115));
#48173=CARTESIAN_POINT('',(1.81978687191668,1.,-1.23627494547115));
#48174=CARTESIAN_POINT('',(1.73811241238545,1.,-1.34869019493419));
#48175=CARTESIAN_POINT('',(1.81978687191668,0.,-1.23627494547115));
#48176=CARTESIAN_POINT('Ctrl Pts',(1.5055822144029,-1.,-0.892032620296855));
#48177=CARTESIAN_POINT('Ctrl Pts',(1.5055822144029,1.,-0.892032620296855));
#48178=CARTESIAN_POINT('Ctrl Pts',(1.50980486807181,-1.,-0.894452006967538));
#48179=CARTESIAN_POINT('Ctrl Pts',(1.50980486807181,1.,-0.894452006967538));
#48180=CARTESIAN_POINT('Ctrl Pts',(1.51805569591479,-1.,-0.89918504749193));
#48181=CARTESIAN_POINT('Ctrl Pts',(1.51805569591479,1.,-0.89918504749193));
#48182=CARTESIAN_POINT('Ctrl Pts',(1.52984849890434,-1.,-0.905967409640499));
#48183=CARTESIAN_POINT('Ctrl Pts',(1.52984849890434,1.,-0.905967409640499));
#48184=CARTESIAN_POINT('Ctrl Pts',(1.54440491152807,-1.,-0.91437591904658));
#48185=CARTESIAN_POINT('Ctrl Pts',(1.54440491152807,1.,-0.91437591904658));
#48186=CARTESIAN_POINT('Ctrl Pts',(1.56065988582509,-1.,-0.923832188966322));
#48187=CARTESIAN_POINT('Ctrl Pts',(1.56065988582509,1.,-0.923832188966322));
#48188=CARTESIAN_POINT('Ctrl Pts',(1.57499388385561,-1.,-0.932246680128849));
#48189=CARTESIAN_POINT('Ctrl Pts',(1.57499388385561,1.,-0.932246680128849));
#48190=CARTESIAN_POINT('Ctrl Pts',(1.58744937489796,-1.,-0.939646377909319));
#48191=CARTESIAN_POINT('Ctrl Pts',(1.58744937489796,1.,-0.939646377909319));
#48192=CARTESIAN_POINT('Ctrl Pts',(1.59810042045408,-1.,-0.946078063325796));
#48193=CARTESIAN_POINT('Ctrl Pts',(1.59810042045408,1.,-0.946078063325796));
#48194=CARTESIAN_POINT('Ctrl Pts',(1.60706069897794,-1.,-0.951613284361248));
#48195=CARTESIAN_POINT('Ctrl Pts',(1.60706069897794,1.,-0.951613284361248));
#48196=CARTESIAN_POINT('Ctrl Pts',(1.61449324337233,-1.,-0.956354422921573));
#48197=CARTESIAN_POINT('Ctrl Pts',(1.61449324337233,1.,-0.956354422921573));
#48198=CARTESIAN_POINT('Ctrl Pts',(1.62061638139929,-1.,-0.960438326099958));
#48199=CARTESIAN_POINT('Ctrl Pts',(1.62061638139929,1.,-0.960438326099958));
#48200=CARTESIAN_POINT('Ctrl Pts',(1.6257193066974,-1.,-0.964046107037821));
#48201=CARTESIAN_POINT('Ctrl Pts',(1.6257193066974,1.,-0.964046107037821));
#48202=CARTESIAN_POINT('Ctrl Pts',(1.63013849959083,-1.,-0.967387853228041));
#48203=CARTESIAN_POINT('Ctrl Pts',(1.63013849959083,1.,-0.967387853228041));
#48204=CARTESIAN_POINT('Ctrl Pts',(1.63420665729609,-1.,-0.970669715996356));
#48205=CARTESIAN_POINT('Ctrl Pts',(1.63420665729609,1.,-0.970669715996356));
#48206=CARTESIAN_POINT('Ctrl Pts',(1.63820952658157,-1.,-0.974066058287501));
#48207=CARTESIAN_POINT('Ctrl Pts',(1.63820952658157,1.,-0.974066058287501));
#48208=CARTESIAN_POINT('Ctrl Pts',(1.64233990826831,-1.,-0.977689794120297));
#48209=CARTESIAN_POINT('Ctrl Pts',(1.64233990826831,1.,-0.977689794120297));
#48210=CARTESIAN_POINT('Ctrl Pts',(1.64665139190834,-1.,-0.981562530940574));
#48211=CARTESIAN_POINT('Ctrl Pts',(1.64665139190834,1.,-0.981562530940574));
#48212=CARTESIAN_POINT('Ctrl Pts',(1.6511001661277,-1.,-0.985642622921626));
#48213=CARTESIAN_POINT('Ctrl Pts',(1.6511001661277,1.,-0.985642622921626));
#48214=CARTESIAN_POINT('Ctrl Pts',(1.65559044289746,-1.,-0.98985562785445));
#48215=CARTESIAN_POINT('Ctrl Pts',(1.65559044289746,1.,-0.98985562785445));
#48216=CARTESIAN_POINT('Ctrl Pts',(1.66001553809916,-1.,-0.994121836661116));
#48217=CARTESIAN_POINT('Ctrl Pts',(1.66001553809916,1.,-0.994121836661116));
#48218=CARTESIAN_POINT('Ctrl Pts',(1.66430758030304,-1.,-0.998389654952317));
#48219=CARTESIAN_POINT('Ctrl Pts',(1.66430758030304,1.,-0.998389654952317));
#48220=CARTESIAN_POINT('Ctrl Pts',(1.66846059277231,-1.,-1.00265091003682));
#48221=CARTESIAN_POINT('Ctrl Pts',(1.66846059277231,1.,-1.00265091003682));
#48222=CARTESIAN_POINT('Ctrl Pts',(1.67250335383248,-1.,-1.00692206696387));
#48223=CARTESIAN_POINT('Ctrl Pts',(1.67250335383248,1.,-1.00692206696387));
#48224=CARTESIAN_POINT('Ctrl Pts',(1.67648246776457,-1.,-1.01123236493507));
#48225=CARTESIAN_POINT('Ctrl Pts',(1.67648246776457,1.,-1.01123236493507));
#48226=CARTESIAN_POINT('Ctrl Pts',(1.6804428989482,-1.,-1.01561026162787));
#48227=CARTESIAN_POINT('Ctrl Pts',(1.6804428989482,1.,-1.01561026162787));
#48228=CARTESIAN_POINT('Ctrl Pts',(1.68440578021739,-1.,-1.02006795074222));
#48229=CARTESIAN_POINT('Ctrl Pts',(1.68440578021739,1.,-1.02006795074222));
#48230=CARTESIAN_POINT('Ctrl Pts',(1.68836910178475,-1.,-1.02460180535272));
#48231=CARTESIAN_POINT('Ctrl Pts',(1.68836910178475,1.,-1.02460180535272));
#48232=CARTESIAN_POINT('Ctrl Pts',(1.69231840863471,-1.,-1.02919977579155));
#48233=CARTESIAN_POINT('Ctrl Pts',(1.69231840863471,1.,-1.02919977579155));
#48234=CARTESIAN_POINT('Ctrl Pts',(1.69623414782769,-1.,-1.03384646003587));
#48235=CARTESIAN_POINT('Ctrl Pts',(1.69623414782769,1.,-1.03384646003587));
#48236=CARTESIAN_POINT('Ctrl Pts',(1.70010052930951,-1.,-1.03852922490782));
#48237=CARTESIAN_POINT('Ctrl Pts',(1.70010052930951,1.,-1.03852922490782));
#48238=CARTESIAN_POINT('Ctrl Pts',(1.70391338707969,-1.,-1.04324363334546));
#48239=CARTESIAN_POINT('Ctrl Pts',(1.70391338707969,1.,-1.04324363334546));
#48240=CARTESIAN_POINT('Ctrl Pts',(1.70767646263641,-1.,-1.0479908540499));
#48241=CARTESIAN_POINT('Ctrl Pts',(1.70767646263641,1.,-1.0479908540499));
#48242=CARTESIAN_POINT('Ctrl Pts',(1.71139783543986,-1.,-1.05277517202854));
#48243=CARTESIAN_POINT('Ctrl Pts',(1.71139783543986,1.,-1.05277517202854));
#48244=CARTESIAN_POINT('Ctrl Pts',(1.71508654427022,-1.,-1.05760163192481));
#48245=CARTESIAN_POINT('Ctrl Pts',(1.71508654427022,1.,-1.05760163192481));
#48246=CARTESIAN_POINT('Ctrl Pts',(1.71874858456908,-1.,-1.0624732468065));
#48247=CARTESIAN_POINT('Ctrl Pts',(1.71874858456908,1.,-1.0624732468065));
#48248=CARTESIAN_POINT('Ctrl Pts',(1.72238500928456,-1.,-1.06738966975463));
#48249=CARTESIAN_POINT('Ctrl Pts',(1.72238500928456,1.,-1.06738966975463));
#48250=CARTESIAN_POINT('Ctrl Pts',(1.72599406198489,-1.,-1.07234866990252));
#48251=CARTESIAN_POINT('Ctrl Pts',(1.72599406198489,1.,-1.07234866990252));
#48252=CARTESIAN_POINT('Ctrl Pts',(1.72957248977424,-1.,-1.0773470373727));
#48253=CARTESIAN_POINT('Ctrl Pts',(1.72957248977424,1.,-1.0773470373727));
#48254=CARTESIAN_POINT('Ctrl Pts',(1.73311705663407,-1.,-1.08238162784749));
#48255=CARTESIAN_POINT('Ctrl Pts',(1.73311705663407,1.,-1.08238162784749));
#48256=CARTESIAN_POINT('Ctrl Pts',(1.73662628326093,-1.,-1.08745056285429));
#48257=CARTESIAN_POINT('Ctrl Pts',(1.73662628326093,1.,-1.08745056285429));
#48258=CARTESIAN_POINT('Ctrl Pts',(1.74010053962252,-1.,-1.09255329056496));
#48259=CARTESIAN_POINT('Ctrl Pts',(1.74010053962252,1.,-1.09255329056496));
#48260=CARTESIAN_POINT('Ctrl Pts',(1.74354119236212,-1.,-1.09768999241229));
#48261=CARTESIAN_POINT('Ctrl Pts',(1.74354119236212,1.,-1.09768999241229));
#48262=CARTESIAN_POINT('Ctrl Pts',(1.74695004214924,-1.,-1.10286118991144));
#48263=CARTESIAN_POINT('Ctrl Pts',(1.74695004214924,1.,-1.10286118991144));
#48264=CARTESIAN_POINT('Ctrl Pts',(1.75032866075914,-1.,-1.10806728183003));
#48265=CARTESIAN_POINT('Ctrl Pts',(1.75032866075914,1.,-1.10806728183003));
#48266=CARTESIAN_POINT('Ctrl Pts',(1.75367772094617,-1.,-1.11330807582542));
#48267=CARTESIAN_POINT('Ctrl Pts',(1.75367772094617,1.,-1.11330807582542));
#48268=CARTESIAN_POINT('Ctrl Pts',(1.75699720772089,-1.,-1.11858293216752));
#48269=CARTESIAN_POINT('Ctrl Pts',(1.75699720772089,1.,-1.11858293216752));
#48270=CARTESIAN_POINT('Ctrl Pts',(1.76028671825084,-1.,-1.12389096855078));
#48271=CARTESIAN_POINT('Ctrl Pts',(1.76028671825084,1.,-1.12389096855078));
#48272=CARTESIAN_POINT('Ctrl Pts',(1.76354571966171,-1.,-1.12923123555076));
#48273=CARTESIAN_POINT('Ctrl Pts',(1.76354571966171,1.,-1.12923123555076));
#48274=CARTESIAN_POINT('Ctrl Pts',(1.76677384551883,-1.,-1.13460291804635));
#48275=CARTESIAN_POINT('Ctrl Pts',(1.76677384551883,1.,-1.13460291804635));
#48276=CARTESIAN_POINT('Ctrl Pts',(1.76997111386806,-1.,-1.14000548337));
#48277=CARTESIAN_POINT('Ctrl Pts',(1.76997111386806,1.,-1.14000548337));
#48278=CARTESIAN_POINT('Ctrl Pts',(1.77313777896234,-1.,-1.14543858226948));
#48279=CARTESIAN_POINT('Ctrl Pts',(1.77313777896234,1.,-1.14543858226948));
#48280=CARTESIAN_POINT('Ctrl Pts',(1.77627422557034,-1.,-1.15090197841531));
#48281=CARTESIAN_POINT('Ctrl Pts',(1.77627422557034,1.,-1.15090197841531));
#48282=CARTESIAN_POINT('Ctrl Pts',(1.77938085564261,-1.,-1.15639547194689));
#48283=CARTESIAN_POINT('Ctrl Pts',(1.77938085564261,1.,-1.15639547194689));
#48284=CARTESIAN_POINT('Ctrl Pts',(1.78245795880949,-1.,-1.16191881298458));
#48285=CARTESIAN_POINT('Ctrl Pts',(1.78245795880949,1.,-1.16191881298458));
#48286=CARTESIAN_POINT('Ctrl Pts',(1.78550566040349,-1.,-1.16747166312239));
#48287=CARTESIAN_POINT('Ctrl Pts',(1.78550566040349,1.,-1.16747166312239));
#48288=CARTESIAN_POINT('Ctrl Pts',(1.78852398877523,-1.,-1.17305363177265));
#48289=CARTESIAN_POINT('Ctrl Pts',(1.78852398877523,1.,-1.17305363177265));
#48290=CARTESIAN_POINT('Ctrl Pts',(1.79151291552646,-1.,-1.17866429440781));
#48291=CARTESIAN_POINT('Ctrl Pts',(1.79151291552646,1.,-1.17866429440781));
#48292=CARTESIAN_POINT('Ctrl Pts',(1.79447240321572,-1.,-1.18430321697471));
#48293=CARTESIAN_POINT('Ctrl Pts',(1.79447240321572,1.,-1.18430321697471));
#48294=CARTESIAN_POINT('Ctrl Pts',(1.79740245923649,-1.,-1.1899699793456));
#48295=CARTESIAN_POINT('Ctrl Pts',(1.79740245923649,1.,-1.1899699793456));
#48296=CARTESIAN_POINT('Ctrl Pts',(1.80030314370121,-1.,-1.19566418930405));
#48297=CARTESIAN_POINT('Ctrl Pts',(1.80030314370121,1.,-1.19566418930405));
#48298=CARTESIAN_POINT('Ctrl Pts',(1.8031745483882,-1.,-1.2013854893912));
#48299=CARTESIAN_POINT('Ctrl Pts',(1.8031745483882,1.,-1.2013854893912));
#48300=CARTESIAN_POINT('Ctrl Pts',(1.80601678480772,-1.,-1.20713356605519));
#48301=CARTESIAN_POINT('Ctrl Pts',(1.80601678480772,1.,-1.20713356605519));
#48302=CARTESIAN_POINT('Ctrl Pts',(1.80882996916931,-1.,-1.2129081570818));
#48303=CARTESIAN_POINT('Ctrl Pts',(1.80882996916931,1.,-1.2129081570818));
#48304=CARTESIAN_POINT('Ctrl Pts',(1.81161420806172,-1.,-1.2187090610323));
#48305=CARTESIAN_POINT('Ctrl Pts',(1.81161420806172,1.,-1.2187090610323));
#48306=CARTESIAN_POINT('Ctrl Pts',(1.81436959209778,-1.,-1.22453613304507));
#48307=CARTESIAN_POINT('Ctrl Pts',(1.81436959209778,1.,-1.22453613304507));
#48308=CARTESIAN_POINT('Ctrl Pts',(1.81655087183054,-1.,-1.22921864890975));
#48309=CARTESIAN_POINT('Ctrl Pts',(1.81655087183054,1.,-1.22921864890975));
#48310=CARTESIAN_POINT('Ctrl Pts',(1.81817389920914,-1.,-1.23274224526804));
#48311=CARTESIAN_POINT('Ctrl Pts',(1.81817389920914,1.,-1.23274224526804));
#48312=CARTESIAN_POINT('Ctrl Pts',(1.81925017193531,-1.,-1.23509651170384));
#48313=CARTESIAN_POINT('Ctrl Pts',(1.81925017193531,1.,-1.23509651170384));
#48314=CARTESIAN_POINT('Ctrl Pts',(1.81978687191668,-1.,-1.23627494547115));
#48315=CARTESIAN_POINT('Ctrl Pts',(1.81978687191668,1.,-1.23627494547115));
#48316=CARTESIAN_POINT('',(1.5055822144029,1.,-0.892032620296855));
#48317=CARTESIAN_POINT('Ctrl Pts',(1.5055822144029,1.,-0.892032620296855));
#48318=CARTESIAN_POINT('Ctrl Pts',(1.50980486807181,1.,-0.894452006967538));
#48319=CARTESIAN_POINT('Ctrl Pts',(1.51805569591479,1.,-0.89918504749193));
#48320=CARTESIAN_POINT('Ctrl Pts',(1.52984849890434,1.,-0.905967409640499));
#48321=CARTESIAN_POINT('Ctrl Pts',(1.54440491152807,1.,-0.91437591904658));
#48322=CARTESIAN_POINT('Ctrl Pts',(1.56065988582509,1.,-0.923832188966322));
#48323=CARTESIAN_POINT('Ctrl Pts',(1.57499388385561,1.,-0.932246680128849));
#48324=CARTESIAN_POINT('Ctrl Pts',(1.58744937489796,1.,-0.939646377909319));
#48325=CARTESIAN_POINT('Ctrl Pts',(1.59810042045408,1.,-0.946078063325796));
#48326=CARTESIAN_POINT('Ctrl Pts',(1.60706069897794,1.,-0.951613284361248));
#48327=CARTESIAN_POINT('Ctrl Pts',(1.61449324337233,1.,-0.956354422921573));
#48328=CARTESIAN_POINT('Ctrl Pts',(1.62061638139929,1.,-0.960438326099958));
#48329=CARTESIAN_POINT('Ctrl Pts',(1.6257193066974,1.,-0.964046107037821));
#48330=CARTESIAN_POINT('Ctrl Pts',(1.63013849959083,1.,-0.967387853228041));
#48331=CARTESIAN_POINT('Ctrl Pts',(1.63420665729609,1.,-0.970669715996356));
#48332=CARTESIAN_POINT('Ctrl Pts',(1.63820952658157,1.,-0.974066058287501));
#48333=CARTESIAN_POINT('Ctrl Pts',(1.64233990826831,1.,-0.977689794120297));
#48334=CARTESIAN_POINT('Ctrl Pts',(1.64665139190834,1.,-0.981562530940574));
#48335=CARTESIAN_POINT('Ctrl Pts',(1.6511001661277,1.,-0.985642622921626));
#48336=CARTESIAN_POINT('Ctrl Pts',(1.65559044289746,1.,-0.98985562785445));
#48337=CARTESIAN_POINT('Ctrl Pts',(1.66001553809916,1.,-0.994121836661116));
#48338=CARTESIAN_POINT('Ctrl Pts',(1.66430758030304,1.,-0.998389654952317));
#48339=CARTESIAN_POINT('Ctrl Pts',(1.66846059277231,1.,-1.00265091003682));
#48340=CARTESIAN_POINT('Ctrl Pts',(1.67250335383248,1.,-1.00692206696387));
#48341=CARTESIAN_POINT('Ctrl Pts',(1.67648246776457,1.,-1.01123236493507));
#48342=CARTESIAN_POINT('Ctrl Pts',(1.6804428989482,1.,-1.01561026162787));
#48343=CARTESIAN_POINT('Ctrl Pts',(1.68440578021739,1.,-1.02006795074222));
#48344=CARTESIAN_POINT('Ctrl Pts',(1.68836910178475,1.,-1.02460180535272));
#48345=CARTESIAN_POINT('Ctrl Pts',(1.69231840863471,1.,-1.02919977579155));
#48346=CARTESIAN_POINT('Ctrl Pts',(1.69623414782769,1.,-1.03384646003587));
#48347=CARTESIAN_POINT('Ctrl Pts',(1.70010052930951,1.,-1.03852922490782));
#48348=CARTESIAN_POINT('Ctrl Pts',(1.70391338707969,1.,-1.04324363334546));
#48349=CARTESIAN_POINT('Ctrl Pts',(1.70767646263641,1.,-1.0479908540499));
#48350=CARTESIAN_POINT('Ctrl Pts',(1.71139783543986,1.,-1.05277517202854));
#48351=CARTESIAN_POINT('Ctrl Pts',(1.71508654427022,1.,-1.05760163192481));
#48352=CARTESIAN_POINT('Ctrl Pts',(1.71874858456908,1.,-1.0624732468065));
#48353=CARTESIAN_POINT('Ctrl Pts',(1.72238500928456,1.,-1.06738966975463));
#48354=CARTESIAN_POINT('Ctrl Pts',(1.72599406198489,1.,-1.07234866990252));
#48355=CARTESIAN_POINT('Ctrl Pts',(1.72957248977424,1.,-1.0773470373727));
#48356=CARTESIAN_POINT('Ctrl Pts',(1.73311705663407,1.,-1.08238162784749));
#48357=CARTESIAN_POINT('Ctrl Pts',(1.73662628326093,1.,-1.08745056285429));
#48358=CARTESIAN_POINT('Ctrl Pts',(1.74010053962252,1.,-1.09255329056496));
#48359=CARTESIAN_POINT('Ctrl Pts',(1.74354119236212,1.,-1.09768999241229));
#48360=CARTESIAN_POINT('Ctrl Pts',(1.74695004214924,1.,-1.10286118991144));
#48361=CARTESIAN_POINT('Ctrl Pts',(1.75032866075914,1.,-1.10806728183003));
#48362=CARTESIAN_POINT('Ctrl Pts',(1.75367772094617,1.,-1.11330807582542));
#48363=CARTESIAN_POINT('Ctrl Pts',(1.75699720772089,1.,-1.11858293216752));
#48364=CARTESIAN_POINT('Ctrl Pts',(1.76028671825084,1.,-1.12389096855078));
#48365=CARTESIAN_POINT('Ctrl Pts',(1.76354571966171,1.,-1.12923123555076));
#48366=CARTESIAN_POINT('Ctrl Pts',(1.76677384551883,1.,-1.13460291804635));
#48367=CARTESIAN_POINT('Ctrl Pts',(1.76997111386806,1.,-1.14000548337));
#48368=CARTESIAN_POINT('Ctrl Pts',(1.77313777896234,1.,-1.14543858226948));
#48369=CARTESIAN_POINT('Ctrl Pts',(1.77627422557034,1.,-1.15090197841531));
#48370=CARTESIAN_POINT('Ctrl Pts',(1.77938085564261,1.,-1.15639547194689));
#48371=CARTESIAN_POINT('Ctrl Pts',(1.78245795880949,1.,-1.16191881298458));
#48372=CARTESIAN_POINT('Ctrl Pts',(1.78550566040349,1.,-1.16747166312239));
#48373=CARTESIAN_POINT('Ctrl Pts',(1.78852398877523,1.,-1.17305363177265));
#48374=CARTESIAN_POINT('Ctrl Pts',(1.79151291552646,1.,-1.17866429440781));
#48375=CARTESIAN_POINT('Ctrl Pts',(1.79447240321572,1.,-1.18430321697471));
#48376=CARTESIAN_POINT('Ctrl Pts',(1.79740245923649,1.,-1.1899699793456));
#48377=CARTESIAN_POINT('Ctrl Pts',(1.80030314370121,1.,-1.19566418930405));
#48378=CARTESIAN_POINT('Ctrl Pts',(1.8031745483882,1.,-1.2013854893912));
#48379=CARTESIAN_POINT('Ctrl Pts',(1.80601678480772,1.,-1.20713356605519));
#48380=CARTESIAN_POINT('Ctrl Pts',(1.80882996916931,1.,-1.2129081570818));
#48381=CARTESIAN_POINT('Ctrl Pts',(1.81161420806172,1.,-1.2187090610323));
#48382=CARTESIAN_POINT('Ctrl Pts',(1.81436959209778,1.,-1.22453613304507));
#48383=CARTESIAN_POINT('Ctrl Pts',(1.81655087183054,1.,-1.22921864890975));
#48384=CARTESIAN_POINT('Ctrl Pts',(1.81817389920914,1.,-1.23274224526804));
#48385=CARTESIAN_POINT('Ctrl Pts',(1.81925017193531,1.,-1.23509651170384));
#48386=CARTESIAN_POINT('Ctrl Pts',(1.81978687191668,1.,-1.23627494547115));
#48387=CARTESIAN_POINT('',(1.5055822144029,0.,-0.892032620296855));
#48388=CARTESIAN_POINT('Origin',(0.,0.,0.));
#48389=CARTESIAN_POINT('',(1.60662857109684,1.,-0.693717979106306));
#48390=CARTESIAN_POINT('Origin',(0.,1.,0.));
#48391=CARTESIAN_POINT('',(1.60662857109684,0.,-0.693717979106308));
#48392=CARTESIAN_POINT('Ctrl Pts',(2.0698113262342,-1.,-0.745574324794401));
#48393=CARTESIAN_POINT('Ctrl Pts',(2.0698113262342,1.,-0.745574324794401));
#48394=CARTESIAN_POINT('Ctrl Pts',(2.06854248895728,-1.,-0.745832791378367));
#48395=CARTESIAN_POINT('Ctrl Pts',(2.06854248895728,1.,-0.745832791378367));
#48396=CARTESIAN_POINT('Ctrl Pts',(2.06600523016815,-1.,-0.746345871544201));
#48397=CARTESIAN_POINT('Ctrl Pts',(2.06600523016815,1.,-0.746345871544201));
#48398=CARTESIAN_POINT('Ctrl Pts',(2.06220058927826,-1.,-0.74710393278792));
#48399=CARTESIAN_POINT('Ctrl Pts',(2.06220058927826,1.,-0.74710393278792));
#48400=CARTESIAN_POINT('Ctrl Pts',(2.05713023031006,-1.,-0.748091554183803));
#48401=CARTESIAN_POINT('Ctrl Pts',(2.05713023031006,1.,-0.748091554183803));
#48402=CARTESIAN_POINT('Ctrl Pts',(2.05079645592154,-1.,-0.749287468665046));
#48403=CARTESIAN_POINT('Ctrl Pts',(2.05079645592154,1.,-0.749287468665046));
#48404=CARTESIAN_POINT('Ctrl Pts',(2.04446689147979,-1.,-0.750444657875576));
#48405=CARTESIAN_POINT('Ctrl Pts',(2.04446689147979,1.,-0.750444657875576));
#48406=CARTESIAN_POINT('Ctrl Pts',(2.03814160092099,-1.,-0.751562963361115));
#48407=CARTESIAN_POINT('Ctrl Pts',(2.03814160092099,1.,-0.751562963361115));
#48408=CARTESIAN_POINT('Ctrl Pts',(2.03182068456221,-1.,-0.752642180487211));
#48409=CARTESIAN_POINT('Ctrl Pts',(2.03182068456221,1.,-0.752642180487211));
#48410=CARTESIAN_POINT('Ctrl Pts',(2.02550428623313,-1.,-0.753682061112768));
#48411=CARTESIAN_POINT('Ctrl Pts',(2.02550428623313,1.,-0.753682061112768));
#48412=CARTESIAN_POINT('Ctrl Pts',(2.01919259405809,-1.,-0.754682330722816));
#48413=CARTESIAN_POINT('Ctrl Pts',(2.01919259405809,1.,-0.754682330722816));
#48414=CARTESIAN_POINT('Ctrl Pts',(2.01288584328084,-1.,-0.755642704957865));
#48415=CARTESIAN_POINT('Ctrl Pts',(2.01288584328084,1.,-0.755642704957865));
#48416=CARTESIAN_POINT('Ctrl Pts',(2.0065843158773,-1.,-0.756562904646671));
#48417=CARTESIAN_POINT('Ctrl Pts',(2.0065843158773,1.,-0.756562904646671));
#48418=CARTESIAN_POINT('Ctrl Pts',(2.00028834739178,-1.,-0.757442676862724));
#48419=CARTESIAN_POINT('Ctrl Pts',(2.00028834739178,1.,-0.757442676862724));
#48420=CARTESIAN_POINT('Ctrl Pts',(1.99399831098817,-1.,-0.758281796766761));
#48421=CARTESIAN_POINT('Ctrl Pts',(1.99399831098817,1.,-0.758281796766761));
#48422=CARTESIAN_POINT('Ctrl Pts',(1.98771456680874,-1.,-0.759080037802488));
#48423=CARTESIAN_POINT('Ctrl Pts',(1.98771456680874,1.,-0.759080037802488));
#48424=CARTESIAN_POINT('Ctrl Pts',(1.98143741418172,-1.,-0.75983714745219));
#48425=CARTESIAN_POINT('Ctrl Pts',(1.98143741418172,1.,-0.75983714745219));
#48426=CARTESIAN_POINT('Ctrl Pts',(1.97516705321494,-1.,-0.760552825409757));
#48427=CARTESIAN_POINT('Ctrl Pts',(1.97516705321494,1.,-0.760552825409757));
#48428=CARTESIAN_POINT('Ctrl Pts',(1.96890351582499,-1.,-0.761226690483821));
#48429=CARTESIAN_POINT('Ctrl Pts',(1.96890351582499,1.,-0.761226690483821));
#48430=CARTESIAN_POINT('Ctrl Pts',(1.96264672744186,-1.,-0.761858300014424));
#48431=CARTESIAN_POINT('Ctrl Pts',(1.96264672744186,1.,-0.761858300014424));
#48432=CARTESIAN_POINT('Ctrl Pts',(1.95639665309869,-1.,-0.762447203806179));
#48433=CARTESIAN_POINT('Ctrl Pts',(1.95639665309869,1.,-0.762447203806179));
#48434=CARTESIAN_POINT('Ctrl Pts',(1.95015342590024,-1.,-0.762992990878769));
#48435=CARTESIAN_POINT('Ctrl Pts',(1.95015342590024,1.,-0.762992990878769));
#48436=CARTESIAN_POINT('Ctrl Pts',(1.9439174661764,-1.,-0.763495333538629));
#48437=CARTESIAN_POINT('Ctrl Pts',(1.9439174661764,1.,-0.763495333538629));
#48438=CARTESIAN_POINT('Ctrl Pts',(1.93768964875886,-1.,-0.763954049121459));
#48439=CARTESIAN_POINT('Ctrl Pts',(1.93768964875886,1.,-0.763954049121459));
#48440=CARTESIAN_POINT('Ctrl Pts',(1.93147105496382,-1.,-0.764369010673941));
#48441=CARTESIAN_POINT('Ctrl Pts',(1.93147105496382,1.,-0.764369010673941));
#48442=CARTESIAN_POINT('Ctrl Pts',(1.92526263537048,-1.,-0.764740025488212));
#48443=CARTESIAN_POINT('Ctrl Pts',(1.92526263537048,1.,-0.764740025488212));
#48444=CARTESIAN_POINT('Ctrl Pts',(1.91906491634196,-1.,-0.765066729667089));
#48445=CARTESIAN_POINT('Ctrl Pts',(1.91906491634196,1.,-0.765066729667089));
#48446=CARTESIAN_POINT('Ctrl Pts',(1.91287765805169,-1.,-0.765348465884722));
#48447=CARTESIAN_POINT('Ctrl Pts',(1.91287765805169,1.,-0.765348465884722));
#48448=CARTESIAN_POINT('Ctrl Pts',(1.90669961402356,-1.,-0.765584196937919));
#48449=CARTESIAN_POINT('Ctrl Pts',(1.90669961402356,1.,-0.765584196937919));
#48450=CARTESIAN_POINT('Ctrl Pts',(1.90052930393596,-1.,-0.765772772593386));
#48451=CARTESIAN_POINT('Ctrl Pts',(1.90052930393596,1.,-0.765772772593386));
#48452=CARTESIAN_POINT('Ctrl Pts',(1.89436577771388,-1.,-0.765913193856978));
#48453=CARTESIAN_POINT('Ctrl Pts',(1.89436577771388,1.,-0.765913193856978));
#48454=CARTESIAN_POINT('Ctrl Pts',(1.88820926433409,-1.,-0.766004837062091));
#48455=CARTESIAN_POINT('Ctrl Pts',(1.88820926433409,1.,-0.766004837062091));
#48456=CARTESIAN_POINT('Ctrl Pts',(1.88206215302561,-1.,-0.766047794851865));
#48457=CARTESIAN_POINT('Ctrl Pts',(1.88206215302561,1.,-0.766047794851865));
#48458=CARTESIAN_POINT('Ctrl Pts',(1.87592888967883,-1.,-0.766042837036744));
#48459=CARTESIAN_POINT('Ctrl Pts',(1.87592888967883,1.,-0.766042837036744));
#48460=CARTESIAN_POINT('Ctrl Pts',(1.86981398314341,-1.,-0.765990708546091));
#48461=CARTESIAN_POINT('Ctrl Pts',(1.86981398314341,1.,-0.765990708546091));
#48462=CARTESIAN_POINT('Ctrl Pts',(1.86372027063312,-1.,-0.765891519092547));
#48463=CARTESIAN_POINT('Ctrl Pts',(1.86372027063312,1.,-0.765891519092547));
#48464=CARTESIAN_POINT('Ctrl Pts',(1.85764741390394,-1.,-0.765744212909319));
#48465=CARTESIAN_POINT('Ctrl Pts',(1.85764741390394,1.,-0.765744212909319));
#48466=CARTESIAN_POINT('Ctrl Pts',(1.85158945130063,-1.,-0.765545710619063));
#48467=CARTESIAN_POINT('Ctrl Pts',(1.85158945130063,1.,-0.765545710619063));
#48468=CARTESIAN_POINT('Ctrl Pts',(1.84553698875924,-1.,-0.765291664862029));
#48469=CARTESIAN_POINT('Ctrl Pts',(1.84553698875924,1.,-0.765291664862029));
#48470=CARTESIAN_POINT('Ctrl Pts',(1.83948181064835,-1.,-0.764978057881738));
#48471=CARTESIAN_POINT('Ctrl Pts',(1.83948181064835,1.,-0.764978057881738));
#48472=CARTESIAN_POINT('Ctrl Pts',(1.83342077227142,-1.,-0.764602549687853));
#48473=CARTESIAN_POINT('Ctrl Pts',(1.83342077227142,1.,-0.764602549687853));
#48474=CARTESIAN_POINT('Ctrl Pts',(1.82735991200065,-1.,-0.764165902605995));
#48475=CARTESIAN_POINT('Ctrl Pts',(1.82735991200065,1.,-0.764165902605995));
#48476=CARTESIAN_POINT('Ctrl Pts',(1.82131873145266,-1.,-0.763673465462727));
#48477=CARTESIAN_POINT('Ctrl Pts',(1.82131873145266,1.,-0.763673465462727));
#48478=CARTESIAN_POINT('Ctrl Pts',(1.8153211840553,-1.,-0.763132003836634));
#48479=CARTESIAN_POINT('Ctrl Pts',(1.8153211840553,1.,-0.763132003836634));
#48480=CARTESIAN_POINT('Ctrl Pts',(1.80938551463965,-1.,-0.762546129463938));
#48481=CARTESIAN_POINT('Ctrl Pts',(1.80938551463965,1.,-0.762546129463938));
#48482=CARTESIAN_POINT('Ctrl Pts',(1.80351583877342,-1.,-0.761915336443547));
#48483=CARTESIAN_POINT('Ctrl Pts',(1.80351583877342,1.,-0.761915336443547));
#48484=CARTESIAN_POINT('Ctrl Pts',(1.79768986997783,-1.,-0.761229695230558));
#48485=CARTESIAN_POINT('Ctrl Pts',(1.79768986997783,1.,-0.761229695230558));
#48486=CARTESIAN_POINT('Ctrl Pts',(1.7918581561088,-1.,-0.760469555880749));
#48487=CARTESIAN_POINT('Ctrl Pts',(1.7918581561088,1.,-0.760469555880749));
#48488=CARTESIAN_POINT('Ctrl Pts',(1.78596964884604,-1.,-0.75961440111019));
#48489=CARTESIAN_POINT('Ctrl Pts',(1.78596964884604,1.,-0.75961440111019));
#48490=CARTESIAN_POINT('Ctrl Pts',(1.77999411220945,-1.,-0.758650626677519));
#48491=CARTESIAN_POINT('Ctrl Pts',(1.77999411220945,1.,-0.758650626677519));
#48492=CARTESIAN_POINT('Ctrl Pts',(1.77394167108292,-1.,-0.757578264077029));
#48493=CARTESIAN_POINT('Ctrl Pts',(1.77394167108292,1.,-0.757578264077029));
#48494=CARTESIAN_POINT('Ctrl Pts',(1.76789396002998,-1.,-0.75642189602781));
#48495=CARTESIAN_POINT('Ctrl Pts',(1.76789396002998,1.,-0.75642189602781));
#48496=CARTESIAN_POINT('Ctrl Pts',(1.76197817240128,-1.,-0.755220979974462));
#48497=CARTESIAN_POINT('Ctrl Pts',(1.76197817240128,1.,-0.755220979974462));
#48498=CARTESIAN_POINT('Ctrl Pts',(1.75631083600019,-1.,-0.754009254027829));
#48499=CARTESIAN_POINT('Ctrl Pts',(1.75631083600019,1.,-0.754009254027829));
#48500=CARTESIAN_POINT('Ctrl Pts',(1.75095139468794,-1.,-0.752797683531314));
#48501=CARTESIAN_POINT('Ctrl Pts',(1.75095139468794,1.,-0.752797683531314));
#48502=CARTESIAN_POINT('Ctrl Pts',(1.74585086852502,-1.,-0.751555614164483));
#48503=CARTESIAN_POINT('Ctrl Pts',(1.74585086852502,1.,-0.751555614164483));
#48504=CARTESIAN_POINT('Ctrl Pts',(1.74080458267114,-1.,-0.75019343598125));
#48505=CARTESIAN_POINT('Ctrl Pts',(1.74080458267114,1.,-0.75019343598125));
#48506=CARTESIAN_POINT('Ctrl Pts',(1.7355035168033,-1.,-0.74858246295687));
#48507=CARTESIAN_POINT('Ctrl Pts',(1.7355035168033,1.,-0.74858246295687));
#48508=CARTESIAN_POINT('Ctrl Pts',(1.72958533647714,-1.,-0.746574710097752));
#48509=CARTESIAN_POINT('Ctrl Pts',(1.72958533647714,1.,-0.746574710097752));
#48510=CARTESIAN_POINT('Ctrl Pts',(1.72268229916769,-1.,-0.744021445433094));
#48511=CARTESIAN_POINT('Ctrl Pts',(1.72268229916769,1.,-0.744021445433094));
#48512=CARTESIAN_POINT('Ctrl Pts',(1.71447789751001,-1.,-0.74079516202821));
#48513=CARTESIAN_POINT('Ctrl Pts',(1.71447789751001,1.,-0.74079516202821));
#48514=CARTESIAN_POINT('Ctrl Pts',(1.70473309004249,-1.,-0.736799665716932));
#48515=CARTESIAN_POINT('Ctrl Pts',(1.70473309004249,1.,-0.736799665716932));
#48516=CARTESIAN_POINT('Ctrl Pts',(1.69326921972915,-1.,-0.731963238685357));
#48517=CARTESIAN_POINT('Ctrl Pts',(1.69326921972915,1.,-0.731963238685357));
#48518=CARTESIAN_POINT('Ctrl Pts',(1.67996158451922,-1.,-0.726235967982445));
#48519=CARTESIAN_POINT('Ctrl Pts',(1.67996158451922,1.,-0.726235967982445));
#48520=CARTESIAN_POINT('Ctrl Pts',(1.66472880551777,-1.,-0.71958543378795));
#48521=CARTESIAN_POINT('Ctrl Pts',(1.66472880551777,1.,-0.71958543378795));
#48522=CARTESIAN_POINT('Ctrl Pts',(1.64752408828442,-1.,-0.711993139340448));
#48523=CARTESIAN_POINT('Ctrl Pts',(1.64752408828442,1.,-0.711993139340448));
#48524=CARTESIAN_POINT('Ctrl Pts',(1.6321654166204,-1.,-0.705159151977294));
#48525=CARTESIAN_POINT('Ctrl Pts',(1.6321654166204,1.,-0.705159151977294));
#48526=CARTESIAN_POINT('Ctrl Pts',(1.61974673471117,-1.,-0.699605146398837));
#48527=CARTESIAN_POINT('Ctrl Pts',(1.61974673471117,1.,-0.699605146398837));
#48528=CARTESIAN_POINT('Ctrl Pts',(1.61106790957619,-1.,-0.69571209787897));
#48529=CARTESIAN_POINT('Ctrl Pts',(1.61106790957619,1.,-0.69571209787897));
#48530=CARTESIAN_POINT('Ctrl Pts',(1.60662857109684,-1.,-0.693717979106306));
#48531=CARTESIAN_POINT('Ctrl Pts',(1.60662857109684,1.,-0.693717979106306));
#48532=CARTESIAN_POINT('',(2.0698113262342,1.,-0.745574324794401));
#48533=CARTESIAN_POINT('Ctrl Pts',(2.0698113262342,1.,-0.745574324794401));
#48534=CARTESIAN_POINT('Ctrl Pts',(2.06854248895728,1.,-0.745832791378367));
#48535=CARTESIAN_POINT('Ctrl Pts',(2.06600523016815,1.,-0.746345871544201));
#48536=CARTESIAN_POINT('Ctrl Pts',(2.06220058927826,1.,-0.74710393278792));
#48537=CARTESIAN_POINT('Ctrl Pts',(2.05713023031006,1.,-0.748091554183803));
#48538=CARTESIAN_POINT('Ctrl Pts',(2.05079645592154,1.,-0.749287468665046));
#48539=CARTESIAN_POINT('Ctrl Pts',(2.04446689147979,1.,-0.750444657875576));
#48540=CARTESIAN_POINT('Ctrl Pts',(2.03814160092099,1.,-0.751562963361115));
#48541=CARTESIAN_POINT('Ctrl Pts',(2.03182068456221,1.,-0.752642180487211));
#48542=CARTESIAN_POINT('Ctrl Pts',(2.02550428623313,1.,-0.753682061112768));
#48543=CARTESIAN_POINT('Ctrl Pts',(2.01919259405809,1.,-0.754682330722816));
#48544=CARTESIAN_POINT('Ctrl Pts',(2.01288584328084,1.,-0.755642704957865));
#48545=CARTESIAN_POINT('Ctrl Pts',(2.0065843158773,1.,-0.756562904646671));
#48546=CARTESIAN_POINT('Ctrl Pts',(2.00028834739178,1.,-0.757442676862724));
#48547=CARTESIAN_POINT('Ctrl Pts',(1.99399831098817,1.,-0.758281796766761));
#48548=CARTESIAN_POINT('Ctrl Pts',(1.98771456680874,1.,-0.759080037802488));
#48549=CARTESIAN_POINT('Ctrl Pts',(1.98143741418172,1.,-0.75983714745219));
#48550=CARTESIAN_POINT('Ctrl Pts',(1.97516705321494,1.,-0.760552825409757));
#48551=CARTESIAN_POINT('Ctrl Pts',(1.96890351582499,1.,-0.761226690483821));
#48552=CARTESIAN_POINT('Ctrl Pts',(1.96264672744186,1.,-0.761858300014424));
#48553=CARTESIAN_POINT('Ctrl Pts',(1.95639665309869,1.,-0.762447203806179));
#48554=CARTESIAN_POINT('Ctrl Pts',(1.95015342590024,1.,-0.762992990878769));
#48555=CARTESIAN_POINT('Ctrl Pts',(1.9439174661764,1.,-0.763495333538629));
#48556=CARTESIAN_POINT('Ctrl Pts',(1.93768964875886,1.,-0.763954049121459));
#48557=CARTESIAN_POINT('Ctrl Pts',(1.93147105496382,1.,-0.764369010673941));
#48558=CARTESIAN_POINT('Ctrl Pts',(1.92526263537048,1.,-0.764740025488212));
#48559=CARTESIAN_POINT('Ctrl Pts',(1.91906491634196,1.,-0.765066729667089));
#48560=CARTESIAN_POINT('Ctrl Pts',(1.91287765805169,1.,-0.765348465884722));
#48561=CARTESIAN_POINT('Ctrl Pts',(1.90669961402356,1.,-0.765584196937919));
#48562=CARTESIAN_POINT('Ctrl Pts',(1.90052930393596,1.,-0.765772772593386));
#48563=CARTESIAN_POINT('Ctrl Pts',(1.89436577771388,1.,-0.765913193856978));
#48564=CARTESIAN_POINT('Ctrl Pts',(1.88820926433409,1.,-0.766004837062091));
#48565=CARTESIAN_POINT('Ctrl Pts',(1.88206215302561,1.,-0.766047794851865));
#48566=CARTESIAN_POINT('Ctrl Pts',(1.87592888967883,1.,-0.766042837036744));
#48567=CARTESIAN_POINT('Ctrl Pts',(1.86981398314341,1.,-0.765990708546091));
#48568=CARTESIAN_POINT('Ctrl Pts',(1.86372027063312,1.,-0.765891519092547));
#48569=CARTESIAN_POINT('Ctrl Pts',(1.85764741390394,1.,-0.765744212909319));
#48570=CARTESIAN_POINT('Ctrl Pts',(1.85158945130063,1.,-0.765545710619063));
#48571=CARTESIAN_POINT('Ctrl Pts',(1.84553698875924,1.,-0.765291664862029));
#48572=CARTESIAN_POINT('Ctrl Pts',(1.83948181064835,1.,-0.764978057881738));
#48573=CARTESIAN_POINT('Ctrl Pts',(1.83342077227142,1.,-0.764602549687853));
#48574=CARTESIAN_POINT('Ctrl Pts',(1.82735991200065,1.,-0.764165902605995));
#48575=CARTESIAN_POINT('Ctrl Pts',(1.82131873145266,1.,-0.763673465462727));
#48576=CARTESIAN_POINT('Ctrl Pts',(1.8153211840553,1.,-0.763132003836634));
#48577=CARTESIAN_POINT('Ctrl Pts',(1.80938551463965,1.,-0.762546129463938));
#48578=CARTESIAN_POINT('Ctrl Pts',(1.80351583877342,1.,-0.761915336443547));
#48579=CARTESIAN_POINT('Ctrl Pts',(1.79768986997783,1.,-0.761229695230558));
#48580=CARTESIAN_POINT('Ctrl Pts',(1.7918581561088,1.,-0.760469555880749));
#48581=CARTESIAN_POINT('Ctrl Pts',(1.78596964884604,1.,-0.75961440111019));
#48582=CARTESIAN_POINT('Ctrl Pts',(1.77999411220945,1.,-0.758650626677519));
#48583=CARTESIAN_POINT('Ctrl Pts',(1.77394167108292,1.,-0.757578264077029));
#48584=CARTESIAN_POINT('Ctrl Pts',(1.76789396002998,1.,-0.75642189602781));
#48585=CARTESIAN_POINT('Ctrl Pts',(1.76197817240128,1.,-0.755220979974462));
#48586=CARTESIAN_POINT('Ctrl Pts',(1.75631083600019,1.,-0.754009254027829));
#48587=CARTESIAN_POINT('Ctrl Pts',(1.75095139468794,1.,-0.752797683531314));
#48588=CARTESIAN_POINT('Ctrl Pts',(1.74585086852502,1.,-0.751555614164483));
#48589=CARTESIAN_POINT('Ctrl Pts',(1.74080458267114,1.,-0.75019343598125));
#48590=CARTESIAN_POINT('Ctrl Pts',(1.7355035168033,1.,-0.74858246295687));
#48591=CARTESIAN_POINT('Ctrl Pts',(1.72958533647714,1.,-0.746574710097752));
#48592=CARTESIAN_POINT('Ctrl Pts',(1.72268229916769,1.,-0.744021445433094));
#48593=CARTESIAN_POINT('Ctrl Pts',(1.71447789751001,1.,-0.74079516202821));
#48594=CARTESIAN_POINT('Ctrl Pts',(1.70473309004249,1.,-0.736799665716932));
#48595=CARTESIAN_POINT('Ctrl Pts',(1.69326921972915,1.,-0.731963238685357));
#48596=CARTESIAN_POINT('Ctrl Pts',(1.67996158451922,1.,-0.726235967982445));
#48597=CARTESIAN_POINT('Ctrl Pts',(1.66472880551777,1.,-0.71958543378795));
#48598=CARTESIAN_POINT('Ctrl Pts',(1.64752408828442,1.,-0.711993139340448));
#48599=CARTESIAN_POINT('Ctrl Pts',(1.6321654166204,1.,-0.705159151977294));
#48600=CARTESIAN_POINT('Ctrl Pts',(1.61974673471117,1.,-0.699605146398837));
#48601=CARTESIAN_POINT('Ctrl Pts',(1.61106790957619,1.,-0.69571209787897));
#48602=CARTESIAN_POINT('Ctrl Pts',(1.60662857109684,1.,-0.693717979106306));
#48603=CARTESIAN_POINT('',(2.0698113262342,0.,-0.745574324794401));
#48604=CARTESIAN_POINT('Origin',(2.11275013067528,0.,-0.61342227326009));
#48605=CARTESIAN_POINT('',(2.11275013067528,1.,-0.61342227326009));
#48606=CARTESIAN_POINT('',(2.0698113262342,1.,-0.745574324794401));
#48607=CARTESIAN_POINT('',(2.11275013067528,0.,-0.61342227326009));
#48608=CARTESIAN_POINT('Ctrl Pts',(1.7075470150345,-1.,-0.383122945602004));
#48609=CARTESIAN_POINT('Ctrl Pts',(1.7075470150345,1.,-0.383122945602004));
#48610=CARTESIAN_POINT('Ctrl Pts',(1.71231062891958,-1.,-0.384119047315542));
#48611=CARTESIAN_POINT('Ctrl Pts',(1.71231062891958,1.,-0.384119047315542));
#48612=CARTESIAN_POINT('Ctrl Pts',(1.72162022246158,-1.,-0.38607079032701));
#48613=CARTESIAN_POINT('Ctrl Pts',(1.72162022246158,1.,-0.38607079032701));
#48614=CARTESIAN_POINT('Ctrl Pts',(1.7349317097561,-1.,-0.388877023509192));
#48615=CARTESIAN_POINT('Ctrl Pts',(1.7349317097561,1.,-0.388877023509192));
#48616=CARTESIAN_POINT('Ctrl Pts',(1.75137405313962,-1.,-0.392375812294307));
#48617=CARTESIAN_POINT('Ctrl Pts',(1.75137405313962,1.,-0.392375812294307));
#48618=CARTESIAN_POINT('Ctrl Pts',(1.7697556004756,-1.,-0.39634619612042));
#48619=CARTESIAN_POINT('Ctrl Pts',(1.7697556004756,1.,-0.39634619612042));
#48620=CARTESIAN_POINT('Ctrl Pts',(1.78598826347533,-1.,-0.399919403783081));
#48621=CARTESIAN_POINT('Ctrl Pts',(1.78598826347533,1.,-0.399919403783081));
#48622=CARTESIAN_POINT('Ctrl Pts',(1.80012077176221,-1.,-0.403107976170441));
#48623=CARTESIAN_POINT('Ctrl Pts',(1.80012077176221,1.,-0.403107976170441));
#48624=CARTESIAN_POINT('Ctrl Pts',(1.81223801813988,-1.,-0.405933518411838));
#48625=CARTESIAN_POINT('Ctrl Pts',(1.81223801813988,1.,-0.405933518411838));
#48626=CARTESIAN_POINT('Ctrl Pts',(1.8224702267854,-1.,-0.408428948108534));
#48627=CARTESIAN_POINT('Ctrl Pts',(1.8224702267854,1.,-0.408428948108534));
#48628=CARTESIAN_POINT('Ctrl Pts',(1.83100408895216,-1.,-0.410641256301675));
#48629=CARTESIAN_POINT('Ctrl Pts',(1.83100408895216,1.,-0.410641256301675));
#48630=CARTESIAN_POINT('Ctrl Pts',(1.83808953475839,-1.,-0.412633125322162));
#48631=CARTESIAN_POINT('Ctrl Pts',(1.83808953475839,1.,-0.412633125322162));
#48632=CARTESIAN_POINT('Ctrl Pts',(1.8440575707371,-1.,-0.41448743825434));
#48633=CARTESIAN_POINT('Ctrl Pts',(1.8440575707371,1.,-0.41448743825434));
#48634=CARTESIAN_POINT('Ctrl Pts',(1.84929312929882,-1.,-0.416300022038864));
#48635=CARTESIAN_POINT('Ctrl Pts',(1.84929312929882,1.,-0.416300022038864));
#48636=CARTESIAN_POINT('Ctrl Pts',(1.85417632856234,-1.,-0.418164129143534));
#48637=CARTESIAN_POINT('Ctrl Pts',(1.85417632856234,1.,-0.418164129143534));
#48638=CARTESIAN_POINT('Ctrl Pts',(1.85903281096686,-1.,-0.42015728797562));
#48639=CARTESIAN_POINT('Ctrl Pts',(1.85903281096686,1.,-0.42015728797562));
#48640=CARTESIAN_POINT('Ctrl Pts',(1.86408083334028,-1.,-0.422327307418275));
#48641=CARTESIAN_POINT('Ctrl Pts',(1.86408083334028,1.,-0.422327307418275));
#48642=CARTESIAN_POINT('Ctrl Pts',(1.86937803944323,-1.,-0.424678177291359));
#48643=CARTESIAN_POINT('Ctrl Pts',(1.86937803944323,1.,-0.424678177291359));
#48644=CARTESIAN_POINT('Ctrl Pts',(1.87486989291484,-1.,-0.427183828519102));
#48645=CARTESIAN_POINT('Ctrl Pts',(1.87486989291484,1.,-0.427183828519102));
#48646=CARTESIAN_POINT('Ctrl Pts',(1.88044229001832,-1.,-0.429803062482345));
#48647=CARTESIAN_POINT('Ctrl Pts',(1.88044229001832,1.,-0.429803062482345));
#48648=CARTESIAN_POINT('Ctrl Pts',(1.88596913666793,-1.,-0.432493038548748));
#48649=CARTESIAN_POINT('Ctrl Pts',(1.88596913666793,1.,-0.432493038548748));
#48650=CARTESIAN_POINT('Ctrl Pts',(1.89136993975504,-1.,-0.435225660963383));
#48651=CARTESIAN_POINT('Ctrl Pts',(1.89136993975504,1.,-0.435225660963383));
#48652=CARTESIAN_POINT('Ctrl Pts',(1.89663648956466,-1.,-0.437995003948244));
#48653=CARTESIAN_POINT('Ctrl Pts',(1.89663648956466,1.,-0.437995003948244));
#48654=CARTESIAN_POINT('Ctrl Pts',(1.90180124389086,-1.,-0.440807833704038));
#48655=CARTESIAN_POINT('Ctrl Pts',(1.90180124389086,1.,-0.440807833704038));
#48656=CARTESIAN_POINT('Ctrl Pts',(1.90691756144898,-1.,-0.443677556849151));
#48657=CARTESIAN_POINT('Ctrl Pts',(1.90691756144898,1.,-0.443677556849151));
#48658=CARTESIAN_POINT('Ctrl Pts',(1.9120369998112,-1.,-0.446617343485711));
#48659=CARTESIAN_POINT('Ctrl Pts',(1.9120369998112,1.,-0.446617343485711));
#48660=CARTESIAN_POINT('Ctrl Pts',(1.91718342555755,-1.,-0.449632260106662));
#48661=CARTESIAN_POINT('Ctrl Pts',(1.91718342555755,1.,-0.449632260106662));
#48662=CARTESIAN_POINT('Ctrl Pts',(1.92235380648502,-1.,-0.452719478359433));
#48663=CARTESIAN_POINT('Ctrl Pts',(1.92235380648502,1.,-0.452719478359433));
#48664=CARTESIAN_POINT('Ctrl Pts',(1.92753067150476,-1.,-0.455872005174371));
#48665=CARTESIAN_POINT('Ctrl Pts',(1.92753067150476,1.,-0.455872005174371));
#48666=CARTESIAN_POINT('Ctrl Pts',(1.93269066517934,-1.,-0.459081234547926));
#48667=CARTESIAN_POINT('Ctrl Pts',(1.93269066517934,1.,-0.459081234547926));
#48668=CARTESIAN_POINT('Ctrl Pts',(1.93781486640821,-1.,-0.462340031009057));
#48669=CARTESIAN_POINT('Ctrl Pts',(1.93781486640821,1.,-0.462340031009057));
#48670=CARTESIAN_POINT('Ctrl Pts',(1.9428979419619,-1.,-0.46564546202603));
#48671=CARTESIAN_POINT('Ctrl Pts',(1.9428979419619,1.,-0.46564546202603));
#48672=CARTESIAN_POINT('Ctrl Pts',(1.94794381136514,-1.,-0.468997482913135));
#48673=CARTESIAN_POINT('Ctrl Pts',(1.94794381136514,1.,-0.468997482913135));
#48674=CARTESIAN_POINT('Ctrl Pts',(1.95296148278133,-1.,-0.472397672264072));
#48675=CARTESIAN_POINT('Ctrl Pts',(1.95296148278133,1.,-0.472397672264072));
#48676=CARTESIAN_POINT('Ctrl Pts',(1.95796111148177,-1.,-0.475848034683176));
#48677=CARTESIAN_POINT('Ctrl Pts',(1.95796111148177,1.,-0.475848034683176));
#48678=CARTESIAN_POINT('Ctrl Pts',(1.96294933055943,-1.,-0.479349583074855));
#48679=CARTESIAN_POINT('Ctrl Pts',(1.96294933055943,1.,-0.479349583074855));
#48680=CARTESIAN_POINT('Ctrl Pts',(1.96792703422362,-1.,-0.482901662120691));
#48681=CARTESIAN_POINT('Ctrl Pts',(1.96792703422362,1.,-0.482901662120691));
#48682=CARTESIAN_POINT('Ctrl Pts',(1.97289186263272,-1.,-0.486502692907659));
#48683=CARTESIAN_POINT('Ctrl Pts',(1.97289186263272,1.,-0.486502692907659));
#48684=CARTESIAN_POINT('Ctrl Pts',(1.97783973019229,-1.,-0.490150627860953));
#48685=CARTESIAN_POINT('Ctrl Pts',(1.97783973019229,1.,-0.490150627860953));
#48686=CARTESIAN_POINT('Ctrl Pts',(1.98276658761821,-1.,-0.493843476541495));
#48687=CARTESIAN_POINT('Ctrl Pts',(1.98276658761821,1.,-0.493843476541495));
#48688=CARTESIAN_POINT('Ctrl Pts',(1.98767044752932,-1.,-0.497579909545574));
#48689=CARTESIAN_POINT('Ctrl Pts',(1.98767044752932,1.,-0.497579909545574));
#48690=CARTESIAN_POINT('Ctrl Pts',(1.99255149126155,-1.,-0.501359287727146));
#48691=CARTESIAN_POINT('Ctrl Pts',(1.99255149126155,1.,-0.501359287727146));
#48692=CARTESIAN_POINT('Ctrl Pts',(1.99741107463572,-1.,-0.505181361323026));
#48693=CARTESIAN_POINT('Ctrl Pts',(1.99741107463572,1.,-0.505181361323026));
#48694=CARTESIAN_POINT('Ctrl Pts',(2.00225107134734,-1.,-0.509046069886157));
#48695=CARTESIAN_POINT('Ctrl Pts',(2.00225107134734,1.,-0.509046069886157));
#48696=CARTESIAN_POINT('Ctrl Pts',(2.00707309946949,-1.,-0.512953306961793));
#48697=CARTESIAN_POINT('Ctrl Pts',(2.00707309946949,1.,-0.512953306961793));
#48698=CARTESIAN_POINT('Ctrl Pts',(2.01187773939242,-1.,-0.516902681728687));
#48699=CARTESIAN_POINT('Ctrl Pts',(2.01187773939242,1.,-0.516902681728687));
#48700=CARTESIAN_POINT('Ctrl Pts',(2.01666477917286,-1.,-0.520893590399371));
#48701=CARTESIAN_POINT('Ctrl Pts',(2.01666477917286,1.,-0.520893590399371));
#48702=CARTESIAN_POINT('Ctrl Pts',(2.02143356304698,-1.,-0.524925318333476));
#48703=CARTESIAN_POINT('Ctrl Pts',(2.02143356304698,1.,-0.524925318333476));
#48704=CARTESIAN_POINT('Ctrl Pts',(2.0261832908329,-1.,-0.528997127241914));
#48705=CARTESIAN_POINT('Ctrl Pts',(2.0261832908329,1.,-0.528997127241914));
#48706=CARTESIAN_POINT('Ctrl Pts',(2.03091336214426,-1.,-0.533108355132977));
#48707=CARTESIAN_POINT('Ctrl Pts',(2.03091336214426,1.,-0.533108355132977));
#48708=CARTESIAN_POINT('Ctrl Pts',(2.03562362954037,-1.,-0.537258489833262));
#48709=CARTESIAN_POINT('Ctrl Pts',(2.03562362954037,1.,-0.537258489833262));
#48710=CARTESIAN_POINT('Ctrl Pts',(2.04031422690527,-1.,-0.541447120615659));
#48711=CARTESIAN_POINT('Ctrl Pts',(2.04031422690527,1.,-0.541447120615659));
#48712=CARTESIAN_POINT('Ctrl Pts',(2.04498544714588,-1.,-0.54567390381743));
#48713=CARTESIAN_POINT('Ctrl Pts',(2.04498544714588,1.,-0.54567390381743));
#48714=CARTESIAN_POINT('Ctrl Pts',(2.04963761077958,-1.,-0.549938525150295));
#48715=CARTESIAN_POINT('Ctrl Pts',(2.04963761077958,1.,-0.549938525150295));
#48716=CARTESIAN_POINT('Ctrl Pts',(2.05427091604413,-1.,-0.554240657463906));
#48717=CARTESIAN_POINT('Ctrl Pts',(2.05427091604413,1.,-0.554240657463906));
#48718=CARTESIAN_POINT('Ctrl Pts',(2.05888537756462,-1.,-0.558579940185152));
#48719=CARTESIAN_POINT('Ctrl Pts',(2.05888537756462,1.,-0.558579940185152));
#48720=CARTESIAN_POINT('Ctrl Pts',(2.06348090160589,-1.,-0.562955993082262));
#48721=CARTESIAN_POINT('Ctrl Pts',(2.06348090160589,1.,-0.562955993082262));
#48722=CARTESIAN_POINT('Ctrl Pts',(2.06805732997334,-1.,-0.567368421181087));
#48723=CARTESIAN_POINT('Ctrl Pts',(2.06805732997334,1.,-0.567368421181087));
#48724=CARTESIAN_POINT('Ctrl Pts',(2.07261449292824,-1.,-0.571816823242603));
#48725=CARTESIAN_POINT('Ctrl Pts',(2.07261449292824,1.,-0.571816823242603));
#48726=CARTESIAN_POINT('Ctrl Pts',(2.07715226767559,-1.,-0.576300797416845));
#48727=CARTESIAN_POINT('Ctrl Pts',(2.07715226767559,1.,-0.576300797416845));
#48728=CARTESIAN_POINT('Ctrl Pts',(2.08167059018418,-1.,-0.580819952108064));
#48729=CARTESIAN_POINT('Ctrl Pts',(2.08167059018418,1.,-0.580819952108064));
#48730=CARTESIAN_POINT('Ctrl Pts',(2.08616943727951,-1.,-0.585373918991617));
#48731=CARTESIAN_POINT('Ctrl Pts',(2.08616943727951,1.,-0.585373918991617));
#48732=CARTESIAN_POINT('Ctrl Pts',(2.09064881812129,-1.,-0.589962365403406));
#48733=CARTESIAN_POINT('Ctrl Pts',(2.09064881812129,1.,-0.589962365403406));
#48734=CARTESIAN_POINT('Ctrl Pts',(2.0951087622027,-1.,-0.594585006052162));
#48735=CARTESIAN_POINT('Ctrl Pts',(2.0951087622027,1.,-0.594585006052162));
#48736=CARTESIAN_POINT('Ctrl Pts',(2.0995493086477,-1.,-0.599241616420534));
#48737=CARTESIAN_POINT('Ctrl Pts',(2.0995493086477,1.,-0.599241616420534));
#48738=CARTESIAN_POINT('Ctrl Pts',(2.10397049886949,-1.,-0.60393203073603));
#48739=CARTESIAN_POINT('Ctrl Pts',(2.10397049886949,1.,-0.60393203073603));
#48740=CARTESIAN_POINT('Ctrl Pts',(2.1074919961518,-1.,-0.607711315454876));
#48741=CARTESIAN_POINT('Ctrl Pts',(2.1074919961518,1.,-0.607711315454876));
#48742=CARTESIAN_POINT('Ctrl Pts',(2.11012443807238,-1.,-0.610560911689899));
#48743=CARTESIAN_POINT('Ctrl Pts',(2.11012443807238,1.,-0.610560911689899));
#48744=CARTESIAN_POINT('Ctrl Pts',(2.11187554259986,-1.,-0.6124673655618));
#48745=CARTESIAN_POINT('Ctrl Pts',(2.11187554259986,1.,-0.6124673655618));
#48746=CARTESIAN_POINT('Ctrl Pts',(2.11275013067528,-1.,-0.61342227326009));
#48747=CARTESIAN_POINT('Ctrl Pts',(2.11275013067528,1.,-0.61342227326009));
#48748=CARTESIAN_POINT('',(1.7075470150345,1.,-0.383122945602004));
#48749=CARTESIAN_POINT('Ctrl Pts',(1.7075470150345,1.,-0.383122945602004));
#48750=CARTESIAN_POINT('Ctrl Pts',(1.71231062891958,1.,-0.384119047315542));
#48751=CARTESIAN_POINT('Ctrl Pts',(1.72162022246158,1.,-0.38607079032701));
#48752=CARTESIAN_POINT('Ctrl Pts',(1.7349317097561,1.,-0.388877023509192));
#48753=CARTESIAN_POINT('Ctrl Pts',(1.75137405313962,1.,-0.392375812294307));
#48754=CARTESIAN_POINT('Ctrl Pts',(1.7697556004756,1.,-0.39634619612042));
#48755=CARTESIAN_POINT('Ctrl Pts',(1.78598826347533,1.,-0.399919403783081));
#48756=CARTESIAN_POINT('Ctrl Pts',(1.80012077176221,1.,-0.403107976170441));
#48757=CARTESIAN_POINT('Ctrl Pts',(1.81223801813988,1.,-0.405933518411838));
#48758=CARTESIAN_POINT('Ctrl Pts',(1.8224702267854,1.,-0.408428948108534));
#48759=CARTESIAN_POINT('Ctrl Pts',(1.83100408895216,1.,-0.410641256301675));
#48760=CARTESIAN_POINT('Ctrl Pts',(1.83808953475839,1.,-0.412633125322162));
#48761=CARTESIAN_POINT('Ctrl Pts',(1.8440575707371,1.,-0.41448743825434));
#48762=CARTESIAN_POINT('Ctrl Pts',(1.84929312929882,1.,-0.416300022038864));
#48763=CARTESIAN_POINT('Ctrl Pts',(1.85417632856234,1.,-0.418164129143534));
#48764=CARTESIAN_POINT('Ctrl Pts',(1.85903281096686,1.,-0.42015728797562));
#48765=CARTESIAN_POINT('Ctrl Pts',(1.86408083334028,1.,-0.422327307418275));
#48766=CARTESIAN_POINT('Ctrl Pts',(1.86937803944323,1.,-0.424678177291359));
#48767=CARTESIAN_POINT('Ctrl Pts',(1.87486989291484,1.,-0.427183828519102));
#48768=CARTESIAN_POINT('Ctrl Pts',(1.88044229001832,1.,-0.429803062482345));
#48769=CARTESIAN_POINT('Ctrl Pts',(1.88596913666793,1.,-0.432493038548748));
#48770=CARTESIAN_POINT('Ctrl Pts',(1.89136993975504,1.,-0.435225660963383));
#48771=CARTESIAN_POINT('Ctrl Pts',(1.89663648956466,1.,-0.437995003948244));
#48772=CARTESIAN_POINT('Ctrl Pts',(1.90180124389086,1.,-0.440807833704038));
#48773=CARTESIAN_POINT('Ctrl Pts',(1.90691756144898,1.,-0.443677556849151));
#48774=CARTESIAN_POINT('Ctrl Pts',(1.9120369998112,1.,-0.446617343485711));
#48775=CARTESIAN_POINT('Ctrl Pts',(1.91718342555755,1.,-0.449632260106662));
#48776=CARTESIAN_POINT('Ctrl Pts',(1.92235380648502,1.,-0.452719478359433));
#48777=CARTESIAN_POINT('Ctrl Pts',(1.92753067150476,1.,-0.455872005174371));
#48778=CARTESIAN_POINT('Ctrl Pts',(1.93269066517934,1.,-0.459081234547926));
#48779=CARTESIAN_POINT('Ctrl Pts',(1.93781486640821,1.,-0.462340031009057));
#48780=CARTESIAN_POINT('Ctrl Pts',(1.9428979419619,1.,-0.46564546202603));
#48781=CARTESIAN_POINT('Ctrl Pts',(1.94794381136514,1.,-0.468997482913135));
#48782=CARTESIAN_POINT('Ctrl Pts',(1.95296148278133,1.,-0.472397672264072));
#48783=CARTESIAN_POINT('Ctrl Pts',(1.95796111148177,1.,-0.475848034683176));
#48784=CARTESIAN_POINT('Ctrl Pts',(1.96294933055943,1.,-0.479349583074855));
#48785=CARTESIAN_POINT('Ctrl Pts',(1.96792703422362,1.,-0.482901662120691));
#48786=CARTESIAN_POINT('Ctrl Pts',(1.97289186263272,1.,-0.486502692907659));
#48787=CARTESIAN_POINT('Ctrl Pts',(1.97783973019229,1.,-0.490150627860953));
#48788=CARTESIAN_POINT('Ctrl Pts',(1.98276658761821,1.,-0.493843476541495));
#48789=CARTESIAN_POINT('Ctrl Pts',(1.98767044752932,1.,-0.497579909545574));
#48790=CARTESIAN_POINT('Ctrl Pts',(1.99255149126155,1.,-0.501359287727146));
#48791=CARTESIAN_POINT('Ctrl Pts',(1.99741107463572,1.,-0.505181361323026));
#48792=CARTESIAN_POINT('Ctrl Pts',(2.00225107134734,1.,-0.509046069886157));
#48793=CARTESIAN_POINT('Ctrl Pts',(2.00707309946949,1.,-0.512953306961793));
#48794=CARTESIAN_POINT('Ctrl Pts',(2.01187773939242,1.,-0.516902681728687));
#48795=CARTESIAN_POINT('Ctrl Pts',(2.01666477917286,1.,-0.520893590399371));
#48796=CARTESIAN_POINT('Ctrl Pts',(2.02143356304698,1.,-0.524925318333476));
#48797=CARTESIAN_POINT('Ctrl Pts',(2.0261832908329,1.,-0.528997127241914));
#48798=CARTESIAN_POINT('Ctrl Pts',(2.03091336214426,1.,-0.533108355132977));
#48799=CARTESIAN_POINT('Ctrl Pts',(2.03562362954037,1.,-0.537258489833262));
#48800=CARTESIAN_POINT('Ctrl Pts',(2.04031422690527,1.,-0.541447120615659));
#48801=CARTESIAN_POINT('Ctrl Pts',(2.04498544714588,1.,-0.54567390381743));
#48802=CARTESIAN_POINT('Ctrl Pts',(2.04963761077958,1.,-0.549938525150295));
#48803=CARTESIAN_POINT('Ctrl Pts',(2.05427091604413,1.,-0.554240657463906));
#48804=CARTESIAN_POINT('Ctrl Pts',(2.05888537756462,1.,-0.558579940185152));
#48805=CARTESIAN_POINT('Ctrl Pts',(2.06348090160589,1.,-0.562955993082262));
#48806=CARTESIAN_POINT('Ctrl Pts',(2.06805732997334,1.,-0.567368421181087));
#48807=CARTESIAN_POINT('Ctrl Pts',(2.07261449292824,1.,-0.571816823242603));
#48808=CARTESIAN_POINT('Ctrl Pts',(2.07715226767559,1.,-0.576300797416845));
#48809=CARTESIAN_POINT('Ctrl Pts',(2.08167059018418,1.,-0.580819952108064));
#48810=CARTESIAN_POINT('Ctrl Pts',(2.08616943727951,1.,-0.585373918991617));
#48811=CARTESIAN_POINT('Ctrl Pts',(2.09064881812129,1.,-0.589962365403406));
#48812=CARTESIAN_POINT('Ctrl Pts',(2.0951087622027,1.,-0.594585006052162));
#48813=CARTESIAN_POINT('Ctrl Pts',(2.0995493086477,1.,-0.599241616420534));
#48814=CARTESIAN_POINT('Ctrl Pts',(2.10397049886949,1.,-0.60393203073603));
#48815=CARTESIAN_POINT('Ctrl Pts',(2.1074919961518,1.,-0.607711315454876));
#48816=CARTESIAN_POINT('Ctrl Pts',(2.11012443807238,1.,-0.610560911689899));
#48817=CARTESIAN_POINT('Ctrl Pts',(2.11187554259986,1.,-0.6124673655618));
#48818=CARTESIAN_POINT('Ctrl Pts',(2.11275013067528,1.,-0.61342227326009));
#48819=CARTESIAN_POINT('',(1.7075470150345,0.,-0.383122945602001));
#48820=CARTESIAN_POINT('Origin',(0.,0.,0.));
#48821=CARTESIAN_POINT('',(1.74236521665491,1.,-0.163289472382896));
#48822=CARTESIAN_POINT('Origin',(0.,1.,0.));
#48823=CARTESIAN_POINT('',(1.74236521665491,0.,-0.163289472382896));
#48824=CARTESIAN_POINT('Ctrl Pts',(2.19890268624765,-1.,-0.0694764450219582));
#48825=CARTESIAN_POINT('Ctrl Pts',(2.19890268624765,1.,-0.0694764450219582));
#48826=CARTESIAN_POINT('Ctrl Pts',(2.19777582085423,-1.,-0.0701143536325491));
#48827=CARTESIAN_POINT('Ctrl Pts',(2.19777582085423,1.,-0.0701143536325491));
#48828=CARTESIAN_POINT('Ctrl Pts',(2.19552129484002,-1.,-0.0713863779526155));
#48829=CARTESIAN_POINT('Ctrl Pts',(2.19552129484002,1.,-0.0713863779526155));
#48830=CARTESIAN_POINT('Ctrl Pts',(2.19213712013662,-1.,-0.0732830357306726));
#48831=CARTESIAN_POINT('Ctrl Pts',(2.19213712013662,1.,-0.0732830357306726));
#48832=CARTESIAN_POINT('Ctrl Pts',(2.1876201139953,-1.,-0.0757891465836149));
#48833=CARTESIAN_POINT('Ctrl Pts',(2.1876201139953,1.,-0.0757891465836149));
#48834=CARTESIAN_POINT('Ctrl Pts',(2.18196589448887,-1.,-0.0788837727685244));
#48835=CARTESIAN_POINT('Ctrl Pts',(2.18196589448887,1.,-0.0788837727685244));
#48836=CARTESIAN_POINT('Ctrl Pts',(2.176303712113,-1.,-0.0819402680872767));
#48837=CARTESIAN_POINT('Ctrl Pts',(2.176303712113,1.,-0.0819402680872767));
#48838=CARTESIAN_POINT('Ctrl Pts',(2.17063357870952,-1.,-0.0849584620835374));
#48839=CARTESIAN_POINT('Ctrl Pts',(2.17063357870952,1.,-0.0849584620835374));
#48840=CARTESIAN_POINT('Ctrl Pts',(2.16495552645014,-1.,-0.0879381291386924));
#48841=CARTESIAN_POINT('Ctrl Pts',(2.16495552645014,1.,-0.0879381291386924));
#48842=CARTESIAN_POINT('Ctrl Pts',(2.15926961544516,-1.,-0.0908789888107267));
#48843=CARTESIAN_POINT('Ctrl Pts',(2.15926961544516,1.,-0.0908789888107267));
#48844=CARTESIAN_POINT('Ctrl Pts',(2.1535759397817,-1.,-0.0937807218867645));
#48845=CARTESIAN_POINT('Ctrl Pts',(2.1535759397817,1.,-0.0937807218867645));
#48846=CARTESIAN_POINT('Ctrl Pts',(2.14787463531795,-1.,-0.096642985230546));
#48847=CARTESIAN_POINT('Ctrl Pts',(2.14787463531795,1.,-0.096642985230546));
#48848=CARTESIAN_POINT('Ctrl Pts',(2.14216588396025,-1.,-0.0994654261990917));
#48849=CARTESIAN_POINT('Ctrl Pts',(2.14216588396025,1.,-0.0994654261990917));
#48850=CARTESIAN_POINT('Ctrl Pts',(2.13644992667165,-1.,-0.102247700556101));
#48851=CARTESIAN_POINT('Ctrl Pts',(2.13644992667165,1.,-0.102247700556101));
#48852=CARTESIAN_POINT('Ctrl Pts',(2.13072704887293,-1.,-0.10498947915274));
#48853=CARTESIAN_POINT('Ctrl Pts',(2.13072704887293,1.,-0.10498947915274));
#48854=CARTESIAN_POINT('Ctrl Pts',(2.12499752307,-1.,-0.10769043523109));
#48855=CARTESIAN_POINT('Ctrl Pts',(2.12499752307,1.,-0.10769043523109));
#48856=CARTESIAN_POINT('Ctrl Pts',(2.11926155590865,-1.,-0.110350236135025));
#48857=CARTESIAN_POINT('Ctrl Pts',(2.11926155590865,1.,-0.110350236135025));
#48858=CARTESIAN_POINT('Ctrl Pts',(2.11351924490306,-1.,-0.112968534419737));
#48859=CARTESIAN_POINT('Ctrl Pts',(2.11351924490306,1.,-0.112968534419737));
#48860=CARTESIAN_POINT('Ctrl Pts',(2.10777050261309,-1.,-0.115544957687927));
#48861=CARTESIAN_POINT('Ctrl Pts',(2.10777050261309,1.,-0.115544957687927));
#48862=CARTESIAN_POINT('Ctrl Pts',(2.102015121329,-1.,-0.118079107988356));
#48863=CARTESIAN_POINT('Ctrl Pts',(2.102015121329,1.,-0.118079107988356));
#48864=CARTESIAN_POINT('Ctrl Pts',(2.0962529286773,-1.,-0.120570567965122));
#48865=CARTESIAN_POINT('Ctrl Pts',(2.0962529286773,1.,-0.120570567965122));
#48866=CARTESIAN_POINT('Ctrl Pts',(2.09048392424825,-1.,-0.123018905621083));
#48867=CARTESIAN_POINT('Ctrl Pts',(2.09048392424825,1.,-0.123018905621083));
#48868=CARTESIAN_POINT('Ctrl Pts',(2.08470840653643,-1.,-0.125423679412062));
#48869=CARTESIAN_POINT('Ctrl Pts',(2.08470840653643,1.,-0.125423679412062));
#48870=CARTESIAN_POINT('Ctrl Pts',(2.07892715110987,-1.,-0.12778444527612));
#48871=CARTESIAN_POINT('Ctrl Pts',(2.07892715110987,1.,-0.12778444527612));
#48872=CARTESIAN_POINT('Ctrl Pts',(2.07314114713063,-1.,-0.130100748328404));
#48873=CARTESIAN_POINT('Ctrl Pts',(2.07314114713063,1.,-0.130100748328404));
#48874=CARTESIAN_POINT('Ctrl Pts',(2.06735123910326,-1.,-0.132372111547711));
#48875=CARTESIAN_POINT('Ctrl Pts',(2.06735123910326,1.,-0.132372111547711));
#48876=CARTESIAN_POINT('Ctrl Pts',(2.06155781517842,-1.,-0.134598026192106));
#48877=CARTESIAN_POINT('Ctrl Pts',(2.06155781517842,1.,-0.134598026192106));
#48878=CARTESIAN_POINT('Ctrl Pts',(2.05576044414264,-1.,-0.136777941218044));
#48879=CARTESIAN_POINT('Ctrl Pts',(2.05576044414264,1.,-0.136777941218044));
#48880=CARTESIAN_POINT('Ctrl Pts',(2.04995762001328,-1.,-0.138911255368966));
#48881=CARTESIAN_POINT('Ctrl Pts',(2.04995762001328,1.,-0.138911255368966));
#48882=CARTESIAN_POINT('Ctrl Pts',(2.04414757947916,-1.,-0.140997332152546));
#48883=CARTESIAN_POINT('Ctrl Pts',(2.04414757947916,1.,-0.140997332152546));
#48884=CARTESIAN_POINT('Ctrl Pts',(2.03832911025912,-1.,-0.143035515058209));
#48885=CARTESIAN_POINT('Ctrl Pts',(2.03832911025912,1.,-0.143035515058209));
#48886=CARTESIAN_POINT('Ctrl Pts',(2.03250223739942,-1.,-0.145025140186058));
#48887=CARTESIAN_POINT('Ctrl Pts',(2.03250223739942,1.,-0.145025140186058));
#48888=CARTESIAN_POINT('Ctrl Pts',(2.02666926182017,-1.,-0.146965557332583));
#48889=CARTESIAN_POINT('Ctrl Pts',(2.02666926182017,1.,-0.146965557332583));
#48890=CARTESIAN_POINT('Ctrl Pts',(2.02083464969894,-1.,-0.148856124775337));
#48891=CARTESIAN_POINT('Ctrl Pts',(2.02083464969894,1.,-0.148856124775337));
#48892=CARTESIAN_POINT('Ctrl Pts',(2.01500291940238,-1.,-0.150696157673078));
#48893=CARTESIAN_POINT('Ctrl Pts',(2.01500291940238,1.,-0.150696157673078));
#48894=CARTESIAN_POINT('Ctrl Pts',(2.00917680318424,-1.,-0.15248488362145));
#48895=CARTESIAN_POINT('Ctrl Pts',(2.00917680318424,1.,-0.15248488362145));
#48896=CARTESIAN_POINT('Ctrl Pts',(2.00335565310543,-1.,-0.154221403049722));
#48897=CARTESIAN_POINT('Ctrl Pts',(2.00335565310543,1.,-0.154221403049722));
#48898=CARTESIAN_POINT('Ctrl Pts',(1.99753284771497,-1.,-0.155904629548784));
#48899=CARTESIAN_POINT('Ctrl Pts',(1.99753284771497,1.,-0.155904629548784));
#48900=CARTESIAN_POINT('Ctrl Pts',(1.99169810931908,-1.,-0.157533331459227));
#48901=CARTESIAN_POINT('Ctrl Pts',(1.99169810931908,1.,-0.157533331459227));
#48902=CARTESIAN_POINT('Ctrl Pts',(1.98584238283292,-1.,-0.159106226437299));
#48903=CARTESIAN_POINT('Ctrl Pts',(1.98584238283292,1.,-0.159106226437299));
#48904=CARTESIAN_POINT('Ctrl Pts',(1.97996195437559,-1.,-0.160622060784611));
#48905=CARTESIAN_POINT('Ctrl Pts',(1.97996195437559,1.,-0.160622060784611));
#48906=CARTESIAN_POINT('Ctrl Pts',(1.97406280235188,-1.,-0.162079693556289));
#48907=CARTESIAN_POINT('Ctrl Pts',(1.97406280235188,1.,-0.162079693556289));
#48908=CARTESIAN_POINT('Ctrl Pts',(1.96816512677967,-1.,-0.163478185457734));
#48909=CARTESIAN_POINT('Ctrl Pts',(1.96816512677967,1.,-0.163478185457734));
#48910=CARTESIAN_POINT('Ctrl Pts',(1.96229379940136,-1.,-0.164816568920269));
#48911=CARTESIAN_POINT('Ctrl Pts',(1.96229379940136,1.,-0.164816568920269));
#48912=CARTESIAN_POINT('Ctrl Pts',(1.9564675971873,-1.,-0.166093592002813));
#48913=CARTESIAN_POINT('Ctrl Pts',(1.9564675971873,1.,-0.166093592002813));
#48914=CARTESIAN_POINT('Ctrl Pts',(1.95069027794294,-1.,-0.167307501784476));
#48915=CARTESIAN_POINT('Ctrl Pts',(1.95069027794294,1.,-0.167307501784476));
#48916=CARTESIAN_POINT('Ctrl Pts',(1.94493757756931,-1.,-0.168455741607556));
#48917=CARTESIAN_POINT('Ctrl Pts',(1.94493757756931,1.,-0.168455741607556));
#48918=CARTESIAN_POINT('Ctrl Pts',(1.93915639211581,-1.,-0.169534904817491));
#48919=CARTESIAN_POINT('Ctrl Pts',(1.93915639211581,1.,-0.169534904817491));
#48920=CARTESIAN_POINT('Ctrl Pts',(1.93329183155539,-1.,-0.170541253116202));
#48921=CARTESIAN_POINT('Ctrl Pts',(1.93329183155539,1.,-0.170541253116202));
#48922=CARTESIAN_POINT('Ctrl Pts',(1.92731093582036,-1.,-0.171471191532988));
#48923=CARTESIAN_POINT('Ctrl Pts',(1.92731093582036,1.,-0.171471191532988));
#48924=CARTESIAN_POINT('Ctrl Pts',(1.9212233439798,-1.,-0.172321621259514));
#48925=CARTESIAN_POINT('Ctrl Pts',(1.9212233439798,1.,-0.172321621259514));
#48926=CARTESIAN_POINT('Ctrl Pts',(1.91511429159527,-1.,-0.173090695383496));
#48927=CARTESIAN_POINT('Ctrl Pts',(1.91511429159527,1.,-0.173090695383496));
#48928=CARTESIAN_POINT('Ctrl Pts',(1.90911693975267,-1.,-0.173776635257817));
#48929=CARTESIAN_POINT('Ctrl Pts',(1.90911693975267,1.,-0.173776635257817));
#48930=CARTESIAN_POINT('Ctrl Pts',(1.90335253862834,-1.,-0.174375518661085));
#48931=CARTESIAN_POINT('Ctrl Pts',(1.90335253862834,1.,-0.174375518661085));
#48932=CARTESIAN_POINT('Ctrl Pts',(1.89788101117132,-1.,-0.174879405091263));
#48933=CARTESIAN_POINT('Ctrl Pts',(1.89788101117132,1.,-0.174879405091263));
#48934=CARTESIAN_POINT('Ctrl Pts',(1.892646301985,-1.,-0.175274276190844));
#48935=CARTESIAN_POINT('Ctrl Pts',(1.892646301985,1.,-0.175274276190844));
#48936=CARTESIAN_POINT('Ctrl Pts',(1.88742606273259,-1.,-0.175538155840648));
#48937=CARTESIAN_POINT('Ctrl Pts',(1.88742606273259,1.,-0.175538155840648));
#48938=CARTESIAN_POINT('Ctrl Pts',(1.88188663145367,-1.,-0.175644148889699));
#48939=CARTESIAN_POINT('Ctrl Pts',(1.88188663145367,1.,-0.175644148889699));
#48940=CARTESIAN_POINT('Ctrl Pts',(1.87563767773588,-1.,-0.175563480746485));
#48941=CARTESIAN_POINT('Ctrl Pts',(1.87563767773588,1.,-0.175563480746485));
#48942=CARTESIAN_POINT('Ctrl Pts',(1.86828349694799,-1.,-0.175268337590758));
#48943=CARTESIAN_POINT('Ctrl Pts',(1.86828349694799,1.,-0.175268337590758));
#48944=CARTESIAN_POINT('Ctrl Pts',(1.85948367088837,-1.,-0.17473525927603));
#48945=CARTESIAN_POINT('Ctrl Pts',(1.85948367088837,1.,-0.17473525927603));
#48946=CARTESIAN_POINT('Ctrl Pts',(1.8489811319852,-1.,-0.173946627587732));
#48947=CARTESIAN_POINT('Ctrl Pts',(1.8489811319852,1.,-0.173946627587732));
#48948=CARTESIAN_POINT('Ctrl Pts',(1.83658380527692,-1.,-0.1728894428919));
#48949=CARTESIAN_POINT('Ctrl Pts',(1.83658380527692,1.,-0.1728894428919));
#48950=CARTESIAN_POINT('Ctrl Pts',(1.82215766811545,-1.,-0.171554770204119));
#48951=CARTESIAN_POINT('Ctrl Pts',(1.82215766811545,1.,-0.171554770204119));
#48952=CARTESIAN_POINT('Ctrl Pts',(1.80561530629706,-1.,-0.169936923904608));
#48953=CARTESIAN_POINT('Ctrl Pts',(1.80561530629706,1.,-0.169936923904608));
#48954=CARTESIAN_POINT('Ctrl Pts',(1.7869064998507,-1.,-0.168032772805197));
#48955=CARTESIAN_POINT('Ctrl Pts',(1.7869064998507,1.,-0.168032772805197));
#48956=CARTESIAN_POINT('Ctrl Pts',(1.77018771684844,-1.,-0.1662793551464));
#48957=CARTESIAN_POINT('Ctrl Pts',(1.77018771684844,1.,-0.1662793551464));
#48958=CARTESIAN_POINT('Ctrl Pts',(1.75666056638427,-1.,-0.164834765707159));
#48959=CARTESIAN_POINT('Ctrl Pts',(1.75666056638427,1.,-0.164834765707159));
#48960=CARTESIAN_POINT('Ctrl Pts',(1.7472034950333,-1.,-0.163814161002002));
#48961=CARTESIAN_POINT('Ctrl Pts',(1.7472034950333,1.,-0.163814161002002));
#48962=CARTESIAN_POINT('Ctrl Pts',(1.74236521665491,-1.,-0.163289472382896));
#48963=CARTESIAN_POINT('Ctrl Pts',(1.74236521665491,1.,-0.163289472382896));
#48964=CARTESIAN_POINT('',(2.19890268624765,1.,-0.0694764450219582));
#48965=CARTESIAN_POINT('Ctrl Pts',(2.19890268624765,1.,-0.0694764450219582));
#48966=CARTESIAN_POINT('Ctrl Pts',(2.19777582085423,1.,-0.0701143536325491));
#48967=CARTESIAN_POINT('Ctrl Pts',(2.19552129484002,1.,-0.0713863779526155));
#48968=CARTESIAN_POINT('Ctrl Pts',(2.19213712013662,1.,-0.0732830357306726));
#48969=CARTESIAN_POINT('Ctrl Pts',(2.1876201139953,1.,-0.0757891465836149));
#48970=CARTESIAN_POINT('Ctrl Pts',(2.18196589448887,1.,-0.0788837727685244));
#48971=CARTESIAN_POINT('Ctrl Pts',(2.176303712113,1.,-0.0819402680872767));
#48972=CARTESIAN_POINT('Ctrl Pts',(2.17063357870952,1.,-0.0849584620835374));
#48973=CARTESIAN_POINT('Ctrl Pts',(2.16495552645014,1.,-0.0879381291386924));
#48974=CARTESIAN_POINT('Ctrl Pts',(2.15926961544516,1.,-0.0908789888107267));
#48975=CARTESIAN_POINT('Ctrl Pts',(2.1535759397817,1.,-0.0937807218867645));
#48976=CARTESIAN_POINT('Ctrl Pts',(2.14787463531795,1.,-0.096642985230546));
#48977=CARTESIAN_POINT('Ctrl Pts',(2.14216588396025,1.,-0.0994654261990917));
#48978=CARTESIAN_POINT('Ctrl Pts',(2.13644992667165,1.,-0.102247700556101));
#48979=CARTESIAN_POINT('Ctrl Pts',(2.13072704887293,1.,-0.10498947915274));
#48980=CARTESIAN_POINT('Ctrl Pts',(2.12499752307,1.,-0.10769043523109));
#48981=CARTESIAN_POINT('Ctrl Pts',(2.11926155590865,1.,-0.110350236135025));
#48982=CARTESIAN_POINT('Ctrl Pts',(2.11351924490306,1.,-0.112968534419737));
#48983=CARTESIAN_POINT('Ctrl Pts',(2.10777050261309,1.,-0.115544957687927));
#48984=CARTESIAN_POINT('Ctrl Pts',(2.102015121329,1.,-0.118079107988356));
#48985=CARTESIAN_POINT('Ctrl Pts',(2.0962529286773,1.,-0.120570567965122));
#48986=CARTESIAN_POINT('Ctrl Pts',(2.09048392424825,1.,-0.123018905621083));
#48987=CARTESIAN_POINT('Ctrl Pts',(2.08470840653643,1.,-0.125423679412062));
#48988=CARTESIAN_POINT('Ctrl Pts',(2.07892715110987,1.,-0.12778444527612));
#48989=CARTESIAN_POINT('Ctrl Pts',(2.07314114713063,1.,-0.130100748328404));
#48990=CARTESIAN_POINT('Ctrl Pts',(2.06735123910326,1.,-0.132372111547711));
#48991=CARTESIAN_POINT('Ctrl Pts',(2.06155781517842,1.,-0.134598026192106));
#48992=CARTESIAN_POINT('Ctrl Pts',(2.05576044414264,1.,-0.136777941218044));
#48993=CARTESIAN_POINT('Ctrl Pts',(2.04995762001328,1.,-0.138911255368966));
#48994=CARTESIAN_POINT('Ctrl Pts',(2.04414757947916,1.,-0.140997332152546));
#48995=CARTESIAN_POINT('Ctrl Pts',(2.03832911025912,1.,-0.143035515058209));
#48996=CARTESIAN_POINT('Ctrl Pts',(2.03250223739942,1.,-0.145025140186058));
#48997=CARTESIAN_POINT('Ctrl Pts',(2.02666926182017,1.,-0.146965557332583));
#48998=CARTESIAN_POINT('Ctrl Pts',(2.02083464969894,1.,-0.148856124775337));
#48999=CARTESIAN_POINT('Ctrl Pts',(2.01500291940238,1.,-0.150696157673078));
#49000=CARTESIAN_POINT('Ctrl Pts',(2.00917680318424,1.,-0.15248488362145));
#49001=CARTESIAN_POINT('Ctrl Pts',(2.00335565310543,1.,-0.154221403049722));
#49002=CARTESIAN_POINT('Ctrl Pts',(1.99753284771497,1.,-0.155904629548784));
#49003=CARTESIAN_POINT('Ctrl Pts',(1.99169810931908,1.,-0.157533331459227));
#49004=CARTESIAN_POINT('Ctrl Pts',(1.98584238283292,1.,-0.159106226437299));
#49005=CARTESIAN_POINT('Ctrl Pts',(1.97996195437559,1.,-0.160622060784611));
#49006=CARTESIAN_POINT('Ctrl Pts',(1.97406280235188,1.,-0.162079693556289));
#49007=CARTESIAN_POINT('Ctrl Pts',(1.96816512677967,1.,-0.163478185457734));
#49008=CARTESIAN_POINT('Ctrl Pts',(1.96229379940136,1.,-0.164816568920269));
#49009=CARTESIAN_POINT('Ctrl Pts',(1.9564675971873,1.,-0.166093592002813));
#49010=CARTESIAN_POINT('Ctrl Pts',(1.95069027794294,1.,-0.167307501784476));
#49011=CARTESIAN_POINT('Ctrl Pts',(1.94493757756931,1.,-0.168455741607556));
#49012=CARTESIAN_POINT('Ctrl Pts',(1.93915639211581,1.,-0.169534904817491));
#49013=CARTESIAN_POINT('Ctrl Pts',(1.93329183155539,1.,-0.170541253116202));
#49014=CARTESIAN_POINT('Ctrl Pts',(1.92731093582036,1.,-0.171471191532988));
#49015=CARTESIAN_POINT('Ctrl Pts',(1.9212233439798,1.,-0.172321621259514));
#49016=CARTESIAN_POINT('Ctrl Pts',(1.91511429159527,1.,-0.173090695383496));
#49017=CARTESIAN_POINT('Ctrl Pts',(1.90911693975267,1.,-0.173776635257817));
#49018=CARTESIAN_POINT('Ctrl Pts',(1.90335253862834,1.,-0.174375518661085));
#49019=CARTESIAN_POINT('Ctrl Pts',(1.89788101117132,1.,-0.174879405091263));
#49020=CARTESIAN_POINT('Ctrl Pts',(1.892646301985,1.,-0.175274276190844));
#49021=CARTESIAN_POINT('Ctrl Pts',(1.88742606273259,1.,-0.175538155840648));
#49022=CARTESIAN_POINT('Ctrl Pts',(1.88188663145367,1.,-0.175644148889699));
#49023=CARTESIAN_POINT('Ctrl Pts',(1.87563767773588,1.,-0.175563480746485));
#49024=CARTESIAN_POINT('Ctrl Pts',(1.86828349694799,1.,-0.175268337590758));
#49025=CARTESIAN_POINT('Ctrl Pts',(1.85948367088837,1.,-0.17473525927603));
#49026=CARTESIAN_POINT('Ctrl Pts',(1.8489811319852,1.,-0.173946627587732));
#49027=CARTESIAN_POINT('Ctrl Pts',(1.83658380527692,1.,-0.1728894428919));
#49028=CARTESIAN_POINT('Ctrl Pts',(1.82215766811545,1.,-0.171554770204119));
#49029=CARTESIAN_POINT('Ctrl Pts',(1.80561530629706,1.,-0.169936923904608));
#49030=CARTESIAN_POINT('Ctrl Pts',(1.7869064998507,1.,-0.168032772805197));
#49031=CARTESIAN_POINT('Ctrl Pts',(1.77018771684844,1.,-0.1662793551464));
#49032=CARTESIAN_POINT('Ctrl Pts',(1.75666056638427,1.,-0.164834765707159));
#49033=CARTESIAN_POINT('Ctrl Pts',(1.7472034950333,1.,-0.163814161002002));
#49034=CARTESIAN_POINT('Ctrl Pts',(1.74236521665491,1.,-0.163289472382896));
#49035=CARTESIAN_POINT('',(2.19890268624765,0.,-0.0694764450219582));
#49036=CARTESIAN_POINT('Origin',(2.19890268624765,0.,0.0694764450219582));
#49037=CARTESIAN_POINT('',(2.19890268624765,1.,0.0694764450219582));
#49038=CARTESIAN_POINT('',(2.19890268624765,1.,-0.0694764450219582));
#49039=CARTESIAN_POINT('',(2.19890268624765,0.,0.0694764450219582));
#49040=CARTESIAN_POINT('Ctrl Pts',(1.74236521665491,-1.,0.163289472382896));
#49041=CARTESIAN_POINT('Ctrl Pts',(1.74236521665491,1.,0.163289472382896));
#49042=CARTESIAN_POINT('Ctrl Pts',(1.74720349503904,-1.,0.163814161002474));
#49043=CARTESIAN_POINT('Ctrl Pts',(1.74720349503904,1.,0.163814161002474));
#49044=CARTESIAN_POINT('Ctrl Pts',(1.75666056640041,-1.,0.164834765708484));
#49045=CARTESIAN_POINT('Ctrl Pts',(1.75666056640041,1.,0.164834765708484));
#49046=CARTESIAN_POINT('Ctrl Pts',(1.77018771687692,-1.,0.166279355148738));
#49047=CARTESIAN_POINT('Ctrl Pts',(1.77018771687692,1.,0.166279355148738));
#49048=CARTESIAN_POINT('Ctrl Pts',(1.78690649988931,-1.,0.16803277280837));
#49049=CARTESIAN_POINT('Ctrl Pts',(1.78690649988931,1.,0.16803277280837));
#49050=CARTESIAN_POINT('Ctrl Pts',(1.80561530633924,-1.,0.169936923908078));
#49051=CARTESIAN_POINT('Ctrl Pts',(1.80561530633924,1.,0.169936923908078));
#49052=CARTESIAN_POINT('Ctrl Pts',(1.82215766815414,-1.,0.171554770207306));
#49053=CARTESIAN_POINT('Ctrl Pts',(1.82215766815414,1.,0.171554770207306));
#49054=CARTESIAN_POINT('Ctrl Pts',(1.83658380530747,-1.,0.17288944289442));
#49055=CARTESIAN_POINT('Ctrl Pts',(1.83658380530747,1.,0.17288944289442));
#49056=CARTESIAN_POINT('Ctrl Pts',(1.84898113200543,-1.,0.173946627589401));
#49057=CARTESIAN_POINT('Ctrl Pts',(1.84898113200543,1.,0.173946627589401));
#49058=CARTESIAN_POINT('Ctrl Pts',(1.85948367089838,-1.,0.174735259276856));
#49059=CARTESIAN_POINT('Ctrl Pts',(1.85948367089838,1.,0.174735259276856));
#49060=CARTESIAN_POINT('Ctrl Pts',(1.86828349694972,-1.,0.1752683375909));
#49061=CARTESIAN_POINT('Ctrl Pts',(1.86828349694972,1.,0.1752683375909));
#49062=CARTESIAN_POINT('Ctrl Pts',(1.87563767773249,-1.,0.175563480746205));
#49063=CARTESIAN_POINT('Ctrl Pts',(1.87563767773249,1.,0.175563480746205));
#49064=CARTESIAN_POINT('Ctrl Pts',(1.88188663144846,-1.,0.175644148889271));
#49065=CARTESIAN_POINT('Ctrl Pts',(1.88188663144846,1.,0.175644148889271));
#49066=CARTESIAN_POINT('Ctrl Pts',(1.88742606272818,-1.,0.175538155840286));
#49067=CARTESIAN_POINT('Ctrl Pts',(1.88742606272818,1.,0.175538155840286));
#49068=CARTESIAN_POINT('Ctrl Pts',(1.89264630198279,-1.,0.175274276190664));
#49069=CARTESIAN_POINT('Ctrl Pts',(1.89264630198279,1.,0.175274276190664));
#49070=CARTESIAN_POINT('Ctrl Pts',(1.89788101117148,-1.,0.174879405091277));
#49071=CARTESIAN_POINT('Ctrl Pts',(1.89788101117148,1.,0.174879405091277));
#49072=CARTESIAN_POINT('Ctrl Pts',(1.90335253863003,-1.,0.174375518661222));
#49073=CARTESIAN_POINT('Ctrl Pts',(1.90335253863003,1.,0.174375518661222));
#49074=CARTESIAN_POINT('Ctrl Pts',(1.90911693975475,-1.,0.173776635257983));
#49075=CARTESIAN_POINT('Ctrl Pts',(1.90911693975475,1.,0.173776635257983));
#49076=CARTESIAN_POINT('Ctrl Pts',(1.91511429159681,-1.,0.173090695383619));
#49077=CARTESIAN_POINT('Ctrl Pts',(1.91511429159681,1.,0.173090695383619));
#49078=CARTESIAN_POINT('Ctrl Pts',(1.92122334398034,-1.,0.172321621259556));
#49079=CARTESIAN_POINT('Ctrl Pts',(1.92122334398034,1.,0.172321621259556));
#49080=CARTESIAN_POINT('Ctrl Pts',(1.92731093582,-1.,0.17147119153296));
#49081=CARTESIAN_POINT('Ctrl Pts',(1.92731093582,1.,0.17147119153296));
#49082=CARTESIAN_POINT('Ctrl Pts',(1.93329183155455,-1.,0.170541253116136));
#49083=CARTESIAN_POINT('Ctrl Pts',(1.93329183155455,1.,0.170541253116136));
#49084=CARTESIAN_POINT('Ctrl Pts',(1.93915639211497,-1.,0.169534904817425));
#49085=CARTESIAN_POINT('Ctrl Pts',(1.93915639211497,1.,0.169534904817425));
#49086=CARTESIAN_POINT('Ctrl Pts',(1.94493757756879,-1.,0.168455741607515));
#49087=CARTESIAN_POINT('Ctrl Pts',(1.94493757756879,1.,0.168455741607515));
#49088=CARTESIAN_POINT('Ctrl Pts',(1.95069027794286,-1.,0.167307501784469));
#49089=CARTESIAN_POINT('Ctrl Pts',(1.95069027794286,1.,0.167307501784469));
#49090=CARTESIAN_POINT('Ctrl Pts',(1.95646759718755,-1.,0.166093592002832));
#49091=CARTESIAN_POINT('Ctrl Pts',(1.95646759718755,1.,0.166093592002832));
#49092=CARTESIAN_POINT('Ctrl Pts',(1.96229379940174,-1.,0.1648165689203));
#49093=CARTESIAN_POINT('Ctrl Pts',(1.96229379940174,1.,0.1648165689203));
#49094=CARTESIAN_POINT('Ctrl Pts',(1.96816512678,-1.,0.16347818545776));
#49095=CARTESIAN_POINT('Ctrl Pts',(1.96816512678,1.,0.16347818545776));
#49096=CARTESIAN_POINT('Ctrl Pts',(1.97406280235204,-1.,0.162079693556302));
#49097=CARTESIAN_POINT('Ctrl Pts',(1.97406280235204,1.,0.162079693556302));
#49098=CARTESIAN_POINT('Ctrl Pts',(1.97996195437557,-1.,0.16062206078461));
#49099=CARTESIAN_POINT('Ctrl Pts',(1.97996195437557,1.,0.16062206078461));
#49100=CARTESIAN_POINT('Ctrl Pts',(1.98584238283279,-1.,0.159106226437288));
#49101=CARTESIAN_POINT('Ctrl Pts',(1.98584238283279,1.,0.159106226437288));
#49102=CARTESIAN_POINT('Ctrl Pts',(1.99169810931893,-1.,0.157533331459215));
#49103=CARTESIAN_POINT('Ctrl Pts',(1.99169810931893,1.,0.157533331459215));
#49104=CARTESIAN_POINT('Ctrl Pts',(1.99753284771487,-1.,0.155904629548774));
#49105=CARTESIAN_POINT('Ctrl Pts',(1.99753284771487,1.,0.155904629548774));
#49106=CARTESIAN_POINT('Ctrl Pts',(2.00335565310539,-1.,0.154221403049719));
#49107=CARTESIAN_POINT('Ctrl Pts',(2.00335565310539,1.,0.154221403049719));
#49108=CARTESIAN_POINT('Ctrl Pts',(2.00917680318426,-1.,0.152484883621452));
#49109=CARTESIAN_POINT('Ctrl Pts',(2.00917680318426,1.,0.152484883621452));
#49110=CARTESIAN_POINT('Ctrl Pts',(2.01500291940243,-1.,0.150696157673084));
#49111=CARTESIAN_POINT('Ctrl Pts',(2.01500291940243,1.,0.150696157673084));
#49112=CARTESIAN_POINT('Ctrl Pts',(2.02083464969897,-1.,0.148856124775342));
#49113=CARTESIAN_POINT('Ctrl Pts',(2.02083464969897,1.,0.148856124775342));
#49114=CARTESIAN_POINT('Ctrl Pts',(2.02666926182017,-1.,0.146965557332586));
#49115=CARTESIAN_POINT('Ctrl Pts',(2.02666926182017,1.,0.146965557332586));
#49116=CARTESIAN_POINT('Ctrl Pts',(2.03250223739941,-1.,0.145025140186058));
#49117=CARTESIAN_POINT('Ctrl Pts',(2.03250223739941,1.,0.145025140186058));
#49118=CARTESIAN_POINT('Ctrl Pts',(2.03832911025913,-1.,0.143035515058208));
#49119=CARTESIAN_POINT('Ctrl Pts',(2.03832911025913,1.,0.143035515058208));
#49120=CARTESIAN_POINT('Ctrl Pts',(2.04414757947919,-1.,0.140997332152545));
#49121=CARTESIAN_POINT('Ctrl Pts',(2.04414757947919,1.,0.140997332152545));
#49122=CARTESIAN_POINT('Ctrl Pts',(2.04995762001333,-1.,0.138911255368966));
#49123=CARTESIAN_POINT('Ctrl Pts',(2.04995762001333,1.,0.138911255368966));
#49124=CARTESIAN_POINT('Ctrl Pts',(2.0557604441427,-1.,0.136777941218044));
#49125=CARTESIAN_POINT('Ctrl Pts',(2.0557604441427,1.,0.136777941218044));
#49126=CARTESIAN_POINT('Ctrl Pts',(2.06155781517844,-1.,0.134598026192107));
#49127=CARTESIAN_POINT('Ctrl Pts',(2.06155781517844,1.,0.134598026192107));
#49128=CARTESIAN_POINT('Ctrl Pts',(2.06735123910319,-1.,0.132372111547709));
#49129=CARTESIAN_POINT('Ctrl Pts',(2.06735123910319,1.,0.132372111547709));
#49130=CARTESIAN_POINT('Ctrl Pts',(2.07314114713047,-1.,0.1301007483284));
#49131=CARTESIAN_POINT('Ctrl Pts',(2.07314114713047,1.,0.1301007483284));
#49132=CARTESIAN_POINT('Ctrl Pts',(2.07892715110967,-1.,0.127784445276116));
#49133=CARTESIAN_POINT('Ctrl Pts',(2.07892715110967,1.,0.127784445276116));
#49134=CARTESIAN_POINT('Ctrl Pts',(2.08470840653628,-1.,0.125423679412058));
#49135=CARTESIAN_POINT('Ctrl Pts',(2.08470840653628,1.,0.125423679412058));
#49136=CARTESIAN_POINT('Ctrl Pts',(2.09048392424826,-1.,0.123018905621083));
#49137=CARTESIAN_POINT('Ctrl Pts',(2.09048392424826,1.,0.123018905621083));
#49138=CARTESIAN_POINT('Ctrl Pts',(2.09625292867756,-1.,0.120570567965129));
#49139=CARTESIAN_POINT('Ctrl Pts',(2.09625292867756,1.,0.120570567965129));
#49140=CARTESIAN_POINT('Ctrl Pts',(2.10201512132945,-1.,0.118079107988368));
#49141=CARTESIAN_POINT('Ctrl Pts',(2.10201512132945,1.,0.118079107988368));
#49142=CARTESIAN_POINT('Ctrl Pts',(2.10777050261359,-1.,0.11554495768794));
#49143=CARTESIAN_POINT('Ctrl Pts',(2.10777050261359,1.,0.11554495768794));
#49144=CARTESIAN_POINT('Ctrl Pts',(2.11351924490335,-1.,0.112968534419746));
#49145=CARTESIAN_POINT('Ctrl Pts',(2.11351924490335,1.,0.112968534419746));
#49146=CARTESIAN_POINT('Ctrl Pts',(2.11926155590849,-1.,0.11035023613502));
#49147=CARTESIAN_POINT('Ctrl Pts',(2.11926155590849,1.,0.11035023613502));
#49148=CARTESIAN_POINT('Ctrl Pts',(2.12499752306927,-1.,0.107690435231068));
#49149=CARTESIAN_POINT('Ctrl Pts',(2.12499752306927,1.,0.107690435231068));
#49150=CARTESIAN_POINT('Ctrl Pts',(2.1307270488718,-1.,0.104989479152703));
#49151=CARTESIAN_POINT('Ctrl Pts',(2.1307270488718,1.,0.104989479152703));
#49152=CARTESIAN_POINT('Ctrl Pts',(2.13644992667052,-1.,0.102247700556063));
#49153=CARTESIAN_POINT('Ctrl Pts',(2.13644992667052,1.,0.102247700556063));
#49154=CARTESIAN_POINT('Ctrl Pts',(2.14216588395974,-1.,0.0994654261990741));
#49155=CARTESIAN_POINT('Ctrl Pts',(2.14216588395974,1.,0.0994654261990741));
#49156=CARTESIAN_POINT('Ctrl Pts',(2.14787463531864,-1.,0.0966429852305688));
#49157=CARTESIAN_POINT('Ctrl Pts',(2.14787463531864,1.,0.0966429852305688));
#49158=CARTESIAN_POINT('Ctrl Pts',(2.15357593978377,-1.,0.0937807218868344));
#49159=CARTESIAN_POINT('Ctrl Pts',(2.15357593978377,1.,0.0937807218868344));
#49160=CARTESIAN_POINT('Ctrl Pts',(2.15926961544808,-1.,0.0908789888108265));
#49161=CARTESIAN_POINT('Ctrl Pts',(2.15926961544808,1.,0.0908789888108265));
#49162=CARTESIAN_POINT('Ctrl Pts',(2.16495552645275,-1.,0.0879381291387821));
#49163=CARTESIAN_POINT('Ctrl Pts',(2.16495552645275,1.,0.0879381291387821));
#49164=CARTESIAN_POINT('Ctrl Pts',(2.17063357871031,-1.,0.0849584620835642));
#49165=CARTESIAN_POINT('Ctrl Pts',(2.17063357871031,1.,0.0849584620835642));
#49166=CARTESIAN_POINT('Ctrl Pts',(2.1763037121106,-1.,0.0819402680871938));
#49167=CARTESIAN_POINT('Ctrl Pts',(2.1763037121106,1.,0.0819402680871938));
#49168=CARTESIAN_POINT('Ctrl Pts',(2.18196589448304,-1.,0.0788837727683226));
#49169=CARTESIAN_POINT('Ctrl Pts',(2.18196589448304,1.,0.0788837727683226));
#49170=CARTESIAN_POINT('Ctrl Pts',(2.1876201139874,-1.,0.075789146583341));
#49171=CARTESIAN_POINT('Ctrl Pts',(2.1876201139874,1.,0.075789146583341));
#49172=CARTESIAN_POINT('Ctrl Pts',(2.19213712012956,-1.,0.0732830357304275));
#49173=CARTESIAN_POINT('Ctrl Pts',(2.19213712012956,1.,0.0732830357304275));
#49174=CARTESIAN_POINT('Ctrl Pts',(2.19552129483562,-1.,0.0713863779524626));
#49175=CARTESIAN_POINT('Ctrl Pts',(2.19552129483562,1.,0.0713863779524626));
#49176=CARTESIAN_POINT('Ctrl Pts',(2.19777582085261,-1.,0.0701143536324925));
#49177=CARTESIAN_POINT('Ctrl Pts',(2.19777582085261,1.,0.0701143536324925));
#49178=CARTESIAN_POINT('Ctrl Pts',(2.19890268624765,-1.,0.0694764450219582));
#49179=CARTESIAN_POINT('Ctrl Pts',(2.19890268624765,1.,0.0694764450219582));
#49180=CARTESIAN_POINT('',(1.74236521665491,1.,0.163289472382896));
#49181=CARTESIAN_POINT('Ctrl Pts',(1.74236521665491,1.,0.163289472382896));
#49182=CARTESIAN_POINT('Ctrl Pts',(1.74720349503904,1.,0.163814161002474));
#49183=CARTESIAN_POINT('Ctrl Pts',(1.75666056640041,1.,0.164834765708484));
#49184=CARTESIAN_POINT('Ctrl Pts',(1.77018771687692,1.,0.166279355148738));
#49185=CARTESIAN_POINT('Ctrl Pts',(1.78690649988931,1.,0.16803277280837));
#49186=CARTESIAN_POINT('Ctrl Pts',(1.80561530633924,1.,0.169936923908078));
#49187=CARTESIAN_POINT('Ctrl Pts',(1.82215766815414,1.,0.171554770207306));
#49188=CARTESIAN_POINT('Ctrl Pts',(1.83658380530747,1.,0.17288944289442));
#49189=CARTESIAN_POINT('Ctrl Pts',(1.84898113200543,1.,0.173946627589401));
#49190=CARTESIAN_POINT('Ctrl Pts',(1.85948367089838,1.,0.174735259276856));
#49191=CARTESIAN_POINT('Ctrl Pts',(1.86828349694972,1.,0.1752683375909));
#49192=CARTESIAN_POINT('Ctrl Pts',(1.87563767773249,1.,0.175563480746205));
#49193=CARTESIAN_POINT('Ctrl Pts',(1.88188663144846,1.,0.175644148889271));
#49194=CARTESIAN_POINT('Ctrl Pts',(1.88742606272818,1.,0.175538155840286));
#49195=CARTESIAN_POINT('Ctrl Pts',(1.89264630198279,1.,0.175274276190664));
#49196=CARTESIAN_POINT('Ctrl Pts',(1.89788101117148,1.,0.174879405091277));
#49197=CARTESIAN_POINT('Ctrl Pts',(1.90335253863003,1.,0.174375518661222));
#49198=CARTESIAN_POINT('Ctrl Pts',(1.90911693975475,1.,0.173776635257983));
#49199=CARTESIAN_POINT('Ctrl Pts',(1.91511429159681,1.,0.173090695383619));
#49200=CARTESIAN_POINT('Ctrl Pts',(1.92122334398034,1.,0.172321621259556));
#49201=CARTESIAN_POINT('Ctrl Pts',(1.92731093582,1.,0.17147119153296));
#49202=CARTESIAN_POINT('Ctrl Pts',(1.93329183155455,1.,0.170541253116136));
#49203=CARTESIAN_POINT('Ctrl Pts',(1.93915639211497,1.,0.169534904817425));
#49204=CARTESIAN_POINT('Ctrl Pts',(1.94493757756879,1.,0.168455741607515));
#49205=CARTESIAN_POINT('Ctrl Pts',(1.95069027794286,1.,0.167307501784469));
#49206=CARTESIAN_POINT('Ctrl Pts',(1.95646759718755,1.,0.166093592002832));
#49207=CARTESIAN_POINT('Ctrl Pts',(1.96229379940174,1.,0.1648165689203));
#49208=CARTESIAN_POINT('Ctrl Pts',(1.96816512678,1.,0.16347818545776));
#49209=CARTESIAN_POINT('Ctrl Pts',(1.97406280235204,1.,0.162079693556302));
#49210=CARTESIAN_POINT('Ctrl Pts',(1.97996195437557,1.,0.16062206078461));
#49211=CARTESIAN_POINT('Ctrl Pts',(1.98584238283279,1.,0.159106226437288));
#49212=CARTESIAN_POINT('Ctrl Pts',(1.99169810931893,1.,0.157533331459215));
#49213=CARTESIAN_POINT('Ctrl Pts',(1.99753284771487,1.,0.155904629548774));
#49214=CARTESIAN_POINT('Ctrl Pts',(2.00335565310539,1.,0.154221403049719));
#49215=CARTESIAN_POINT('Ctrl Pts',(2.00917680318426,1.,0.152484883621452));
#49216=CARTESIAN_POINT('Ctrl Pts',(2.01500291940243,1.,0.150696157673084));
#49217=CARTESIAN_POINT('Ctrl Pts',(2.02083464969897,1.,0.148856124775342));
#49218=CARTESIAN_POINT('Ctrl Pts',(2.02666926182017,1.,0.146965557332586));
#49219=CARTESIAN_POINT('Ctrl Pts',(2.03250223739941,1.,0.145025140186058));
#49220=CARTESIAN_POINT('Ctrl Pts',(2.03832911025913,1.,0.143035515058208));
#49221=CARTESIAN_POINT('Ctrl Pts',(2.04414757947919,1.,0.140997332152545));
#49222=CARTESIAN_POINT('Ctrl Pts',(2.04995762001333,1.,0.138911255368966));
#49223=CARTESIAN_POINT('Ctrl Pts',(2.0557604441427,1.,0.136777941218044));
#49224=CARTESIAN_POINT('Ctrl Pts',(2.06155781517844,1.,0.134598026192107));
#49225=CARTESIAN_POINT('Ctrl Pts',(2.06735123910319,1.,0.132372111547709));
#49226=CARTESIAN_POINT('Ctrl Pts',(2.07314114713047,1.,0.1301007483284));
#49227=CARTESIAN_POINT('Ctrl Pts',(2.07892715110967,1.,0.127784445276116));
#49228=CARTESIAN_POINT('Ctrl Pts',(2.08470840653628,1.,0.125423679412058));
#49229=CARTESIAN_POINT('Ctrl Pts',(2.09048392424826,1.,0.123018905621083));
#49230=CARTESIAN_POINT('Ctrl Pts',(2.09625292867756,1.,0.120570567965129));
#49231=CARTESIAN_POINT('Ctrl Pts',(2.10201512132945,1.,0.118079107988368));
#49232=CARTESIAN_POINT('Ctrl Pts',(2.10777050261359,1.,0.11554495768794));
#49233=CARTESIAN_POINT('Ctrl Pts',(2.11351924490335,1.,0.112968534419746));
#49234=CARTESIAN_POINT('Ctrl Pts',(2.11926155590849,1.,0.11035023613502));
#49235=CARTESIAN_POINT('Ctrl Pts',(2.12499752306927,1.,0.107690435231068));
#49236=CARTESIAN_POINT('Ctrl Pts',(2.1307270488718,1.,0.104989479152703));
#49237=CARTESIAN_POINT('Ctrl Pts',(2.13644992667052,1.,0.102247700556063));
#49238=CARTESIAN_POINT('Ctrl Pts',(2.14216588395974,1.,0.0994654261990741));
#49239=CARTESIAN_POINT('Ctrl Pts',(2.14787463531864,1.,0.0966429852305688));
#49240=CARTESIAN_POINT('Ctrl Pts',(2.15357593978377,1.,0.0937807218868344));
#49241=CARTESIAN_POINT('Ctrl Pts',(2.15926961544808,1.,0.0908789888108265));
#49242=CARTESIAN_POINT('Ctrl Pts',(2.16495552645275,1.,0.0879381291387821));
#49243=CARTESIAN_POINT('Ctrl Pts',(2.17063357871031,1.,0.0849584620835642));
#49244=CARTESIAN_POINT('Ctrl Pts',(2.1763037121106,1.,0.0819402680871938));
#49245=CARTESIAN_POINT('Ctrl Pts',(2.18196589448304,1.,0.0788837727683226));
#49246=CARTESIAN_POINT('Ctrl Pts',(2.1876201139874,1.,0.075789146583341));
#49247=CARTESIAN_POINT('Ctrl Pts',(2.19213712012956,1.,0.0732830357304275));
#49248=CARTESIAN_POINT('Ctrl Pts',(2.19552129483562,1.,0.0713863779524626));
#49249=CARTESIAN_POINT('Ctrl Pts',(2.19777582085261,1.,0.0701143536324925));
#49250=CARTESIAN_POINT('Ctrl Pts',(2.19890268624765,1.,0.0694764450219582));
#49251=CARTESIAN_POINT('',(1.74236521665491,0.,0.163289472382896));
#49252=CARTESIAN_POINT('Origin',(0.,1.,0.));
#49253=CARTESIAN_POINT('Origin',(0.,1.,0.));
#49254=CARTESIAN_POINT('Origin',(0.,0.,0.));
#73290=UNCERTAINTY_MEASURE_WITH_UNIT(LENGTH_MEASURE(0.001),#73367,
'DISTANCE_ACCURACY_VALUE',
'Maximum model space distance between geometric entities at asserted c
onnectivities');
#73302=UNCERTAINTY_MEASURE_WITH_UNIT(LENGTH_MEASURE(0.001),#73367,
'DISTANCE_ACCURACY_VALUE',
'Maximum model space distance between geometric entities at asserted c
onnectivities');
#73354=(
GEOMETRIC_REPRESENTATION_CONTEXT(3)
GLOBAL_UNCERTAINTY_ASSIGNED_CONTEXT((#73290))
GLOBAL_UNIT_ASSIGNED_CONTEXT((#73367,#73369,#73370))
REPRESENTATION_CONTEXT('','3D')
);
#73366=(
GEOMETRIC_REPRESENTATION_CONTEXT(3)
GLOBAL_UNCERTAINTY_ASSIGNED_CONTEXT((#73302))
GLOBAL_UNIT_ASSIGNED_CONTEXT((#73367,#73369,#73370))
REPRESENTATION_CONTEXT('','3D')
);
#73367=(
LENGTH_UNIT()
NAMED_UNIT(*)
SI_UNIT(.CENTI.,.METRE.)
);
#73369=(
NAMED_UNIT(*)
PLANE_ANGLE_UNIT()
SI_UNIT($,.RADIAN.)
);
#73370=(
NAMED_UNIT(*)
SI_UNIT($,.STERADIAN.)
SOLID_ANGLE_UNIT()
);
#73422=SHAPE_DEFINITION_REPRESENTATION(#73555,#73658);
#73555=PRODUCT_DEFINITION_SHAPE('',$,#73722);
#73658=SHAPE_REPRESENTATION('',(#18044),#73354);
#73670=PRODUCT_DEFINITION_CONTEXT('part definition',#73861,'design');
#73722=PRODUCT_DEFINITION('Compound pinion m2 z20 b20',
'Compound pinion m2 z20 b20',#73785,#73670);
#73785=PRODUCT_DEFINITION_FORMATION('',$,#73914);
#73861=APPLICATION_CONTEXT(
'Core Data for Automotive Mechanical Design Process');
#73862=PRODUCT_CONTEXT('part definition',#73861,'mechanical');
#73914=PRODUCT('Compound pinion m2 z20 b20',
'Compound pinion m2 z20 b20','Compound pinion m2 z20 b20',(#73862));
#73968=COLOUR_RGB('Light Blue',0.38,0.62,0.78);
#73969=FILL_AREA_STYLE_COLOUR('',#73968);
#73970=FILL_AREA_STYLE('',(#73969));
#73971=SURFACE_STYLE_FILL_AREA(#73970);
#73972=SURFACE_SIDE_STYLE('',(#73971));
#73973=SURFACE_STYLE_USAGE(.BOTH.,#73972);
#73974=PRESENTATION_STYLE_ASSIGNMENT((#73973));
ENDSEC;
END-ISO-10303-21;
